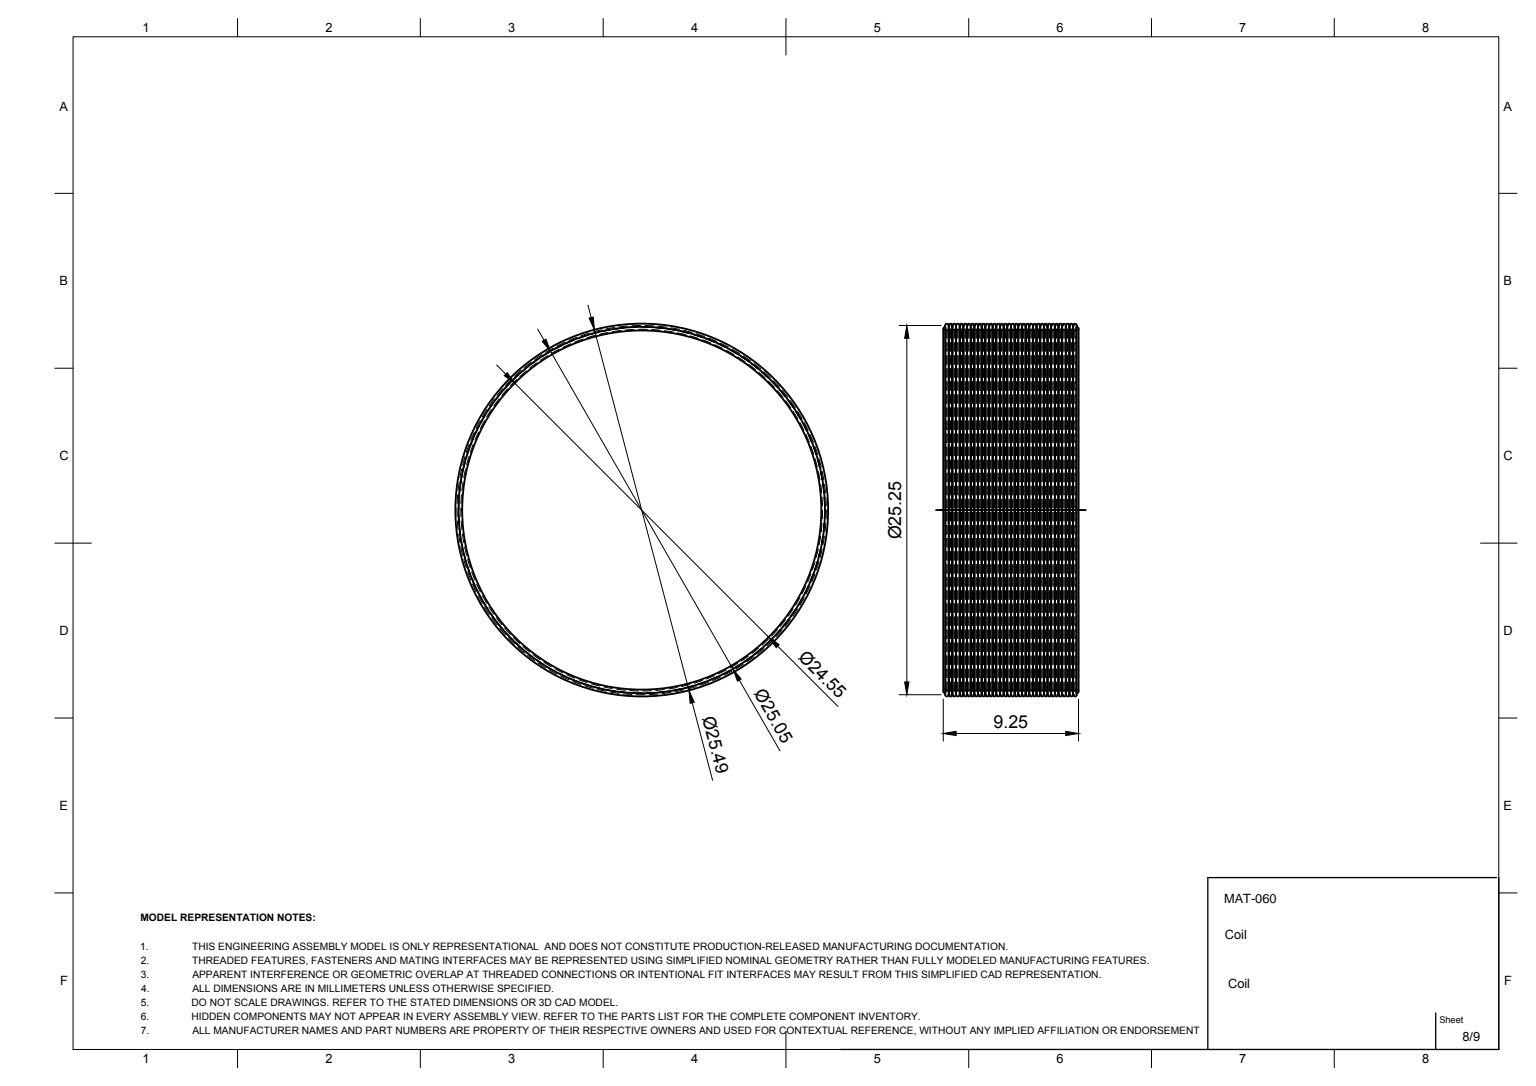
ISO-10303-21;
HEADER;
FILE_DESCRIPTION (('STEP AP214'),
    '1' );
FILE_NAME ('Coil.step',
    '2026-10-29T23:46:56',
    ( '' ),
    ( '' ),
    'SwSTEP 2.0',
    'SolidWorks 2020',
    '' );
FILE_SCHEMA (( 'AUTOMOTIVE_DESIGN' ));
ENDSEC;

DATA;
#4=CIRCLE ( 'NONE', #18333, 0.1250000000000001110 ) ;
#5=EDGE_CURVE ( 'NONE', #10473, #12904, #9508, .T. ) ;
#6=ADVANCED_FACE ( 'NONE', ( #18472 ), #27339, .T. ) ;
#8=ORIENTED_EDGE ( 'NONE', *, *, #21426, .T. ) ;
#12=DIRECTION ( 'NONE',  ( -1.000000000000000000, 0.000000000000000000, 0.000000000000000000 ) ) ;
#21=ORIENTED_EDGE ( 'NONE', *, *, #19854, .F. ) ;
#30=EDGE_CURVE ( 'NONE', #9758, #27591, #28910, .T. ) ;
#31=DIRECTION ( 'NONE',  ( -1.101824276508909887E-16, 1.000000000000000000, -0.000000000000000000 ) ) ;
#32=AXIS2_PLACEMENT_3D ( 'NONE', #27691, #3055, #609 ) ;
#39=VECTOR ( 'NONE', #4275, 1000.000000000000000 ) ;
#43=ORIENTED_EDGE ( 'NONE', *, *, #17117, .T. ) ;
#44=ORIENTED_EDGE ( 'NONE', *, *, #10247, .F. ) ;
#46=DIRECTION ( 'NONE',  ( -1.000000000000000000, 0.000000000000000000, 0.000000000000000000 ) ) ;
#49=EDGE_CURVE ( 'NONE', #29330, #16793, #26511, .T. ) ;
#50=DIRECTION ( 'NONE',  ( -1.000000000000000000, 0.000000000000000000, 0.000000000000000000 ) ) ;
#51=ADVANCED_FACE ( 'NONE', ( #19270 ), #7428, .T. ) ;
#53=DIRECTION ( 'NONE',  ( -1.000000000000000000, 0.000000000000000000, 0.000000000000000000 ) ) ;
#59=AXIS2_PLACEMENT_3D ( 'NONE', #2818, #5773, #10865 ) ;
#63=VERTEX_POINT ( 'NONE', #26669 ) ;
#64=DIRECTION ( 'NONE',  ( -1.101824276508909887E-16, 1.000000000000000000, -0.000000000000000000 ) ) ;
#73=EDGE_LOOP ( 'NONE', ( #31161, #6796, #19023, #7064 ) ) ;
#74=CARTESIAN_POINT ( 'NONE',  ( 21.09992658989238734, 38.56284415653841791, 47.04930799450051637 ) ) ;
#79=DIRECTION ( 'NONE',  ( -1.000000000000000000, 0.000000000000000000, 0.000000000000000000 ) ) ;
#80=DIRECTION ( 'NONE',  ( -1.000000000000000000, -1.101824276508909887E-16, 0.000000000000000000 ) ) ;
#81=EDGE_CURVE ( 'NONE', #21567, #17692, #8244, .T. ) ;
#84=ADVANCED_FACE ( 'NONE', ( #31282 ), #25012, .T. ) ;
#86=ORIENTED_EDGE ( 'NONE', *, *, #14796, .T. ) ;
#89=DIRECTION ( 'NONE',  ( -1.000000000000000000, 0.000000000000000000, 0.000000000000000000 ) ) ;
#92=CARTESIAN_POINT ( 'NONE',  ( 21.09992658989239089, 30.34164230456639544, 47.04930799450051637 ) ) ;
#95=ORIENTED_EDGE ( 'NONE', *, *, #26981, .T. ) ;
#97=ORIENTED_EDGE ( 'NONE', *, *, #2403, .T. ) ;
#102=DIRECTION ( 'NONE',  ( 1.000000000000000000, 0.000000000000000000, 0.000000000000000000 ) ) ;
#104=VERTEX_POINT ( 'NONE', #1886 ) ;
#107=DIRECTION ( 'NONE',  ( 1.000000000000000000, 0.000000000000000000, 0.000000000000000000 ) ) ;
#112=VERTEX_POINT ( 'NONE', #21899 ) ;
#113=CARTESIAN_POINT ( 'NONE',  ( 8.732853799281732776, 24.72145308207319303, 47.04930799450051637 ) ) ;
#116=VERTEX_POINT ( 'NONE', #3866 ) ;
#117=CARTESIAN_POINT ( 'NONE',  ( 8.732853799281729223, 24.47145308207319303, 47.04930799450051637 ) ) ;
#119=DIRECTION ( 'NONE',  ( -1.101824276508909887E-16, 1.000000000000000000, -0.000000000000000000 ) ) ;
#120=CYLINDRICAL_SURFACE ( 'NONE', #5324, 12.36707279061065101 ) ;
#121=FACE_OUTER_BOUND ( 'NONE', #7290, .T. ) ;
#124=TOROIDAL_SURFACE ( 'NONE', #25795, 12.40141737965280555, 0.1250000000000006939 ) ;
#129=ADVANCED_FACE ( 'NONE', ( #26182 ), #24211, .T. ) ;
#130=ADVANCED_FACE ( 'NONE', ( #9112 ), #21404, .F. ) ;
#131=EDGE_LOOP ( 'NONE', ( #2067, #16349, #32197, #29803 ) ) ;
#133=CARTESIAN_POINT ( 'NONE',  ( 33.72499318558949710, 28.84143805560861296, 47.04930799450051637 ) ) ;
#134=ORIENTED_EDGE ( 'NONE', *, *, #4627, .F. ) ;
#135=AXIS2_PLACEMENT_3D ( 'NONE', #30752, #22633, #17877 ) ;
#139=EDGE_LOOP ( 'NONE', ( #10436, #9194, #21125, #26055 ) ) ;
#140=CARTESIAN_POINT ( 'NONE',  ( 21.09992658989239089, 27.84164230456639544, 47.04930799450051637 ) ) ;
#141=ORIENTED_EDGE ( 'NONE', *, *, #21145, .F. ) ;
#142=CIRCLE ( 'NONE', #13264, 12.36707279061065101 ) ;
#146=EDGE_CURVE ( 'NONE', #7136, #25895, #22084, .T. ) ;
#150=FACE_OUTER_BOUND ( 'NONE', #25843, .T. ) ;
#154=VERTEX_POINT ( 'NONE', #31766 ) ;
#157=DIRECTION ( 'NONE',  ( -1.000000000000000000, 0.000000000000000000, 0.000000000000000000 ) ) ;
#172=EDGE_LOOP ( 'NONE', ( #1126, #13141, #16684, #10184 ) ) ;
#173=CARTESIAN_POINT ( 'NONE',  ( 21.09992658989239089, 24.71664230456639899, 47.04930799450051637 ) ) ;
#174=DIRECTION ( 'NONE',  ( -1.101824276508909887E-16, 1.000000000000000000, -0.000000000000000000 ) ) ;
#178=EDGE_CURVE ( 'NONE', #17205, #26283, #21557, .T. ) ;
#181=ORIENTED_EDGE ( 'NONE', *, *, #20445, .T. ) ;
#182=DIRECTION ( 'NONE',  ( -1.000000000000000000, 0.000000000000000000, 0.000000000000000000 ) ) ;
#183=ADVANCED_FACE ( 'NONE', ( #22228 ), #31147, .T. ) ;
#190=CARTESIAN_POINT ( 'NONE',  ( 21.09992658989238734, 38.56284415653841791, 47.04930799450051637 ) ) ;
#191=CARTESIAN_POINT ( 'NONE',  ( 8.698509210239514289, 24.84164230456639544, 47.04930799450051637 ) ) ;
#193=DIRECTION ( 'NONE',  ( -1.000000000000000000, 0.000000000000000000, 0.000000000000000000 ) ) ;
#200=DIRECTION ( 'NONE',  ( -1.000000000000000000, 0.000000000000000000, 0.000000000000000000 ) ) ;
#204=CARTESIAN_POINT ( 'NONE',  ( 33.46699938050303302, 38.56284415653841791, 47.04930799450051637 ) ) ;
#213=ORIENTED_EDGE ( 'NONE', *, *, #21228, .T. ) ;
#215=CARTESIAN_POINT ( 'NONE',  ( 8.732853799281732776, 31.97145308207317171, 47.04930799450051637 ) ) ;
#217=DIRECTION ( 'NONE',  ( -1.000000000000000000, 0.000000000000000000, 0.000000000000000000 ) ) ;
#219=CARTESIAN_POINT ( 'NONE',  ( 8.823509210239564027, 29.84164230456639899, 47.04930799450051637 ) ) ;
#220=ADVANCED_FACE ( 'NONE', ( #24531 ), #2050, .F. ) ;
#221=EDGE_CURVE ( 'NONE', #14341, #26283, #20036, .T. ) ;
#222=EDGE_LOOP ( 'NONE', ( #26928, #11446, #19601, #18830 ) ) ;
#223=DIRECTION ( 'NONE',  ( -1.000000000000000000, 0.000000000000000000, 0.000000000000000000 ) ) ;
#228=DIRECTION ( 'NONE',  ( -1.101824276508909887E-16, 1.000000000000000000, -0.000000000000000000 ) ) ;
#230=CARTESIAN_POINT ( 'NONE',  ( 21.09992658989238734, 31.96183152705962272, 47.04930799450051637 ) ) ;
#231=VERTEX_POINT ( 'NONE', #9774 ) ;
#236=AXIS2_PLACEMENT_3D ( 'NONE', #25222, #28009, #15050 ) ;
#237=DIRECTION ( 'NONE',  ( -1.101824276508909887E-16, 1.000000000000000000, -0.000000000000000000 ) ) ;
#246=ORIENTED_EDGE ( 'NONE', *, *, #15564, .T. ) ;
#248=DIRECTION ( 'NONE',  ( 0.000000000000000000, -0.000000000000000000, -1.000000000000000000 ) ) ;
#254=DIRECTION ( 'NONE',  ( -1.101824276508909887E-16, 1.000000000000000000, -0.000000000000000000 ) ) ;
#256=EDGE_CURVE ( 'NONE', #10661, #20619, #16974, .T. ) ;
#262=EDGE_CURVE ( 'NONE', #32275, #3483, #1780, .T. ) ;
#264=CARTESIAN_POINT ( 'NONE',  ( 8.732853799281732776, 30.71183152705961916, 47.04930799450051637 ) ) ;
#266=ORIENTED_EDGE ( 'NONE', *, *, #15415, .T. ) ;
#267=ORIENTED_EDGE ( 'NONE', *, *, #8560, .T. ) ;
#270=LINE ( 'NONE', #3046, #13238 ) ;
#272=VERTEX_POINT ( 'NONE', #8893 ) ;
#281=DIRECTION ( 'NONE',  ( -1.101824276508909887E-16, 1.000000000000000000, -0.000000000000000000 ) ) ;
#287=CARTESIAN_POINT ( 'NONE',  ( 21.09992658989239089, 24.84164230456639544, 47.04930799450051637 ) ) ;
#291=AXIS2_PLACEMENT_3D ( 'NONE', #31241, #28293, #23031 ) ;
#293=ORIENTED_EDGE ( 'NONE', *, *, #30810, .T. ) ;
#295=DIRECTION ( 'NONE',  ( -1.101824276508909887E-16, 1.000000000000000000, -0.000000000000000000 ) ) ;
#299=ADVANCED_FACE ( 'NONE', ( #6919 ), #23984, .F. ) ;
#303=EDGE_CURVE ( 'NONE', #15685, #10922, #5506, .T. ) ;
#305=CIRCLE ( 'NONE', #9213, 12.27641737965284996 ) ;
#312=CARTESIAN_POINT ( 'NONE',  ( 21.09992658989239089, 28.46183152705961206, 47.04930799450051637 ) ) ;
#314=TOROIDAL_SURFACE ( 'NONE', #1339, 12.61792373059896377, 0.1249999999999977518 ) ;
#321=VERTEX_POINT ( 'NONE', #31552 ) ;
#326=ORIENTED_EDGE ( 'NONE', *, *, #9341, .F. ) ;
#327=CARTESIAN_POINT ( 'NONE',  ( 33.72499318558949710, 27.84184655352419568, 47.04930799450051637 ) ) ;
#330=CIRCLE ( 'NONE', #8187, 12.27641737965285529 ) ;
#331=( GEOMETRIC_REPRESENTATION_CONTEXT ( 3 ) GLOBAL_UNCERTAINTY_ASSIGNED_CONTEXT ( ( #30822 ) ) GLOBAL_UNIT_ASSIGNED_CONTEXT ( ( #10061, #30087, #12694 ) ) REPRESENTATION_CONTEXT ( 'NONE', 'WORKASPACE' ) );
#333=ORIENTED_EDGE ( 'NONE', *, *, #7951, .F. ) ;
#334=ADVANCED_FACE ( 'NONE', ( #16752 ), #23450, .T. ) ;
#335=EDGE_CURVE ( 'NONE', #25296, #11753, #1955, .T. ) ;
#338=DIRECTION ( 'NONE',  ( -1.101824276508909887E-16, 1.000000000000000000, -0.000000000000000000 ) ) ;
#340=DIRECTION ( 'NONE',  ( -1.101824276508909887E-16, 1.000000000000000000, -0.000000000000000000 ) ) ;
#341=ORIENTED_EDGE ( 'NONE', *, *, #19982, .F. ) ;
#346=CARTESIAN_POINT ( 'NONE',  ( 8.698509210239533829, 26.84164230456639899, 47.04930799450051637 ) ) ;
#349=CARTESIAN_POINT ( 'NONE',  ( 21.09992658989239089, 28.46183152705961206, 47.04930799450051637 ) ) ;
#351=DIRECTION ( 'NONE',  ( 1.000000000000000000, 0.000000000000000000, 0.000000000000000000 ) ) ;
#352=DIRECTION ( 'NONE',  ( -1.000000000000000000, 0.000000000000000000, 0.000000000000000000 ) ) ;
#358=DIRECTION ( 'NONE',  ( -1.101824276508909887E-16, 1.000000000000000000, -0.000000000000000000 ) ) ;
#360=AXIS2_PLACEMENT_3D ( 'NONE', #25134, #12675, #32035 ) ;
#362=ORIENTED_EDGE ( 'NONE', *, *, #4106, .T. ) ;
#363=CARTESIAN_POINT ( 'NONE',  ( 8.732853799281732776, 31.21183152705961206, 47.04930799450051637 ) ) ;
#368=DIRECTION ( 'NONE',  ( -1.101824276508909887E-16, 1.000000000000000000, -0.000000000000000000 ) ) ;
#371=EDGE_CURVE ( 'NONE', #32203, #7136, #10883, .T. ) ;
#373=DIRECTION ( 'NONE',  ( -1.101824276508909887E-16, 1.000000000000000000, -0.000000000000000000 ) ) ;
#375=AXIS2_PLACEMENT_3D ( 'NONE', #26320, #1199, #3831 ) ;
#377=ADVANCED_FACE ( 'NONE', ( #14478 ), #21344, .F. ) ;
#381=LINE ( 'NONE', #32408, #22412 ) ;
#387=EDGE_CURVE ( 'NONE', #272, #6908, #900, .T. ) ;
#392=AXIS2_PLACEMENT_3D ( 'NONE', #10385, #24997, #12533 ) ;
#397=DIRECTION ( 'NONE',  ( -0.5849755626391566210, -0.8110509177080080789, 7.163884503654653530E-17 ) ) ;
#401=DIRECTION ( 'NONE',  ( -1.000000000000000000, -1.101824276508909764E-16, 0.000000000000000000 ) ) ;
#403=ORIENTED_EDGE ( 'NONE', *, *, #28119, .T. ) ;
#404=DIRECTION ( 'NONE',  ( -1.101824276508909887E-16, 1.000000000000000000, -0.000000000000000000 ) ) ;
#405=DIRECTION ( 'NONE',  ( -1.000000000000000000, 0.000000000000000000, 0.000000000000000000 ) ) ;
#406=ADVANCED_FACE ( 'NONE', ( #1831 ), #16107, .T. ) ;
#409=AXIS2_PLACEMENT_3D ( 'NONE', #26501, #24355, #11732 ) ;
#410=DIRECTION ( 'NONE',  ( -1.000000000000000000, 0.000000000000000000, 0.000000000000000000 ) ) ;
#412=ORIENTED_EDGE ( 'NONE', *, *, #4110, .T. ) ;
#414=VERTEX_POINT ( 'NONE', #16673 ) ;
#420=TOROIDAL_SURFACE ( 'NONE', #8282, 12.61792373059898154, 0.1249999999999967248 ) ;
#429=EDGE_CURVE ( 'NONE', #5692, #16617, #5104, .T. ) ;
#430=CARTESIAN_POINT ( 'NONE',  ( 33.50134396954523197, 28.09164230456639544, 47.04930799450051637 ) ) ;
#434=DIRECTION ( 'NONE',  ( -1.101824276508909887E-16, 1.000000000000000000, -0.000000000000000000 ) ) ;
#435=EDGE_LOOP ( 'NONE', ( #10154, #19210, #8973, #1783 ) ) ;
#442=DIRECTION ( 'NONE',  ( -1.101824276508909887E-16, 1.000000000000000000, -0.000000000000000000 ) ) ;
#443=DIRECTION ( 'NONE',  ( -1.000000000000000000, 0.000000000000000000, 0.000000000000000000 ) ) ;
#444=ORIENTED_EDGE ( 'NONE', *, *, #23203, .F. ) ;
#445=CARTESIAN_POINT ( 'NONE',  ( 21.09992658989239089, 28.09164230456639544, 47.04930799450051637 ) ) ;
#449=ADVANCED_FACE ( 'NONE', ( #28848 ), #6361, .F. ) ;
#450=AXIS2_PLACEMENT_3D ( 'NONE', #12001, #14627, #24141 ) ;
#457=DIRECTION ( 'NONE',  ( -1.101824276508909887E-16, 1.000000000000000000, -0.000000000000000000 ) ) ;
#460=VERTEX_POINT ( 'NONE', #16358 ) ;
#464=EDGE_LOOP ( 'NONE', ( #6672, #7321, #19519, #30159 ) ) ;
#465=AXIS2_PLACEMENT_3D ( 'NONE', #20669, #30697, #8207 ) ;
#473=EDGE_LOOP ( 'NONE', ( #24500, #19436, #2603, #32349 ) ) ;
#474=AXIS2_PLACEMENT_3D ( 'NONE', #27244, #4772, #14789 ) ;
#477=CARTESIAN_POINT ( 'NONE',  ( 21.09992658989239089, 25.72145308207319303, 47.04930799450051637 ) ) ;
#478=LINE ( 'NONE', #7396, #21500 ) ;
#481=DIRECTION ( 'NONE',  ( -1.101824276508909887E-16, 1.000000000000000000, -0.000000000000000000 ) ) ;
#488=AXIS2_PLACEMENT_3D ( 'NONE', #13721, #10934, #17987 ) ;
#498=CARTESIAN_POINT ( 'NONE',  ( 33.46699938050303302, 38.56284415653841791, 47.04930799450051637 ) ) ;
#505=AXIS2_PLACEMENT_3D ( 'NONE', #21570, #21893, #31922 ) ;
#511=DIRECTION ( 'NONE',  ( -1.101824276508909887E-16, 1.000000000000000000, -0.000000000000000000 ) ) ;
#515=DIRECTION ( 'NONE',  ( -1.224646799147353207E-16, -1.349345573449484691E-32, 1.000000000000000000 ) ) ;
#517=CIRCLE ( 'NONE', #11031, 0.1249999999999966416 ) ;
#518=CIRCLE ( 'NONE', #27799, 12.62506659569710266 ) ;
#519=EDGE_CURVE ( 'NONE', #12816, #17665, #21603, .T. ) ;
#520=DIRECTION ( 'NONE',  ( -1.101824276508909887E-16, 1.000000000000000000, -0.000000000000000000 ) ) ;
#521=EDGE_CURVE ( 'NONE', #13589, #18578, #21569, .T. ) ;
#523=ORIENTED_EDGE ( 'NONE', *, *, #9183, .T. ) ;
#528=ORIENTED_EDGE ( 'NONE', *, *, #976, .F. ) ;
#531=EDGE_CURVE ( 'NONE', #4270, #19118, #14239, .T. ) ;
#537=VECTOR ( 'NONE', #21856, 1000.000000000000000 ) ;
#540=CARTESIAN_POINT ( 'NONE',  ( 33.46699938050303302, 30.47145308207317882, 47.04930799450050927 ) ) ;
#542=CIRCLE ( 'NONE', #23088, 12.27641737965281266 ) ;
#543=ORIENTED_EDGE ( 'NONE', *, *, #8534, .F. ) ;
#544=CIRCLE ( 'NONE', #9998, 12.36707279061065101 ) ;
#552=ORIENTED_EDGE ( 'NONE', *, *, #8175, .T. ) ;
#554=FACE_OUTER_BOUND ( 'NONE', #4438, .T. ) ;
#555=DIRECTION ( 'NONE',  ( -1.101824276508909887E-16, 1.000000000000000000, -0.000000000000000000 ) ) ;
#556=DIRECTION ( 'NONE',  ( -1.101824276508909887E-16, 1.000000000000000000, -0.000000000000000000 ) ) ;
#562=CARTESIAN_POINT ( 'NONE',  ( 21.09992658989239089, 25.09143805560860940, 47.04930799450051637 ) ) ;
#568=EDGE_LOOP ( 'NONE', ( #14512, #13383, #25114, #14670 ) ) ;
#570=ADVANCED_FACE ( 'NONE', ( #26865 ), #5884, .T. ) ;
#573=CIRCLE ( 'NONE', #3187, 12.36707279061065101 ) ;
#574=CARTESIAN_POINT ( 'NONE',  ( 21.09992658989238734, 32.59164230456639899, 47.04930799450051637 ) ) ;
#575=ORIENTED_EDGE ( 'NONE', *, *, #29988, .T. ) ;
#576=CARTESIAN_POINT ( 'NONE',  ( 8.823509210239508960, 24.34164230456639544, 47.04930799450051637 ) ) ;
#578=CIRCLE ( 'NONE', #23109, 12.62506659569710266 ) ;
#579=EDGE_LOOP ( 'NONE', ( #28790, #1429, #13483, #28688 ) ) ;
#580=CIRCLE ( 'NONE', #21523, 12.27641737965287660 ) ;
#582=ORIENTED_EDGE ( 'NONE', *, *, #11719, .F. ) ;
#583=EDGE_CURVE ( 'NONE', #20144, #2267, #11926, .T. ) ;
#590=EDGE_CURVE ( 'NONE', #21064, #20430, #26831, .T. ) ;
#593=VERTEX_POINT ( 'NONE', #10739 ) ;
#597=FACE_OUTER_BOUND ( 'NONE', #26506, .T. ) ;
#599=DIRECTION ( 'NONE',  ( -1.101824276508909887E-16, 1.000000000000000000, -0.000000000000000000 ) ) ;
#602=CARTESIAN_POINT ( 'NONE',  ( 21.09992658989238734, 32.34143805560860585, 47.04930799450051637 ) ) ;
#609=DIRECTION ( 'NONE',  ( -1.000000000000000000, 0.000000000000000000, 0.000000000000000000 ) ) ;
#611=CARTESIAN_POINT ( 'NONE',  ( 21.09992658989238734, 31.34164230456639544, 47.04930799450051637 ) ) ;
#618=DIRECTION ( 'NONE',  ( 0.000000000000000000, -0.000000000000000000, -1.000000000000000000 ) ) ;
#623=ORIENTED_EDGE ( 'NONE', *, *, #14827, .F. ) ;
#625=ADVANCED_FACE ( 'NONE', ( #9634 ), #30756, .F. ) ;
#628=DIRECTION ( 'NONE',  ( -1.101824276508909887E-16, 1.000000000000000000, -0.000000000000000000 ) ) ;
#630=ADVANCED_FACE ( 'NONE', ( #2411 ), #30939, .T. ) ;
#633=AXIS2_PLACEMENT_3D ( 'NONE', #24321, #29422, #19555 ) ;
#635=CARTESIAN_POINT ( 'NONE',  ( 33.50134396954526750, 24.84164230456639544, 47.04930799450051637 ) ) ;
#641=ORIENTED_EDGE ( 'NONE', *, *, #13247, .T. ) ;
#642=CIRCLE ( 'NONE', #30013, 12.36707279061065101 ) ;
#643=DIRECTION ( 'NONE',  ( 1.000000000000000000, 0.000000000000000000, 0.000000000000000000 ) ) ;
#645=DIRECTION ( 'NONE',  ( -1.000000000000000000, -1.101824276508910010E-16, 0.000000000000000000 ) ) ;
#648=DIRECTION ( 'NONE',  ( 1.101824276508909887E-16, -1.000000000000000000, 0.000000000000000000 ) ) ;
#650=DIRECTION ( 'NONE',  ( 1.000000000000000000, 0.000000000000000000, 0.000000000000000000 ) ) ;
#657=CARTESIAN_POINT ( 'NONE',  ( 21.09992658989238734, 38.56284415653841791, 47.04930799450051637 ) ) ;
#658=DIRECTION ( 'NONE',  ( 0.000000000000000000, -0.000000000000000000, -1.000000000000000000 ) ) ;
#661=AXIS2_PLACEMENT_3D ( 'NONE', #13637, #15449, #25779 ) ;
#662=AXIS2_PLACEMENT_3D ( 'NONE', #7675, #4884, #7833 ) ;
#667=DIRECTION ( 'NONE',  ( -1.101824276508909887E-16, 1.000000000000000000, -0.000000000000000000 ) ) ;
#671=EDGE_CURVE ( 'NONE', #28587, #29229, #2630, .T. ) ;
#672=ADVANCED_FACE ( 'NONE', ( #28602 ), #22535, .T. ) ;
#679=DIRECTION ( 'NONE',  ( -1.101824276508909887E-16, 1.000000000000000000, -0.000000000000000000 ) ) ;
#680=CARTESIAN_POINT ( 'NONE',  ( 33.62634396954528171, 23.59164230456639544, 47.04930799450050927 ) ) ;
#682=CIRCLE ( 'NONE', #19008, 12.62506659569710266 ) ;
#687=ORIENTED_EDGE ( 'NONE', *, *, #2527, .F. ) ;
#689=FACE_OUTER_BOUND ( 'NONE', #3946, .T. ) ;
#693=DIRECTION ( 'NONE',  ( -1.224646799147353207E-16, -1.349345573449484691E-32, 1.000000000000000000 ) ) ;
#694=CARTESIAN_POINT ( 'NONE',  ( 8.823509210239512512, 24.59164230456639544, 47.04930799450051637 ) ) ;
#695=EDGE_LOOP ( 'NONE', ( #23280, #30142, #10297, #134 ) ) ;
#696=EDGE_LOOP ( 'NONE', ( #17955, #23554, #928, #3207 ) ) ;
#702=TOROIDAL_SURFACE ( 'NONE', #15402, 12.40141737965284108, 0.1249999999999997918 ) ;
#703=VECTOR ( 'NONE', #2894, 1000.000000000000000 ) ;
#704=DIRECTION ( 'NONE',  ( -1.000000000000000000, 0.000000000000000000, 0.000000000000000000 ) ) ;
#705=APPLICATION_CONTEXT ( 'automotive_design' ) ;
#708=ORIENTED_EDGE ( 'NONE', *, *, #2194, .T. ) ;
#711=EDGE_CURVE ( 'NONE', #20645, #17250, #26734, .T. ) ;
#713=AXIS2_PLACEMENT_3D ( 'NONE', #13100, #30498, #10310 ) ;
#714=EDGE_CURVE ( 'NONE', #24189, #27727, #5769, .T. ) ;
#717=ADVANCED_FACE ( 'NONE', ( #868 ), #14154, .T. ) ;
#729=DIRECTION ( 'NONE',  ( -1.000000000000000000, 0.000000000000000000, 0.000000000000000000 ) ) ;
#735=ORIENTED_EDGE ( 'NONE', *, *, #14856, .T. ) ;
#736=CARTESIAN_POINT ( 'NONE',  ( 21.09992658989239089, 26.59184655352419568, 47.04930799450051637 ) ) ;
#740=VECTOR ( 'NONE', #4684, 1000.000000000000000 ) ;
#741=ORIENTED_EDGE ( 'NONE', *, *, #31620, .T. ) ;
#744=EDGE_CURVE ( 'NONE', #30931, #20832, #4, .T. ) ;
#748=DIRECTION ( 'NONE',  ( -1.101824276508909887E-16, 1.000000000000000000, -0.000000000000000000 ) ) ;
#749=CARTESIAN_POINT ( 'NONE',  ( 33.46699938050304013, 25.21183152705960140, 47.04930799450051637 ) ) ;
#750=CIRCLE ( 'NONE', #26968, 0.1250000000000001110 ) ;
#757=CIRCLE ( 'NONE', #4954, 0.1250000000000001110 ) ;
#763=DIRECTION ( 'NONE',  ( -1.101824276508909887E-16, 1.000000000000000000, -0.000000000000000000 ) ) ;
#766=CARTESIAN_POINT ( 'NONE',  ( 21.09992658989238734, 38.56284415653841791, 47.04930799450051637 ) ) ;
#767=ORIENTED_EDGE ( 'NONE', *, *, #12081, .F. ) ;
#770=DIRECTION ( 'NONE',  ( -1.000000000000000000, -1.101824276508909887E-16, 0.000000000000000000 ) ) ;
#778=AXIS2_PLACEMENT_3D ( 'NONE', #28726, #16083, #11486 ) ;
#781=AXIS2_PLACEMENT_3D ( 'NONE', #5119, #12351, #22344 ) ;
#785=CIRCLE ( 'NONE', #19101, 12.62506659569710266 ) ;
#788=CARTESIAN_POINT ( 'NONE',  ( 8.732853799281738105, 29.21183152705961206, 47.04930799450051637 ) ) ;
#790=EDGE_LOOP ( 'NONE', ( #28035, #4033, #21933, #28843 ) ) ;
#792=CARTESIAN_POINT ( 'NONE',  ( 21.09992658989238734, 30.96183152705961206, 47.04930799450051637 ) ) ;
#797=ORIENTED_EDGE ( 'NONE', *, *, #29579, .T. ) ;
#798=ORIENTED_EDGE ( 'NONE', *, *, #992, .F. ) ;
#800=CARTESIAN_POINT ( 'NONE',  ( 21.09992658989239089, 28.34164230456639544, 47.04930799450051637 ) ) ;
#807=CARTESIAN_POINT ( 'NONE',  ( 33.46699938050304013, 27.47145308207318593, 47.04930799450050927 ) ) ;
#810=ORIENTED_EDGE ( 'NONE', *, *, #8618, .F. ) ;
#812=CARTESIAN_POINT ( 'NONE',  ( 21.09992658989238734, 31.09164230456639544, 47.04930799450051637 ) ) ;
#835=ORIENTED_EDGE ( 'NONE', *, *, #12736, .T. ) ;
#844=ORIENTED_EDGE ( 'NONE', *, *, #2452, .T. ) ;
#850=ORIENTED_EDGE ( 'NONE', *, *, #29495, .F. ) ;
#853=ORIENTED_EDGE ( 'NONE', *, *, #19976, .F. ) ;
#858=CIRCLE ( 'NONE', #22872, 12.62506659569710266 ) ;
#860=EDGE_CURVE ( 'NONE', #13790, #27623, #578, .T. ) ;
#863=CIRCLE ( 'NONE', #13468, 0.1250000000000001110 ) ;
#865=ORIENTED_EDGE ( 'NONE', *, *, #20443, .F. ) ;
#867=FACE_OUTER_BOUND ( 'NONE', #19263, .T. ) ;
#868=FACE_OUTER_BOUND ( 'NONE', #17054, .T. ) ;
#869=AXIS2_PLACEMENT_3D ( 'NONE', #29737, #14966, #29905 ) ;
#881=ORIENTED_EDGE ( 'NONE', *, *, #31352, .F. ) ;
#888=CIRCLE ( 'NONE', #30776, 12.27641737965288726 ) ;
#889=DIRECTION ( 'NONE',  ( -1.000000000000000000, 0.000000000000000000, 0.000000000000000000 ) ) ;
#893=VERTEX_POINT ( 'NONE', #12685 ) ;
#894=EDGE_CURVE ( 'NONE', #7034, #9970, #12106, .T. ) ;
#900=CIRCLE ( 'NONE', #31833, 12.62506659569710266 ) ;
#903=CARTESIAN_POINT ( 'NONE',  ( 8.573509210239501854, 23.59164230456639544, 47.04930799450051637 ) ) ;
#905=ORIENTED_EDGE ( 'NONE', *, *, #16478, .F. ) ;
#906=LINE ( 'NONE', #10621, #25046 ) ;
#910=DIRECTION ( 'NONE',  ( -1.000000000000000000, -1.101824276508909764E-16, 0.000000000000000000 ) ) ;
#913=EDGE_CURVE ( 'NONE', #25724, #15900, #27600, .T. ) ;
#914=ORIENTED_EDGE ( 'NONE', *, *, #23784, .T. ) ;
#917=CARTESIAN_POINT ( 'NONE',  ( 33.50134396954528171, 23.84164230456639544, 47.04930799450051637 ) ) ;
#918=DIRECTION ( 'NONE',  ( -1.000000000000000000, 0.000000000000000000, 0.000000000000000000 ) ) ;
#922=CARTESIAN_POINT ( 'NONE',  ( 21.09992658989239089, 28.46664230456639899, 47.04930799450051637 ) ) ;
#924=CARTESIAN_POINT ( 'NONE',  ( 33.37634396954526750, 25.09164230456639899, 47.04930799450051637 ) ) ;
#926=DIRECTION ( 'NONE',  ( -1.101824276508909887E-16, 1.000000000000000000, -0.000000000000000000 ) ) ;
#928=ORIENTED_EDGE ( 'NONE', *, *, #23814, .T. ) ;
#929=CARTESIAN_POINT ( 'NONE',  ( 33.46699938050304013, 28.72145308207318237, 47.04930799450050927 ) ) ;
#934=ORIENTED_EDGE ( 'NONE', *, *, #16622, .F. ) ;
#940=ORIENTED_EDGE ( 'NONE', *, *, #29043, .F. ) ;
#941=CIRCLE ( 'NONE', #31356, 12.62506659569710266 ) ;
#942=AXIS2_PLACEMENT_3D ( 'NONE', #17620, #12882, #24854 ) ;
#947=DIRECTION ( 'NONE',  ( -1.101824276508909887E-16, 1.000000000000000000, -0.000000000000000000 ) ) ;
#950=ADVANCED_FACE ( 'NONE', ( #2490 ), #25622, .F. ) ;
#951=ORIENTED_EDGE ( 'NONE', *, *, #18687, .F. ) ;
#955=EDGE_CURVE ( 'NONE', #13402, #21770, #9293, .T. ) ;
#963=AXIS2_PLACEMENT_3D ( 'NONE', #7486, #14707, #4524 ) ;
#965=CARTESIAN_POINT ( 'NONE',  ( 33.50134396954524618, 26.59164230456639899, 47.04930799450051637 ) ) ;
#968=CARTESIAN_POINT ( 'NONE',  ( 21.09992658989239089, 26.59164230456639899, 47.04930799450051637 ) ) ;
#976=EDGE_CURVE ( 'NONE', #27344, #24538, #26061, .T. ) ;
#979=VECTOR ( 'NONE', #254, 1000.000000000000000 ) ;
#984=CARTESIAN_POINT ( 'NONE',  ( 21.09992658989239089, 25.34184655352419213, 47.04930799450051637 ) ) ;
#987=AXIS2_PLACEMENT_3D ( 'NONE', #4935, #14949, #9537 ) ;
#992=EDGE_CURVE ( 'NONE', #10697, #9081, #30273, .T. ) ;
#995=ADVANCED_FACE ( 'NONE', ( #18386 ), #31829, .T. ) ;
#997=DIRECTION ( 'NONE',  ( -1.101824276508909887E-16, 1.000000000000000000, -0.000000000000000000 ) ) ;
#1000=DIRECTION ( 'NONE',  ( -1.101824276508909887E-16, 1.000000000000000000, -0.000000000000000000 ) ) ;
#1001=CARTESIAN_POINT ( 'NONE',  ( 8.732853799281734553, 38.56284415653841791, 47.04930799450051637 ) ) ;
#1002=FACE_OUTER_BOUND ( 'NONE', #23225, .T. ) ;
#1003=ORIENTED_EDGE ( 'NONE', *, *, #7201, .T. ) ;
#1004=ORIENTED_EDGE ( 'NONE', *, *, #5227, .F. ) ;
#1006=TOROIDAL_SURFACE ( 'NONE', #23517, 12.40141737965281088, 0.1249999999999987788 ) ;
#1019=AXIS2_PLACEMENT_3D ( 'NONE', #16547, #14431, #19660 ) ;
#1020=ORIENTED_EDGE ( 'NONE', *, *, #10985, .T. ) ;
#1024=TOROIDAL_SURFACE ( 'NONE', #17777, 12.61792373059896732, 0.1249999999999974604 ) ;
#1027=VERTEX_POINT ( 'NONE', #26268 ) ;
#1030=DIRECTION ( 'NONE',  ( -1.000000000000000000, 0.000000000000000000, 0.000000000000000000 ) ) ;
#1031=EDGE_CURVE ( 'NONE', #23957, #25242, #18699, .T. ) ;
#1032=AXIS2_PLACEMENT_3D ( 'NONE', #27247, #9702, #19534 ) ;
#1033=ORIENTED_EDGE ( 'NONE', *, *, #20379, .T. ) ;
#1034=VECTOR ( 'NONE', #9749, 1000.000000000000000 ) ;
#1035=DIRECTION ( 'NONE',  ( -1.101824276508909887E-16, 1.000000000000000000, -0.000000000000000000 ) ) ;
#1037=DIRECTION ( 'NONE',  ( -1.101824276508909887E-16, 1.000000000000000000, -0.000000000000000000 ) ) ;
#1039=AXIS2_PLACEMENT_3D ( 'NONE', #6070, #23305, #5912 ) ;
#1044=DIRECTION ( 'NONE',  ( 1.000000000000000000, 0.000000000000000000, 0.000000000000000000 ) ) ;
#1054=DIRECTION ( 'NONE',  ( -1.101824276508909887E-16, 1.000000000000000000, -0.000000000000000000 ) ) ;
#1055=TOROIDAL_SURFACE ( 'NONE', #17283, 12.40141737965287838, 0.1249999999999998335 ) ;
#1058=ORIENTED_EDGE ( 'NONE', *, *, #4110, .F. ) ;
#1061=CIRCLE ( 'NONE', #21472, 0.1250000000000001110 ) ;
#1062=ORIENTED_EDGE ( 'NONE', *, *, #8099, .F. ) ;
#1064=VECTOR ( 'NONE', #6334, 1000.000000000000000 ) ;
#1068=DIRECTION ( 'NONE',  ( -1.000000000000000000, 0.000000000000000000, 0.000000000000000000 ) ) ;
#1073=VERTEX_POINT ( 'NONE', #6245 ) ;
#1075=FACE_OUTER_BOUND ( 'NONE', #20162, .T. ) ;
#1076=DIRECTION ( 'NONE',  ( -1.101824276508909887E-16, 1.000000000000000000, -0.000000000000000000 ) ) ;
#1084=DIRECTION ( 'NONE',  ( -1.224646799147353207E-16, -1.349345573449484691E-32, 1.000000000000000000 ) ) ;
#1100=ORIENTED_EDGE ( 'NONE', *, *, #7352, .F. ) ;
#1107=ADVANCED_FACE ( 'NONE', ( #13328 ), #31202, .T. ) ;
#1108=EDGE_CURVE ( 'NONE', #22169, #9593, #15435, .T. ) ;
#1112=CARTESIAN_POINT ( 'NONE',  ( 21.09992658989239089, 25.84164230456639899, 47.04930799450051637 ) ) ;
#1114=EDGE_CURVE ( 'NONE', #116, #23509, #31166, .T. ) ;
#1121=VERTEX_POINT ( 'NONE', #10860 ) ;
#1126=ORIENTED_EDGE ( 'NONE', *, *, #29812, .T. ) ;
#1127=DIRECTION ( 'NONE',  ( -1.101824276508909887E-16, 1.000000000000000000, -0.000000000000000000 ) ) ;
#1128=AXIS2_PLACEMENT_3D ( 'NONE', #27328, #4847, #17796 ) ;
#1129=FACE_OUTER_BOUND ( 'NONE', #695, .T. ) ;
#1133=ORIENTED_EDGE ( 'NONE', *, *, #146, .T. ) ;
#1134=DIRECTION ( 'NONE',  ( -1.101824276508909887E-16, 1.000000000000000000, -0.000000000000000000 ) ) ;
#1136=CARTESIAN_POINT ( 'NONE',  ( 33.46699938050303302, 38.56284415653841791, 47.04930799450051637 ) ) ;
#1140=VERTEX_POINT ( 'NONE', #29378 ) ;
#1143=CARTESIAN_POINT ( 'NONE',  ( 33.50134396954523908, 27.09164230456639899, 47.04930799450051637 ) ) ;
#1144=ORIENTED_EDGE ( 'NONE', *, *, #5166, .F. ) ;
#1148=CARTESIAN_POINT ( 'NONE',  ( 21.09992658989239089, 26.59143805560860940, 47.04930799450051637 ) ) ;
#1153=DIRECTION ( 'NONE',  ( -1.101824276508909887E-16, 1.000000000000000000, -0.000000000000000000 ) ) ;
#1154=DIRECTION ( 'NONE',  ( -1.000000000000000000, 0.000000000000000000, 0.000000000000000000 ) ) ;
#1161=FACE_OUTER_BOUND ( 'NONE', #5845, .T. ) ;
#1162=TOROIDAL_SURFACE ( 'NONE', #11675, 12.40141737965283042, 0.1249999999999995420 ) ;
#1164=LINE ( 'NONE', #18085, #25026 ) ;
#1171=ADVANCED_FACE ( 'NONE', ( #12149 ), #27233, .F. ) ;
#1177=DIRECTION ( 'NONE',  ( -1.101824276508909887E-16, 1.000000000000000000, -0.000000000000000000 ) ) ;
#1183=AXIS2_PLACEMENT_3D ( 'NONE', #22137, #14606, #32166 ) ;
#1186=DIRECTION ( 'NONE',  ( -1.000000000000000000, 0.000000000000000000, 0.000000000000000000 ) ) ;
#1190=CARTESIAN_POINT ( 'NONE',  ( 21.09992658989238734, 31.34184655352422766, 47.04930799450051637 ) ) ;
#1199=DIRECTION ( 'NONE',  ( 0.000000000000000000, -0.000000000000000000, -1.000000000000000000 ) ) ;
#1205=DIRECTION ( 'NONE',  ( 1.000000000000000000, 0.000000000000000000, 0.000000000000000000 ) ) ;
#1207=EDGE_CURVE ( 'NONE', #14676, #24757, #29053, .T. ) ;
#1209=TOROIDAL_SURFACE ( 'NONE', #13804, 12.61792373059897621, 0.1249999999999970163 ) ;
#1214=EDGE_CURVE ( 'NONE', #30342, #31925, #15331, .T. ) ;
#1221=DIRECTION ( 'NONE',  ( -1.101824276508909887E-16, 1.000000000000000000, -0.000000000000000000 ) ) ;
#1228=DIRECTION ( 'NONE',  ( -1.000000000000000000, 0.000000000000000000, 0.000000000000000000 ) ) ;
#1229=VERTEX_POINT ( 'NONE', #17703 ) ;
#1232=DIRECTION ( 'NONE',  ( 1.000000000000000000, 0.000000000000000000, 0.000000000000000000 ) ) ;
#1233=DIRECTION ( 'NONE',  ( -1.000000000000000000, 0.000000000000000000, 0.000000000000000000 ) ) ;
#1241=AXIS2_PLACEMENT_3D ( 'NONE', #4451, #6592, #13985 ) ;
#1247=DIRECTION ( 'NONE',  ( -1.101824276508909887E-16, 1.000000000000000000, -0.000000000000000000 ) ) ;
#1249=ORIENTED_EDGE ( 'NONE', *, *, #26072, .T. ) ;
#1250=ORIENTED_EDGE ( 'NONE', *, *, #9597, .F. ) ;
#1253=ADVANCED_FACE ( 'NONE', ( #12805 ), #10093, .T. ) ;
#1254=ORIENTED_EDGE ( 'NONE', *, *, #21788, .F. ) ;
#1258=ORIENTED_EDGE ( 'NONE', *, *, #11197, .F. ) ;
#1264=EDGE_LOOP ( 'NONE', ( #23405, #5716, #4879, #844 ) ) ;
#1266=DIRECTION ( 'NONE',  ( -1.224646799147353207E-16, -1.349345573449484691E-32, 1.000000000000000000 ) ) ;
#1267=ORIENTED_EDGE ( 'NONE', *, *, #2115, .T. ) ;
#1269=CARTESIAN_POINT ( 'NONE',  ( 21.09992658989239089, 24.96183152705960140, 47.04930799450051637 ) ) ;
#1272=AXIS2_PLACEMENT_3D ( 'NONE', #3616, #28729, #21163 ) ;
#1274=DIRECTION ( 'NONE',  ( -1.000000000000000000, 0.000000000000000000, 0.000000000000000000 ) ) ;
#1277=ORIENTED_EDGE ( 'NONE', *, *, #711, .T. ) ;
#1280=CIRCLE ( 'NONE', #5493, 0.1250000000000001110 ) ;
#1282=AXIS2_PLACEMENT_3D ( 'NONE', #25712, #30968, #2899 ) ;
#1284=DIRECTION ( 'NONE',  ( -1.101824276508909887E-16, 1.000000000000000000, -0.000000000000000000 ) ) ;
#1287=DIRECTION ( 'NONE',  ( -1.000000000000000000, 0.000000000000000000, 0.000000000000000000 ) ) ;
#1294=EDGE_CURVE ( 'NONE', #19345, #18749, #642, .T. ) ;
#1297=TOROIDAL_SURFACE ( 'NONE', #778, 12.40141737965288904, 0.1249999999999998612 ) ;
#1304=DIRECTION ( 'NONE',  ( -1.224646799147353207E-16, -1.349345573449484691E-32, 1.000000000000000000 ) ) ;
#1306=VECTOR ( 'NONE', #4417, 1000.000000000000000 ) ;
#1307=ORIENTED_EDGE ( 'NONE', *, *, #13757, .F. ) ;
#1311=VERTEX_POINT ( 'NONE', #2458 ) ;
#1314=CYLINDRICAL_SURFACE ( 'NONE', #9732, 12.36707279061065279 ) ;
#1319=VERTEX_POINT ( 'NONE', #12964 ) ;
#1320=EDGE_CURVE ( 'NONE', #31644, #4648, #25806, .T. ) ;
#1323=FACE_OUTER_BOUND ( 'NONE', #17617, .T. ) ;
#1324=AXIS2_PLACEMENT_3D ( 'NONE', #22136, #32165, #7208 ) ;
#1325=ORIENTED_EDGE ( 'NONE', *, *, #1420, .F. ) ;
#1330=TOROIDAL_SURFACE ( 'NONE', #4473, 12.40141737965281621, 0.1250000000000009159 ) ;
#1334=FACE_OUTER_BOUND ( 'NONE', #579, .T. ) ;
#1335=AXIS2_PLACEMENT_3D ( 'NONE', #21891, #19595, #19435 ) ;
#1337=ADVANCED_FACE ( 'NONE', ( #7876 ), #23185, .T. ) ;
#1338=EDGE_CURVE ( 'NONE', #15696, #1073, #15847, .T. ) ;
#1339=AXIS2_PLACEMENT_3D ( 'NONE', #28718, #16558, #6237 ) ;
#1343=DIRECTION ( 'NONE',  ( 1.000000000000000000, 0.000000000000000000, 0.000000000000000000 ) ) ;
#1347=DIRECTION ( 'NONE',  ( -1.000000000000000000, -1.101824276508910010E-16, 0.000000000000000000 ) ) ;
#1348=CIRCLE ( 'NONE', #5561, 12.36707279061065101 ) ;
#1354=DIRECTION ( 'NONE',  ( 0.000000000000000000, 0.000000000000000000, 1.000000000000000000 ) ) ;
#1355=ORIENTED_EDGE ( 'NONE', *, *, #7152, .T. ) ;
#1360=DIRECTION ( 'NONE',  ( -1.000000000000000000, -1.101824276508909887E-16, 0.000000000000000000 ) ) ;
#1361=DIRECTION ( 'NONE',  ( -1.000000000000000000, 0.000000000000000000, 0.000000000000000000 ) ) ;
#1364=ORIENTED_EDGE ( 'NONE', *, *, #21443, .T. ) ;
#1369=CARTESIAN_POINT ( 'NONE',  ( 8.474859994195282908, 38.56284415653841791, 47.04930799450051637 ) ) ;
#1375=VERTEX_POINT ( 'NONE', #25582 ) ;
#1378=ORIENTED_EDGE ( 'NONE', *, *, #31391, .F. ) ;
#1381=ADVANCED_FACE ( 'NONE', ( #30196 ), #7984, .T. ) ;
#1383=DIRECTION ( 'NONE',  ( -1.101824276508909887E-16, 1.000000000000000000, -0.000000000000000000 ) ) ;
#1384=DIRECTION ( 'NONE',  ( -1.000000000000000000, 0.000000000000000000, 0.000000000000000000 ) ) ;
#1385=EDGE_CURVE ( 'NONE', #10661, #15368, #9022, .T. ) ;
#1391=LINE ( 'NONE', #21247, #8965 ) ;
#1392=VERTEX_POINT ( 'NONE', #20817 ) ;
#1395=DIRECTION ( 'NONE',  ( -1.101824276508909887E-16, 1.000000000000000000, -0.000000000000000000 ) ) ;
#1397=AXIS2_PLACEMENT_3D ( 'NONE', #3502, #11227, #21372 ) ;
#1400=VERTEX_POINT ( 'NONE', #11298 ) ;
#1405=EDGE_CURVE ( 'NONE', #14676, #10661, #3261, .T. ) ;
#1406=DIRECTION ( 'NONE',  ( 0.000000000000000000, -0.000000000000000000, -1.000000000000000000 ) ) ;
#1407=ORIENTED_EDGE ( 'NONE', *, *, #7950, .F. ) ;
#1410=ORIENTED_EDGE ( 'NONE', *, *, #5755, .F. ) ;
#1412=AXIS2_PLACEMENT_3D ( 'NONE', #13319, #28407, #7736 ) ;
#1413=FACE_OUTER_BOUND ( 'NONE', #29852, .T. ) ;
#1414=ORIENTED_EDGE ( 'NONE', *, *, #955, .T. ) ;
#1418=AXIS2_PLACEMENT_3D ( 'NONE', #22607, #24582, #5059 ) ;
#1420=EDGE_CURVE ( 'NONE', #20658, #19118, #20031, .T. ) ;
#1421=DIRECTION ( 'NONE',  ( -1.000000000000000000, 0.000000000000000000, 0.000000000000000000 ) ) ;
#1423=ORIENTED_EDGE ( 'NONE', *, *, #26261, .F. ) ;
#1429=ORIENTED_EDGE ( 'NONE', *, *, #23635, .F. ) ;
#1438=ADVANCED_FACE ( 'NONE', ( #28215 ), #22118, .T. ) ;
#1448=DIRECTION ( 'NONE',  ( -1.101824276508909887E-16, 1.000000000000000000, -0.000000000000000000 ) ) ;
#1451=TOROIDAL_SURFACE ( 'NONE', #31866, 12.40141737965288904, 0.1249999999999998612 ) ;
#1459=CARTESIAN_POINT ( 'NONE',  ( 33.72499318558949710, 31.59184655352418503, 47.04930799450051637 ) ) ;
#1463=EDGE_LOOP ( 'NONE', ( #32458, #3921, #4900, #4428 ) ) ;
#1465=TOROIDAL_SURFACE ( 'NONE', #8296, 12.61792373059898331, 0.1249999999999965583 ) ;
#1471=CARTESIAN_POINT ( 'NONE',  ( 21.09992658989239089, 29.47145308207317882, 47.04930799450051637 ) ) ;
#1474=AXIS2_PLACEMENT_3D ( 'NONE', #17583, #30074, #30231 ) ;
#1477=CARTESIAN_POINT ( 'NONE',  ( 8.474859994195286461, 28.84184655352418858, 47.04930799450051637 ) ) ;
#1479=ORIENTED_EDGE ( 'NONE', *, *, #19983, .T. ) ;
#1485=DIRECTION ( 'NONE',  ( -1.101824276508909887E-16, 1.000000000000000000, -0.000000000000000000 ) ) ;
#1487=ORIENTED_EDGE ( 'NONE', *, *, #15824, .F. ) ;
#1490=CIRCLE ( 'NONE', #7811, 12.36707279061065101 ) ;
#1492=CARTESIAN_POINT ( 'NONE',  ( 33.72499318558949710, 29.34184655352418858, 47.04930799450051637 ) ) ;
#1497=ORIENTED_EDGE ( 'NONE', *, *, #22865, .F. ) ;
#1499=CARTESIAN_POINT ( 'NONE',  ( 8.474859994195286461, 30.09143805560860585, 47.04930799450051637 ) ) ;
#1502=ORIENTED_EDGE ( 'NONE', *, *, #7949, .T. ) ;
#1503=FACE_OUTER_BOUND ( 'NONE', #29236, .T. ) ;
#1507=CIRCLE ( 'NONE', #12003, 12.27641737965281266 ) ;
#1510=DIRECTION ( 'NONE',  ( -1.000000000000000000, -1.101824276508909887E-16, 0.000000000000000000 ) ) ;
#1517=EDGE_LOOP ( 'NONE', ( #29288, #17413, #14062, #5917 ) ) ;
#1518=DIRECTION ( 'NONE',  ( -1.101824276508909887E-16, 1.000000000000000000, -0.000000000000000000 ) ) ;
#1523=ORIENTED_EDGE ( 'NONE', *, *, #1031, .F. ) ;
#1525=AXIS2_PLACEMENT_3D ( 'NONE', #173, #7567, #2636 ) ;
#1530=CARTESIAN_POINT ( 'NONE',  ( 33.71785032049138664, 23.96664230456639899, 47.04930799450051637 ) ) ;
#1536=AXIS2_PLACEMENT_3D ( 'NONE', #16619, #1054, #21066 ) ;
#1538=EDGE_CURVE ( 'NONE', #16672, #11669, #29014, .T. ) ;
#1539=ADVANCED_FACE ( 'NONE', ( #21613 ), #14826, .T. ) ;
#1541=CIRCLE ( 'NONE', #1019, 12.62506659569710266 ) ;
#1545=AXIS2_PLACEMENT_3D ( 'NONE', #3835, #18755, #3997 ) ;
#1548=ORIENTED_EDGE ( 'NONE', *, *, #14796, .F. ) ;
#1553=DIRECTION ( 'NONE',  ( 0.000000000000000000, -0.000000000000000000, -1.000000000000000000 ) ) ;
#1556=AXIS2_PLACEMENT_3D ( 'NONE', #19758, #17627, #12558 ) ;
#1561=CARTESIAN_POINT ( 'NONE',  ( 33.46699938050303302, 38.56284415653841791, 47.04930799450051637 ) ) ;
#1568=FACE_OUTER_BOUND ( 'NONE', #14914, .T. ) ;
#1570=AXIS2_PLACEMENT_3D ( 'NONE', #7904, #5439, #15768 ) ;
#1571=LINE ( 'NONE', #16660, #17978 ) ;
#1579=ORIENTED_EDGE ( 'NONE', *, *, #29541, .F. ) ;
#1580=EDGE_CURVE ( 'NONE', #2178, #10687, #25386, .T. ) ;
#1583=LINE ( 'NONE', #26862, #8802 ) ;
#1594=CIRCLE ( 'NONE', #5809, 12.36707279061065101 ) ;
#1596=CARTESIAN_POINT ( 'NONE',  ( 21.09992658989239089, 24.97145308207319303, 47.04930799450051637 ) ) ;
#1597=ORIENTED_EDGE ( 'NONE', *, *, #31123, .F. ) ;
#1604=CARTESIAN_POINT ( 'NONE',  ( 33.72499318558949710, 26.09143805560860940, 47.04930799450051637 ) ) ;
#1608=ORIENTED_EDGE ( 'NONE', *, *, #11781, .T. ) ;
#1612=DIRECTION ( 'NONE',  ( -1.101824276508909887E-16, 1.000000000000000000, -0.000000000000000000 ) ) ;
#1619=FACE_OUTER_BOUND ( 'NONE', #12270, .T. ) ;
#1621=EDGE_CURVE ( 'NONE', #27550, #112, #2254, .T. ) ;
#1627=ADVANCED_FACE ( 'NONE', ( #7342 ), #12200, .T. ) ;
#1628=ORIENTED_EDGE ( 'NONE', *, *, #5035, .F. ) ;
#1637=ORIENTED_EDGE ( 'NONE', *, *, #10423, .T. ) ;
#1642=DIRECTION ( 'NONE',  ( -1.101824276508909887E-16, 1.000000000000000000, -0.000000000000000000 ) ) ;
#1647=ORIENTED_EDGE ( 'NONE', *, *, #18364, .T. ) ;
#1649=AXIS2_PLACEMENT_3D ( 'NONE', #31446, #1395, #8950 ) ;
#1657=ORIENTED_EDGE ( 'NONE', *, *, #29871, .F. ) ;
#1660=CIRCLE ( 'NONE', #29454, 0.1249999999999983763 ) ;
#1665=VECTOR ( 'NONE', #9472, 1000.000000000000000 ) ;
#1671=ORIENTED_EDGE ( 'NONE', *, *, #9993, .F. ) ;
#1679=DIRECTION ( 'NONE',  ( 0.000000000000000000, -0.000000000000000000, -1.000000000000000000 ) ) ;
#1680=VECTOR ( 'NONE', #31721, 1000.000000000000000 ) ;
#1681=DIRECTION ( 'NONE',  ( -1.000000000000000000, -1.101824276508910010E-16, 0.000000000000000000 ) ) ;
#1687=CARTESIAN_POINT ( 'NONE',  ( 21.09992658989238734, 31.59143805560860585, 47.04930799450051637 ) ) ;
#1690=CIRCLE ( 'NONE', #18969, 0.1250000000000001110 ) ;
#1694=DIRECTION ( 'NONE',  ( -1.101824276508909887E-16, 1.000000000000000000, -0.000000000000000000 ) ) ;
#1695=EDGE_LOOP ( 'NONE', ( #32328, #18815, #6147, #19536 ) ) ;
#1696=DIRECTION ( 'NONE',  ( -1.101824276508909887E-16, 1.000000000000000000, -0.000000000000000000 ) ) ;
#1700=ORIENTED_EDGE ( 'NONE', *, *, #27158, .F. ) ;
#1702=EDGE_LOOP ( 'NONE', ( #19188, #4075, #21485, #17491 ) ) ;
#1704=ORIENTED_EDGE ( 'NONE', *, *, #19291, .T. ) ;
#1706=EDGE_CURVE ( 'NONE', #17323, #12553, #24768, .T. ) ;
#1714=AXIS2_PLACEMENT_3D ( 'NONE', #23583, #11123, #10807 ) ;
#1725=CARTESIAN_POINT ( 'NONE',  ( 21.09992658989238734, 38.56284415653841791, 47.04930799450051637 ) ) ;
#1729=FACE_OUTER_BOUND ( 'NONE', #28058, .T. ) ;
#1731=CARTESIAN_POINT ( 'NONE',  ( 8.732853799281738105, 30.46183152705961561, 47.04930799450051637 ) ) ;
#1732=ORIENTED_EDGE ( 'NONE', *, *, #16074, .T. ) ;
#1733=CARTESIAN_POINT ( 'NONE',  ( 21.09992658989239089, 28.09164230456639544, 47.04930799450051637 ) ) ;
#1734=CYLINDRICAL_SURFACE ( 'NONE', #11748, 12.36707279061065279 ) ;
#1738=ADVANCED_FACE ( 'NONE', ( #11110 ), #26184, .F. ) ;
#1739=DIRECTION ( 'NONE',  ( -1.101824276508909887E-16, 1.000000000000000000, -0.000000000000000000 ) ) ;
#1740=ORIENTED_EDGE ( 'NONE', *, *, #6664, .F. ) ;
#1741=CIRCLE ( 'NONE', #24274, 12.36707279061065101 ) ;
#1746=EDGE_CURVE ( 'NONE', #17665, #27575, #6430, .T. ) ;
#1748=AXIS2_PLACEMENT_3D ( 'NONE', #5290, #25308, #30395 ) ;
#1751=ORIENTED_EDGE ( 'NONE', *, *, #19877, .F. ) ;
#1752=CARTESIAN_POINT ( 'NONE',  ( 21.09992658989239089, 25.46183152705960140, 47.04930799450051637 ) ) ;
#1753=AXIS2_PLACEMENT_3D ( 'NONE', #7802, #25993, #23048 ) ;
#1754=DIRECTION ( 'NONE',  ( -1.101824276508909887E-16, 1.000000000000000000, -0.000000000000000000 ) ) ;
#1756=CIRCLE ( 'NONE', #28514, 0.1250000000000001110 ) ;
#1758=DIRECTION ( 'NONE',  ( -1.101824276508909887E-16, 1.000000000000000000, -0.000000000000000000 ) ) ;
#1766=EDGE_CURVE ( 'NONE', #12417, #27575, #16173, .T. ) ;
#1769=CARTESIAN_POINT ( 'NONE',  ( 8.732853799281734553, 38.56284415653841791, 47.04930799450051637 ) ) ;
#1770=DIRECTION ( 'NONE',  ( -1.000000000000000000, 0.000000000000000000, 0.000000000000000000 ) ) ;
#1775=CARTESIAN_POINT ( 'NONE',  ( 33.71785032049135111, 27.46664230456639899, 47.04930799450051637 ) ) ;
#1780=CIRCLE ( 'NONE', #13322, 12.27641737965283042 ) ;
#1781=DIRECTION ( 'NONE',  ( -1.000000000000000000, 0.000000000000000000, 0.000000000000000000 ) ) ;
#1783=ORIENTED_EDGE ( 'NONE', *, *, #8175, .F. ) ;
#1784=CARTESIAN_POINT ( 'NONE',  ( 33.72499318558949710, 30.59184655352422411, 47.04930799450051637 ) ) ;
#1785=ORIENTED_EDGE ( 'NONE', *, *, #13241, .T. ) ;
#1786=CARTESIAN_POINT ( 'NONE',  ( 21.09992658989238734, 38.56284415653841791, 47.04930799450051637 ) ) ;
#1793=CARTESIAN_POINT ( 'NONE',  ( 8.823509210239526723, 26.09164230456639899, 47.04930799450051637 ) ) ;
#1795=CARTESIAN_POINT ( 'NONE',  ( 33.50134396954518223, 32.59164230456639899, 47.04930799450051637 ) ) ;
#1811=ORIENTED_EDGE ( 'NONE', *, *, #16257, .F. ) ;
#1813=CARTESIAN_POINT ( 'NONE',  ( 21.09992658989239089, 27.59164230456639544, 47.04930799450051637 ) ) ;
#1821=EDGE_LOOP ( 'NONE', ( #10516, #4936, #4488, #13134 ) ) ;
#1825=VECTOR ( 'NONE', #8073, 1000.000000000000000 ) ;
#1831=FACE_OUTER_BOUND ( 'NONE', #26578, .T. ) ;
#1836=CARTESIAN_POINT ( 'NONE',  ( 21.09992658989239089, 29.84164230456639899, 47.04930799450051637 ) ) ;
#1837=EDGE_CURVE ( 'NONE', #5204, #8602, #26814, .T. ) ;
#1840=CARTESIAN_POINT ( 'NONE',  ( 21.09992658989239089, 28.96664230456639899, 47.04930799450051637 ) ) ;
#1844=CIRCLE ( 'NONE', #18607, 0.1250000000000001110 ) ;
#1848=VECTOR ( 'NONE', #1885, 1000.000000000000000 ) ;
#1849=CIRCLE ( 'NONE', #5001, 0.1250000000000001110 ) ;
#1851=EDGE_CURVE ( 'NONE', #25423, #22382, #26024, .T. ) ;
#1861=EDGE_LOOP ( 'NONE', ( #29758, #1487, #31150, #31943 ) ) ;
#1870=DIRECTION ( 'NONE',  ( -1.101824276508909887E-16, 1.000000000000000000, -0.000000000000000000 ) ) ;
#1874=CARTESIAN_POINT ( 'NONE',  ( 21.09992658989239089, 24.71183152705960140, 47.04930799450051637 ) ) ;
#1881=CARTESIAN_POINT ( 'NONE',  ( 21.09992658989239089, 26.71664230456639899, 47.04930799450051637 ) ) ;
#1885=DIRECTION ( 'NONE',  ( -1.101824276508909887E-16, 1.000000000000000000, -0.000000000000000000 ) ) ;
#1886=CARTESIAN_POINT ( 'NONE',  ( 8.732853799281732776, 27.47145308207318237, 47.04930799450051637 ) ) ;
#1892=FACE_OUTER_BOUND ( 'NONE', #30186, .T. ) ;
#1896=DIRECTION ( 'NONE',  ( -1.101824276508909887E-16, 1.000000000000000000, -0.000000000000000000 ) ) ;
#1900=MECHANICAL_DESIGN_GEOMETRIC_PRESENTATION_REPRESENTATION('',(#11858),#30216);
#1901=DIRECTION ( 'NONE',  ( -1.101824276508909887E-16, 1.000000000000000000, -0.000000000000000000 ) ) ;
#1910=DIRECTION ( 'NONE',  ( -1.000000000000000000, 0.000000000000000000, 0.000000000000000000 ) ) ;
#1917=ORIENTED_EDGE ( 'NONE', *, *, #28279, .F. ) ;
#1921=DIRECTION ( 'NONE',  ( -1.101824276508909887E-16, 1.000000000000000000, -0.000000000000000000 ) ) ;
#1923=DIRECTION ( 'NONE',  ( -1.000000000000000000, 0.000000000000000000, 0.000000000000000000 ) ) ;
#1940=VERTEX_POINT ( 'NONE', #6494 ) ;
#1941=DIRECTION ( 'NONE',  ( -1.000000000000000000, 0.000000000000000000, 0.000000000000000000 ) ) ;
#1947=CARTESIAN_POINT ( 'NONE',  ( 33.72499318558949710, 30.84184655352422411, 47.04930799450051637 ) ) ;
#1948=ADVANCED_FACE ( 'NONE', ( #24212 ), #8785, .T. ) ;
#1949=CARTESIAN_POINT ( 'NONE',  ( 21.09992658989239089, 27.72145308207318237, 47.04930799450051637 ) ) ;
#1952=ORIENTED_EDGE ( 'NONE', *, *, #11352, .T. ) ;
#1954=CARTESIAN_POINT ( 'NONE',  ( 8.474859994195282908, 38.56284415653841791, 47.04930799450051637 ) ) ;
#1955=CIRCLE ( 'NONE', #21866, 12.36707279061065101 ) ;
#1956=DIRECTION ( 'NONE',  ( 0.000000000000000000, -0.000000000000000000, -1.000000000000000000 ) ) ;
#1962=ORIENTED_EDGE ( 'NONE', *, *, #4009, .T. ) ;
#1963=DIRECTION ( 'NONE',  ( 1.000000000000000000, 0.000000000000000000, 0.000000000000000000 ) ) ;
#1964=DIRECTION ( 'NONE',  ( -1.101824276508909887E-16, 1.000000000000000000, -0.000000000000000000 ) ) ;
#1966=TOROIDAL_SURFACE ( 'NONE', #22937, 12.61792373059890693, 0.1250000000000019429 ) ;
#1967=DIRECTION ( 'NONE',  ( -1.101824276508909887E-16, 1.000000000000000000, -0.000000000000000000 ) ) ;
#1972=DIRECTION ( 'NONE',  ( -1.000000000000000000, 0.000000000000000000, 0.000000000000000000 ) ) ;
#1979=DIRECTION ( 'NONE',  ( -1.101824276508909887E-16, 1.000000000000000000, -0.000000000000000000 ) ) ;
#1980=DIRECTION ( 'NONE',  ( -1.101824276508909887E-16, 1.000000000000000000, -0.000000000000000000 ) ) ;
#1981=DIRECTION ( 'NONE',  ( -1.101824276508909887E-16, 1.000000000000000000, -0.000000000000000000 ) ) ;
#1984=CIRCLE ( 'NONE', #9326, 12.36707279061065279 ) ;
#1989=DIRECTION ( 'NONE',  ( -1.000000000000000000, 0.000000000000000000, 0.000000000000000000 ) ) ;
#1995=ORIENTED_EDGE ( 'NONE', *, *, #15821, .T. ) ;
#1996=ADVANCED_FACE ( 'NONE', ( #2860 ), #9931, .T. ) ;
#1997=CARTESIAN_POINT ( 'NONE',  ( 33.71785032049099584, 30.96664230456641675, 47.04930799450051637 ) ) ;
#2000=CARTESIAN_POINT ( 'NONE',  ( 21.09992658989238734, 32.59164230456639899, 47.04930799450051637 ) ) ;
#2001=CARTESIAN_POINT ( 'NONE',  ( 8.698509210239571132, 30.34164230456639544, 47.04930799450051637 ) ) ;
#2004=FACE_OUTER_BOUND ( 'NONE', #10096, .T. ) ;
#2006=EDGE_CURVE ( 'NONE', #16515, #15368, #32070, .T. ) ;
#2007=VERTEX_POINT ( 'NONE', #27650 ) ;
#2018=FACE_OUTER_BOUND ( 'NONE', #29941, .T. ) ;
#2019=AXIS2_PLACEMENT_3D ( 'NONE', #9128, #1247, #29308 ) ;
#2020=ORIENTED_EDGE ( 'NONE', *, *, #7856, .F. ) ;
#2021=VERTEX_POINT ( 'NONE', #24868 ) ;
#2025=AXIS2_PLACEMENT_3D ( 'NONE', #31213, #23969, #11345 ) ;
#2026=DIRECTION ( 'NONE',  ( -1.000000000000000000, -1.101824276508909887E-16, 0.000000000000000000 ) ) ;
#2027=VERTEX_POINT ( 'NONE', #9607 ) ;
#2029=ORIENTED_EDGE ( 'NONE', *, *, #14198, .F. ) ;
#2031=EDGE_CURVE ( 'NONE', #28434, #15217, #25759, .T. ) ;
#2032=ORIENTED_EDGE ( 'NONE', *, *, #25394, .F. ) ;
#2041=VERTEX_POINT ( 'NONE', #17475 ) ;
#2042=CIRCLE ( 'NONE', #6239, 0.1250000000000001110 ) ;
#2044=ORIENTED_EDGE ( 'NONE', *, *, #26227, .F. ) ;
#2048=ORIENTED_EDGE ( 'NONE', *, *, #29916, .F. ) ;
#2049=CARTESIAN_POINT ( 'NONE',  ( 21.09992658989239089, 25.09164230456639899, 47.04930799450051637 ) ) ;
#2050=CYLINDRICAL_SURFACE ( 'NONE', #4327, 12.36707279061065101 ) ;
#2058=DIRECTION ( 'NONE',  ( -1.000000000000000000, 0.000000000000000000, 0.000000000000000000 ) ) ;
#2062=CIRCLE ( 'NONE', #31939, 12.62506659569710266 ) ;
#2064=VERTEX_POINT ( 'NONE', #12404 ) ;
#2066=AXIS2_PLACEMENT_3D ( 'NONE', #1530, #9418, #26972 ) ;
#2067=ORIENTED_EDGE ( 'NONE', *, *, #49, .F. ) ;
#2070=ADVANCED_FACE ( 'NONE', ( #27494 ), #29966, .T. ) ;
#2072=EDGE_CURVE ( 'NONE', #12553, #7860, #31016, .T. ) ;
#2075=ORIENTED_EDGE ( 'NONE', *, *, #32083, .T. ) ;
#2076=EDGE_LOOP ( 'NONE', ( #17495, #22198, #1962, #16896 ) ) ;
#2078=DIRECTION ( 'NONE',  ( -1.000000000000000000, 0.000000000000000000, 0.000000000000000000 ) ) ;
#2080=CARTESIAN_POINT ( 'NONE',  ( 21.09992658989239089, 23.71183152705959429, 47.04930799450051637 ) ) ;
#2082=EDGE_LOOP ( 'NONE', ( #15005, #21265, #17984, #14405 ) ) ;
#2089=TOROIDAL_SURFACE ( 'NONE', #19894, 12.40141737965280022, 0.1249999999999992228 ) ;
#2090=TOROIDAL_SURFACE ( 'NONE', #31989, 12.61792373059896200, 0.1249999999999979183 ) ;
#2093=CARTESIAN_POINT ( 'NONE',  ( 33.46699938050304013, 25.22145308207319303, 47.04930799450050927 ) ) ;
#2096=DIRECTION ( 'NONE',  ( -1.000000000000000000, 0.000000000000000000, 0.000000000000000000 ) ) ;
#2097=ORIENTED_EDGE ( 'NONE', *, *, #6002, .F. ) ;
#2100=AXIS2_PLACEMENT_3D ( 'NONE', #6138, #1696, #11716 ) ;
#2101=DIRECTION ( 'NONE',  ( -1.101824276508909887E-16, 1.000000000000000000, -0.000000000000000000 ) ) ;
#2107=CARTESIAN_POINT ( 'NONE',  ( 21.09992658989238734, 31.09164230456639544, 47.04930799450051637 ) ) ;
#2108=CIRCLE ( 'NONE', #27820, 12.52641737965288904 ) ;
#2110=EDGE_CURVE ( 'NONE', #3554, #1319, #4271, .T. ) ;
#2115=EDGE_CURVE ( 'NONE', #25631, #5457, #8469, .T. ) ;
#2117=ORIENTED_EDGE ( 'NONE', *, *, #14572, .T. ) ;
#2118=EDGE_CURVE ( 'NONE', #31159, #14982, #10591, .T. ) ;
#2119=EDGE_CURVE ( 'NONE', #14676, #16515, #11127, .T. ) ;
#2122=TOROIDAL_SURFACE ( 'NONE', #18854, 12.40141737965281621, 0.1250000000000009159 ) ;
#2124=VERTEX_POINT ( 'NONE', #18588 ) ;
#2141=ORIENTED_EDGE ( 'NONE', *, *, #29004, .F. ) ;
#2145=CARTESIAN_POINT ( 'NONE',  ( 8.474859994195282908, 38.56284415653841791, 47.04930799450051637 ) ) ;
#2149=CARTESIAN_POINT ( 'NONE',  ( 8.732853799281738105, 25.71183152705960140, 47.04930799450051637 ) ) ;
#2150=AXIS2_PLACEMENT_3D ( 'NONE', #346, #4958, #2966 ) ;
#2155=EDGE_CURVE ( 'NONE', #30753, #31841, #26830, .T. ) ;
#2156=AXIS2_PLACEMENT_3D ( 'NONE', #13055, #17960, #18436 ) ;
#2157=DIRECTION ( 'NONE',  ( 0.000000000000000000, -0.000000000000000000, -1.000000000000000000 ) ) ;
#2163=CARTESIAN_POINT ( 'NONE',  ( 8.474859994195282908, 38.56284415653841791, 47.04930799450051637 ) ) ;
#2168=TOROIDAL_SURFACE ( 'NONE', #3729, 12.40141737965280555, 0.1250000000000006939 ) ;
#2174=CARTESIAN_POINT ( 'NONE',  ( 21.09992658989238734, 38.56284415653841791, 47.04930799450051637 ) ) ;
#2175=CARTESIAN_POINT ( 'NONE',  ( 8.698509210239507183, 24.09164230456639544, 47.04930799450051637 ) ) ;
#2178=VERTEX_POINT ( 'NONE', #26147 ) ;
#2184=FACE_OUTER_BOUND ( 'NONE', #24835, .T. ) ;
#2188=CARTESIAN_POINT ( 'NONE',  ( 21.09992658989239089, 24.84164230456639544, 47.04930799450051637 ) ) ;
#2189=ORIENTED_EDGE ( 'NONE', *, *, #15032, .T. ) ;
#2194=EDGE_CURVE ( 'NONE', #13126, #21006, #21056, .T. ) ;
#2205=ORIENTED_EDGE ( 'NONE', *, *, #12784, .F. ) ;
#2211=ORIENTED_EDGE ( 'NONE', *, *, #23688, .T. ) ;
#2218=LINE ( 'NONE', #6977, #1848 ) ;
#2224=EDGE_LOOP ( 'NONE', ( #3469, #18305, #23139, #26666 ) ) ;
#2225=CARTESIAN_POINT ( 'NONE',  ( 21.09992658989238734, 31.34184655352422766, 47.04930799450051637 ) ) ;
#2229=DIRECTION ( 'NONE',  ( -1.000000000000000000, 0.000000000000000000, 0.000000000000000000 ) ) ;
#2239=CARTESIAN_POINT ( 'NONE',  ( 33.71785032049134401, 28.21664230456639899, 47.04930799450051637 ) ) ;
#2244=CARTESIAN_POINT ( 'NONE',  ( 21.09992658989238734, 38.56284415653841791, 47.04930799450051637 ) ) ;
#2249=DIRECTION ( 'NONE',  ( -1.000000000000000000, 0.000000000000000000, 0.000000000000000000 ) ) ;
#2250=VERTEX_POINT ( 'NONE', #25434 ) ;
#2252=ORIENTED_EDGE ( 'NONE', *, *, #26261, .T. ) ;
#2254=LINE ( 'NONE', #4716, #27916 ) ;
#2258=ADVANCED_FACE ( 'NONE', ( #20179 ), #3094, .F. ) ;
#2261=LINE ( 'NONE', #29841, #23746 ) ;
#2264=AXIS2_PLACEMENT_3D ( 'NONE', #20141, #15067, #20297 ) ;
#2266=CARTESIAN_POINT ( 'NONE',  ( 21.09992658989239089, 28.09143805560861296, 47.04930799450051637 ) ) ;
#2267=VERTEX_POINT ( 'NONE', #13133 ) ;
#2270=ORIENTED_EDGE ( 'NONE', *, *, #18446, .F. ) ;
#2275=ORIENTED_EDGE ( 'NONE', *, *, #262, .T. ) ;
#2276=DIRECTION ( 'NONE',  ( -1.101824276508909887E-16, 1.000000000000000000, -0.000000000000000000 ) ) ;
#2277=ORIENTED_EDGE ( 'NONE', *, *, #32113, .T. ) ;
#2287=CARTESIAN_POINT ( 'NONE',  ( 21.09992658989239089, 23.84184655352419213, 47.04930799450051637 ) ) ;
#2298=CIRCLE ( 'NONE', #6486, 0.1250000000000001110 ) ;
#2303=ORIENTED_EDGE ( 'NONE', *, *, #4028, .F. ) ;
#2308=ADVANCED_FACE ( 'NONE', ( #22469 ), #25270, .T. ) ;
#2322=AXIS2_PLACEMENT_3D ( 'NONE', #5370, #12921, #15687 ) ;
#2329=DIRECTION ( 'NONE',  ( -1.000000000000000000, 0.000000000000000000, 0.000000000000000000 ) ) ;
#2338=DIRECTION ( 'NONE',  ( -1.000000000000000000, 0.000000000000000000, 0.000000000000000000 ) ) ;
#2340=ORIENTED_EDGE ( 'NONE', *, *, #16245, .T. ) ;
#2342=CARTESIAN_POINT ( 'NONE',  ( 33.72499318558949000, 38.56284415653841791, 47.04930799450051637 ) ) ;
#2346=DIRECTION ( 'NONE',  ( -1.000000000000000000, 0.000000000000000000, 0.000000000000000000 ) ) ;
#2349=EDGE_CURVE ( 'NONE', #63, #14845, #17884, .T. ) ;
#2351=DIRECTION ( 'NONE',  ( -1.101824276508909887E-16, 1.000000000000000000, -0.000000000000000000 ) ) ;
#2362=LINE ( 'NONE', #7286, #1034 ) ;
#2363=DIRECTION ( 'NONE',  ( -1.101824276508909887E-16, 1.000000000000000000, -0.000000000000000000 ) ) ;
#2366=ORIENTED_EDGE ( 'NONE', *, *, #387, .F. ) ;
#2367=ORIENTED_EDGE ( 'NONE', *, *, #7537, .F. ) ;
#2372=CARTESIAN_POINT ( 'NONE',  ( 21.09992658989239089, 29.71183152705961561, 47.04930799450051637 ) ) ;
#2377=ADVANCED_FACE ( 'NONE', ( #28694 ), #25755, .F. ) ;
#2382=DIRECTION ( 'NONE',  ( -1.000000000000000000, -1.101824276508910010E-16, 0.000000000000000000 ) ) ;
#2383=DIRECTION ( 'NONE',  ( -1.101824276508909887E-16, 1.000000000000000000, -0.000000000000000000 ) ) ;
#2384=VERTEX_POINT ( 'NONE', #6061 ) ;
#2386=CARTESIAN_POINT ( 'NONE',  ( 21.09992658989238734, 38.56284415653841791, 47.04930799450051637 ) ) ;
#2392=DIRECTION ( 'NONE',  ( -1.000000000000000000, 0.000000000000000000, 0.000000000000000000 ) ) ;
#2395=EDGE_CURVE ( 'NONE', #16985, #13978, #11459, .T. ) ;
#2396=CARTESIAN_POINT ( 'NONE',  ( 21.09992658989238734, 38.56284415653841791, 47.04930799450051637 ) ) ;
#2397=CYLINDRICAL_SURFACE ( 'NONE', #18502, 12.36707279061065101 ) ;
#2401=AXIS2_PLACEMENT_3D ( 'NONE', #18268, #13216, #8748 ) ;
#2402=ORIENTED_EDGE ( 'NONE', *, *, #17078, .T. ) ;
#2403=EDGE_CURVE ( 'NONE', #27591, #9758, #4892, .T. ) ;
#2411=FACE_OUTER_BOUND ( 'NONE', #20446, .T. ) ;
#2416=ORIENTED_EDGE ( 'NONE', *, *, #23784, .F. ) ;
#2418=EDGE_LOOP ( 'NONE', ( #26739, #13481, #9987, #17226 ) ) ;
#2419=CARTESIAN_POINT ( 'NONE',  ( 21.09992658989239089, 25.09184655352419213, 47.04930799450051637 ) ) ;
#2424=DIRECTION ( 'NONE',  ( -1.000000000000000000, 0.000000000000000000, 0.000000000000000000 ) ) ;
#2427=FACE_OUTER_BOUND ( 'NONE', #23670, .T. ) ;
#2430=CARTESIAN_POINT ( 'NONE',  ( 21.09992658989238734, 31.59184655352418503, 47.04930799450051637 ) ) ;
#2433=FACE_OUTER_BOUND ( 'NONE', #2418, .T. ) ;
#2436=CIRCLE ( 'NONE', #25489, 12.62506659569710266 ) ;
#2437=CARTESIAN_POINT ( 'NONE',  ( 8.698509210239548040, 28.09164230456639544, 47.04930799450051637 ) ) ;
#2440=CARTESIAN_POINT ( 'NONE',  ( 21.09992658989239089, 29.09164230456639899, 47.04930799450051637 ) ) ;
#2444=ORIENTED_EDGE ( 'NONE', *, *, #12081, .T. ) ;
#2446=ORIENTED_EDGE ( 'NONE', *, *, #12465, .T. ) ;
#2452=EDGE_CURVE ( 'NONE', #15022, #19678, #30061, .T. ) ;
#2458=CARTESIAN_POINT ( 'NONE',  ( 8.474859994195286461, 24.84143805560860940, 47.04930799450051637 ) ) ;
#2459=ORIENTED_EDGE ( 'NONE', *, *, #29086, .F. ) ;
#2461=DIRECTION ( 'NONE',  ( -1.101824276508909887E-16, 1.000000000000000000, -0.000000000000000000 ) ) ;
#2462=DIRECTION ( 'NONE',  ( -1.101824276508909887E-16, 1.000000000000000000, -0.000000000000000000 ) ) ;
#2469=AXIS2_PLACEMENT_3D ( 'NONE', #9577, #14503, #4644 ) ;
#2470=CARTESIAN_POINT ( 'NONE',  ( 21.09992658989238734, 38.56284415653841791, 47.04930799450051637 ) ) ;
#2475=FACE_OUTER_BOUND ( 'NONE', #10012, .T. ) ;
#2481=AXIS2_PLACEMENT_3D ( 'NONE', #20226, #2351, #30251 ) ;
#2486=EDGE_CURVE ( 'NONE', #7948, #25895, #16934, .T. ) ;
#2490=FACE_OUTER_BOUND ( 'NONE', #13565, .T. ) ;
#2495=DIRECTION ( 'NONE',  ( -1.000000000000000000, 0.000000000000000000, 0.000000000000000000 ) ) ;
#2506=LINE ( 'NONE', #12858, #30280 ) ;
#2510=ORIENTED_EDGE ( 'NONE', *, *, #19097, .T. ) ;
#2513=AXIS2_PLACEMENT_3D ( 'NONE', #3595, #31183, #18047 ) ;
#2518=CIRCLE ( 'NONE', #5149, 12.36707279061065279 ) ;
#2520=FACE_OUTER_BOUND ( 'NONE', #1517, .T. ) ;
#2521=ORIENTED_EDGE ( 'NONE', *, *, #29812, .F. ) ;
#2524=EDGE_CURVE ( 'NONE', #27647, #17361, #29345, .T. ) ;
#2525=DIRECTION ( 'NONE',  ( -1.101824276508909887E-16, 1.000000000000000000, -0.000000000000000000 ) ) ;
#2527=EDGE_CURVE ( 'NONE', #9420, #29931, #8567, .T. ) ;
#2528=AXIS2_PLACEMENT_3D ( 'NONE', #22537, #27632, #25010 ) ;
#2533=AXIS2_PLACEMENT_3D ( 'NONE', #30091, #358, #7598 ) ;
#2534=DIRECTION ( 'NONE',  ( -1.101824276508909887E-16, 1.000000000000000000, -0.000000000000000000 ) ) ;
#2536=( NAMED_UNIT ( * ) SI_UNIT ( $, .STERADIAN. ) SOLID_ANGLE_UNIT ( ) );
#2537=VERTEX_POINT ( 'NONE', #18995 ) ;
#2540=CARTESIAN_POINT ( 'NONE',  ( 8.698509210239517842, 25.34164230456639899, 47.04930799450051637 ) ) ;
#2549=DIRECTION ( 'NONE',  ( -1.000000000000000000, 0.000000000000000000, 0.000000000000000000 ) ) ;
#2551=DIRECTION ( 'NONE',  ( 0.000000000000000000, -0.000000000000000000, -1.000000000000000000 ) ) ;
#2559=CIRCLE ( 'NONE', #21396, 12.27641737965283397 ) ;
#2570=VERTEX_POINT ( 'NONE', #26557 ) ;
#2573=DIRECTION ( 'NONE',  ( -1.000000000000000000, 0.000000000000000000, 0.000000000000000000 ) ) ;
#2578=DIRECTION ( 'NONE',  ( -1.000000000000000000, -1.101824276508909887E-16, 0.000000000000000000 ) ) ;
#2589=CARTESIAN_POINT ( 'NONE',  ( 8.732853799281734553, 38.56284415653841791, 47.04930799450051637 ) ) ;
#2592=AXIS2_PLACEMENT_3D ( 'NONE', #13616, #19001, #31663 ) ;
#2600=ORIENTED_EDGE ( 'NONE', *, *, #17148, .F. ) ;
#2603=ORIENTED_EDGE ( 'NONE', *, *, #17117, .F. ) ;
#2609=AXIS2_PLACEMENT_3D ( 'NONE', #9333, #24100, #29358 ) ;
#2615=ORIENTED_EDGE ( 'NONE', *, *, #2737, .F. ) ;
#2616=DIRECTION ( 'NONE',  ( -1.000000000000000000, 0.000000000000000000, 0.000000000000000000 ) ) ;
#2623=EDGE_CURVE ( 'NONE', #16795, #10074, #24416, .T. ) ;
#2630=CIRCLE ( 'NONE', #11519, 0.1250000000000001110 ) ;
#2632=FACE_OUTER_BOUND ( 'NONE', #29935, .T. ) ;
#2633=ORIENTED_EDGE ( 'NONE', *, *, #5229, .F. ) ;
#2636=DIRECTION ( 'NONE',  ( -1.000000000000000000, -1.101824276508909887E-16, 0.000000000000000000 ) ) ;
#2639=CIRCLE ( 'NONE', #24632, 12.36707279061065101 ) ;
#2647=DIRECTION ( 'NONE',  ( -1.101824276508909887E-16, 1.000000000000000000, -0.000000000000000000 ) ) ;
#2656=CYLINDRICAL_SURFACE ( 'NONE', #5032, 12.62506659569710266 ) ;
#2665=AXIS2_PLACEMENT_3D ( 'NONE', #20127, #7170, #17167 ) ;
#2666=ORIENTED_EDGE ( 'NONE', *, *, #22445, .F. ) ;
#2670=CARTESIAN_POINT ( 'NONE',  ( 21.09992658989239089, 24.09164230456639544, 47.04930799450051637 ) ) ;
#2688=AXIS2_PLACEMENT_3D ( 'NONE', #14002, #16605, #1681 ) ;
#2698=DIRECTION ( 'NONE',  ( -1.101824276508909887E-16, 1.000000000000000000, -0.000000000000000000 ) ) ;
#2705=DIRECTION ( 'NONE',  ( -1.000000000000000000, 0.000000000000000000, 0.000000000000000000 ) ) ;
#2706=LINE ( 'NONE', #10754, #31338 ) ;
#2707=VECTOR ( 'NONE', #8596, 1000.000000000000000 ) ;
#2710=VECTOR ( 'NONE', #28353, 1000.000000000000000 ) ;
#2711=CARTESIAN_POINT ( 'NONE',  ( 21.09992658989238734, 32.09164230456639899, 47.04930799450051637 ) ) ;
#2714=DIRECTION ( 'NONE',  ( -1.101824276508909887E-16, 1.000000000000000000, -0.000000000000000000 ) ) ;
#2716=EDGE_CURVE ( 'NONE', #32455, #14337, #8035, .T. ) ;
#2717=CARTESIAN_POINT ( 'NONE',  ( 8.482002859293443109, 28.46664230456639899, 47.04930799450051637 ) ) ;
#2718=EDGE_CURVE ( 'NONE', #14523, #2027, #20604, .T. ) ;
#2721=EDGE_CURVE ( 'NONE', #12417, #12904, #1756, .T. ) ;
#2728=AXIS2_PLACEMENT_3D ( 'NONE', #2225, #14868, #27825 ) ;
#2736=DIRECTION ( 'NONE',  ( 0.000000000000000000, -0.000000000000000000, -1.000000000000000000 ) ) ;
#2737=EDGE_CURVE ( 'NONE', #5504, #27500, #14879, .T. ) ;
#2738=EDGE_LOOP ( 'NONE', ( #24640, #20713, #687, #12474 ) ) ;
#2743=AXIS2_PLACEMENT_3D ( 'NONE', #26516, #21579, #8482 ) ;
#2750=AXIS2_PLACEMENT_3D ( 'NONE', #4589, #14614, #21976 ) ;
#2757=AXIS2_PLACEMENT_3D ( 'NONE', #29874, #7390, #17384 ) ;
#2760=ADVANCED_FACE ( 'NONE', ( #30173 ), #14907, .F. ) ;
#2761=AXIS2_PLACEMENT_3D ( 'NONE', #6066, #31179, #31334 ) ;
#2763=EDGE_CURVE ( 'NONE', #2915, #32455, #17494, .T. ) ;
#2764=ORIENTED_EDGE ( 'NONE', *, *, #2763, .T. ) ;
#2767=EDGE_LOOP ( 'NONE', ( #14506, #267, #22597, #1671 ) ) ;
#2773=CIRCLE ( 'NONE', #30032, 12.36707279061065101 ) ;
#2778=ORIENTED_EDGE ( 'NONE', *, *, #15032, .F. ) ;
#2779=ORIENTED_EDGE ( 'NONE', *, *, #14759, .F. ) ;
#2785=LINE ( 'NONE', #15421, #22569 ) ;
#2786=DIRECTION ( 'NONE',  ( -1.000000000000000000, 0.000000000000000000, 0.000000000000000000 ) ) ;
#2792=TOROIDAL_SURFACE ( 'NONE', #20079, 12.40141737965285529, 0.1250000000000000555 ) ;
#2797=EDGE_CURVE ( 'NONE', #21972, #16102, #21675, .T. ) ;
#2799=AXIS2_PLACEMENT_3D ( 'NONE', #31420, #14187, #2026 ) ;
#2801=ORIENTED_EDGE ( 'NONE', *, *, #13825, .F. ) ;
#2802=ORIENTED_EDGE ( 'NONE', *, *, #4971, .T. ) ;
#2803=EDGE_CURVE ( 'NONE', #20430, #16795, #25880, .T. ) ;
#2811=EDGE_CURVE ( 'NONE', #2027, #26330, #3850, .T. ) ;
#2813=EDGE_CURVE ( 'NONE', #26531, #27840, #30084, .T. ) ;
#2818=CARTESIAN_POINT ( 'NONE',  ( 21.09992658989239089, 29.09164230456639899, 47.04930799450051637 ) ) ;
#2829=CARTESIAN_POINT ( 'NONE',  ( 33.72499318558949000, 38.56284415653841791, 47.04930799450051637 ) ) ;
#2836=CARTESIAN_POINT ( 'NONE',  ( 21.09992658989239089, 26.84143805560860940, 47.04930799450051637 ) ) ;
#2838=DIRECTION ( 'NONE',  ( -1.101824276508909887E-16, 1.000000000000000000, -0.000000000000000000 ) ) ;
#2843=ORIENTED_EDGE ( 'NONE', *, *, #18427, .F. ) ;
#2859=DIRECTION ( 'NONE',  ( -1.101824276508909887E-16, 1.000000000000000000, -0.000000000000000000 ) ) ;
#2860=FACE_OUTER_BOUND ( 'NONE', #25007, .T. ) ;
#2874=DIRECTION ( 'NONE',  ( -1.224646799147353207E-16, -1.349345573449484691E-32, 1.000000000000000000 ) ) ;
#2875=ORIENTED_EDGE ( 'NONE', *, *, #7120, .T. ) ;
#2883=AXIS2_PLACEMENT_3D ( 'NONE', #16494, #14042, #31765 ) ;
#2888=ADVANCED_FACE ( 'NONE', ( #15704 ), #27450, .T. ) ;
#2894=DIRECTION ( 'NONE',  ( -1.101824276508909887E-16, 1.000000000000000000, -0.000000000000000000 ) ) ;
#2895=CARTESIAN_POINT ( 'NONE',  ( 8.482002859293450214, 29.21664230456640254, 47.04930799450051637 ) ) ;
#2899=DIRECTION ( 'NONE',  ( 1.000000000000000000, 0.000000000000000000, 0.000000000000000000 ) ) ;
#2908=DIRECTION ( 'NONE',  ( -1.000000000000000000, 0.000000000000000000, 0.000000000000000000 ) ) ;
#2910=ORIENTED_EDGE ( 'NONE', *, *, #17751, .F. ) ;
#2911=CARTESIAN_POINT ( 'NONE',  ( 21.09992658989239089, 26.34143805560860940, 47.04930799450051637 ) ) ;
#2913=AXIS2_PLACEMENT_3D ( 'NONE', #230, #17624, #17784 ) ;
#2915=VERTEX_POINT ( 'NONE', #18638 ) ;
#2917=CARTESIAN_POINT ( 'NONE',  ( 21.09992658989238734, 38.56284415653841791, 47.04930799450051637 ) ) ;
#2919=ORIENTED_EDGE ( 'NONE', *, *, #12849, .T. ) ;
#2920=EDGE_LOOP ( 'NONE', ( #13323, #6461, #20434, #8177 ) ) ;
#2923=ORIENTED_EDGE ( 'NONE', *, *, #25215, .T. ) ;
#2925=ADVANCED_FACE ( 'NONE', ( #3388 ), #6177, .F. ) ;
#2927=CARTESIAN_POINT ( 'NONE',  ( 21.09992658989238734, 38.56284415653841791, 47.04930799450051637 ) ) ;
#2928=LINE ( 'NONE', #12960, #17990 ) ;
#2931=ORIENTED_EDGE ( 'NONE', *, *, #32403, .T. ) ;
#2933=DIRECTION ( 'NONE',  ( -1.101824276508909887E-16, 1.000000000000000000, -0.000000000000000000 ) ) ;
#2943=DIRECTION ( 'NONE',  ( -1.224646799147353207E-16, -1.349345573449484691E-32, 1.000000000000000000 ) ) ;
#2946=DIRECTION ( 'NONE',  ( 0.000000000000000000, -0.000000000000000000, -1.000000000000000000 ) ) ;
#2950=DIRECTION ( 'NONE',  ( -1.000000000000000000, 0.000000000000000000, 0.000000000000000000 ) ) ;
#2956=ORIENTED_EDGE ( 'NONE', *, *, #19881, .F. ) ;
#2958=DIRECTION ( 'NONE',  ( -1.000000000000000000, 0.000000000000000000, 0.000000000000000000 ) ) ;
#2959=CARTESIAN_POINT ( 'NONE',  ( 21.09992658989239089, 25.09184655352419213, 47.04930799450051637 ) ) ;
#2964=ADVANCED_FACE ( 'NONE', ( #21908 ), #1734, .F. ) ;
#2966=DIRECTION ( 'NONE',  ( -1.000000000000000000, 0.000000000000000000, 0.000000000000000000 ) ) ;
#2977=CARTESIAN_POINT ( 'NONE',  ( 21.09992658989239089, 26.09164230456639899, 47.04930799450051637 ) ) ;
#2978=TOROIDAL_SURFACE ( 'NONE', #1412, 12.61792373059897798, 0.1249999999999968636 ) ;
#2980=EDGE_LOOP ( 'NONE', ( #25527, #19797, #14227, #2141 ) ) ;
#2982=LINE ( 'NONE', #27947, #3798 ) ;
#2984=EDGE_CURVE ( 'NONE', #22139, #31904, #10708, .T. ) ;
#2987=DIRECTION ( 'NONE',  ( -1.101824276508909887E-16, 1.000000000000000000, -0.000000000000000000 ) ) ;
#2994=EDGE_CURVE ( 'NONE', #10069, #32344, #11592, .T. ) ;
#2995=EDGE_LOOP ( 'NONE', ( #31600, #19757, #7686, #16895 ) ) ;
#2996=ADVANCED_FACE ( 'NONE', ( #4522 ), #19055, .T. ) ;
#2998=DIRECTION ( 'NONE',  ( 0.000000000000000000, -0.000000000000000000, -1.000000000000000000 ) ) ;
#3001=CARTESIAN_POINT ( 'NONE',  ( 21.09992658989239089, 25.09164230456639899, 47.04930799450051637 ) ) ;
#3005=DIRECTION ( 'NONE',  ( -1.000000000000000000, 0.000000000000000000, 0.000000000000000000 ) ) ;
#3011=TOROIDAL_SURFACE ( 'NONE', #26582, 12.61792373059891226, 0.1250000000000024980 ) ;
#3012=DIRECTION ( 'NONE',  ( 0.000000000000000000, -0.000000000000000000, -1.000000000000000000 ) ) ;
#3014=CARTESIAN_POINT ( 'NONE',  ( 33.72499318558949710, 28.09184655352419213, 47.04930799450051637 ) ) ;
#3015=DIRECTION ( 'NONE',  ( -1.000000000000000000, -1.101824276508909887E-16, 0.000000000000000000 ) ) ;
#3017=ORIENTED_EDGE ( 'NONE', *, *, #1837, .F. ) ;
#3019=CARTESIAN_POINT ( 'NONE',  ( 21.09992658989239089, 25.84164230456639899, 47.04930799450051637 ) ) ;
#3020=CIRCLE ( 'NONE', #27138, 12.36707279061065101 ) ;
#3021=EDGE_CURVE ( 'NONE', #15217, #27344, #29039, .T. ) ;
#3024=DIRECTION ( 'NONE',  ( -1.101824276508909887E-16, 1.000000000000000000, -0.000000000000000000 ) ) ;
#3036=CIRCLE ( 'NONE', #25588, 0.1250000000000001110 ) ;
#3037=TOROIDAL_SURFACE ( 'NONE', #20331, 12.61792373059890693, 0.1250000000000019429 ) ;
#3046=CARTESIAN_POINT ( 'NONE',  ( 33.46699938050303302, 38.56284415653841791, 47.04930799450051637 ) ) ;
#3049=CARTESIAN_POINT ( 'NONE',  ( 21.09992658989239089, 26.84184655352419568, 47.04930799450051637 ) ) ;
#3053=ORIENTED_EDGE ( 'NONE', *, *, #5071, .T. ) ;
#3055=DIRECTION ( 'NONE',  ( -1.101824276508909887E-16, 1.000000000000000000, -0.000000000000000000 ) ) ;
#3059=DIRECTION ( 'NONE',  ( -1.000000000000000000, 0.000000000000000000, 0.000000000000000000 ) ) ;
#3061=ORIENTED_EDGE ( 'NONE', *, *, #10945, .T. ) ;
#3066=VERTEX_POINT ( 'NONE', #18955 ) ;
#3068=ORIENTED_EDGE ( 'NONE', *, *, #25059, .F. ) ;
#3069=DIRECTION ( 'NONE',  ( -1.000000000000000000, -1.101824276508910010E-16, 0.000000000000000000 ) ) ;
#3070=EDGE_CURVE ( 'NONE', #9009, #25296, #26523, .T. ) ;
#3088=ORIENTED_EDGE ( 'NONE', *, *, #28269, .T. ) ;
#3089=DIRECTION ( 'NONE',  ( -1.000000000000000000, 0.000000000000000000, 0.000000000000000000 ) ) ;
#3090=CARTESIAN_POINT ( 'NONE',  ( 21.09992658989238734, 32.34184655352418503, 47.04930799450051637 ) ) ;
#3091=CARTESIAN_POINT ( 'NONE',  ( 21.09992658989239089, 28.59164230456639544, 47.04930799450051637 ) ) ;
#3094=CYLINDRICAL_SURFACE ( 'NONE', #25774, 12.36707279061065101 ) ;
#3096=DIRECTION ( 'NONE',  ( -1.101824276508909887E-16, 1.000000000000000000, -0.000000000000000000 ) ) ;
#3097=DIRECTION ( 'NONE',  ( -1.101824276508909887E-16, 1.000000000000000000, -0.000000000000000000 ) ) ;
#3102=CYLINDRICAL_SURFACE ( 'NONE', #22976, 12.62506659569710266 ) ;
#3111=TOROIDAL_SURFACE ( 'NONE', #15197, 12.40141737965285706, 0.1250000000000007494 ) ;
#3113=VERTEX_POINT ( 'NONE', #19939 ) ;
#3117=DIRECTION ( 'NONE',  ( -1.101824276508909887E-16, 1.000000000000000000, -0.000000000000000000 ) ) ;
#3119=VERTEX_POINT ( 'NONE', #12410 ) ;
#3122=DIRECTION ( 'NONE',  ( -1.101824276508909887E-16, 1.000000000000000000, -0.000000000000000000 ) ) ;
#3123=DIRECTION ( 'NONE',  ( -1.101824276508909887E-16, 1.000000000000000000, -0.000000000000000000 ) ) ;
#3125=AXIS2_PLACEMENT_3D ( 'NONE', #29089, #6607, #16286 ) ;
#3128=CARTESIAN_POINT ( 'NONE',  ( 21.09992658989239089, 28.34164230456639544, 47.04930799450051637 ) ) ;
#3134=EDGE_CURVE ( 'NONE', #27738, #29931, #10692, .T. ) ;
#3135=DIRECTION ( 'NONE',  ( 1.000000000000000000, 0.000000000000000000, 0.000000000000000000 ) ) ;
#3138=VERTEX_POINT ( 'NONE', #12570 ) ;
#3139=DIRECTION ( 'NONE',  ( -1.000000000000000000, 0.000000000000000000, 0.000000000000000000 ) ) ;
#3140=AXIS2_PLACEMENT_3D ( 'NONE', #11063, #16290, #28937 ) ;
#3143=EDGE_LOOP ( 'NONE', ( #3357, #5469, #5179, #30796 ) ) ;
#3144=DIRECTION ( 'NONE',  ( -1.000000000000000000, 0.000000000000000000, 0.000000000000000000 ) ) ;
#3150=ADVANCED_FACE ( 'NONE', ( #17312 ), #16955, .T. ) ;
#3155=DIRECTION ( 'NONE',  ( -1.000000000000000000, 0.000000000000000000, 0.000000000000000000 ) ) ;
#3158=ORIENTED_EDGE ( 'NONE', *, *, #6146, .T. ) ;
#3160=CYLINDRICAL_SURFACE ( 'NONE', #25404, 12.62506659569710266 ) ;
#3166=EDGE_LOOP ( 'NONE', ( #30523, #4042, #31346, #7444 ) ) ;
#3167=CARTESIAN_POINT ( 'NONE',  ( 33.72499318558949710, 28.34143805560861296, 47.04930799450051637 ) ) ;
#3169=CARTESIAN_POINT ( 'NONE',  ( 33.72499318558949000, 38.56284415653841791, 47.04930799450051637 ) ) ;
#3170=LINE ( 'NONE', #17472, #23870 ) ;
#3172=EDGE_CURVE ( 'NONE', #25895, #7948, #8581, .T. ) ;
#3176=DIRECTION ( 'NONE',  ( -1.101824276508909887E-16, 1.000000000000000000, -0.000000000000000000 ) ) ;
#3184=DIRECTION ( 'NONE',  ( 0.000000000000000000, -0.000000000000000000, -1.000000000000000000 ) ) ;
#3186=DIRECTION ( 'NONE',  ( -1.000000000000000000, 0.000000000000000000, 0.000000000000000000 ) ) ;
#3187=AXIS2_PLACEMENT_3D ( 'NONE', #7480, #27159, #27498 ) ;
#3189=ORIENTED_EDGE ( 'NONE', *, *, #6713, .T. ) ;
#3194=AXIS2_PLACEMENT_3D ( 'NONE', #430, #10455, #23246 ) ;
#3201=CARTESIAN_POINT ( 'NONE',  ( 21.09992658989238734, 30.97145308207317171, 47.04930799450051637 ) ) ;
#3202=DIRECTION ( 'NONE',  ( -1.101824276508909887E-16, 1.000000000000000000, -0.000000000000000000 ) ) ;
#3203=CARTESIAN_POINT ( 'NONE',  ( 33.72499318558949000, 38.56284415653841791, 47.04930799450051637 ) ) ;
#3207=ORIENTED_EDGE ( 'NONE', *, *, #14170, .F. ) ;
#3213=DIRECTION ( 'NONE',  ( -1.000000000000000000, 0.000000000000000000, 0.000000000000000000 ) ) ;
#3214=CIRCLE ( 'NONE', #21551, 12.36707279061065279 ) ;
#3216=CLOSED_SHELL ( 'NONE', ( #5387, #22410, #23745, #26164, #7189, #23787, #4533, #20018, #1337, #8499, #20156, #26105, #21236, #5713, #23815, #26573, #30862, #630, #28094, #5545, #1438, #16925, #570, #12981, #24711, #23934, #7824, #30266, #7954, #10399, #9761, #28096, #17342, #31268, #16050, #29813, #3516, #18163, #31132, #22673, #7229, #14594, #29121, #11054, #19746, #20644, #3561, #24605, #3770, #13586, #6080, #6, #23904, #26608, #24436, #22049, #30282, #25126, #27081, #717, #20797, #16148, #6605, #11346, #3717, #10379, #11848, #9338, #13427, #7862, #27433, #3650, #21326, #9363, #26160, #672, #8933, #29983, #4866, #3479, #13432, #8625, #15674, #2925, #13083, #4943, #29953, #10649, #183, #29894, #14873, #28056, #28251, #32214, #26121, #10592, #28452, #28755, #26790, #26753, #6345, #3405, #21279, #31030, #28872, #299, #406, #25268, #21657, #14677, #9296, #14356, #6073, #9265, #17484, #20882, #12422, #4450, #25708, #28324, #995, #449, #28278, #28274, #16479, #13022, #27532, #26489, #22178, #11923, #28706, #2377, #5715, #12464, #27221, #12173, #1627, #19017, #26605, #23653, #23163, #11520, #24385, #10210, #334, #28485, #19245, #24194, #17333, #2964, #31749, #2308, #4863, #31388, #21272, #12659, #28203, #16586, #12956, #1107, #27713, #9857, #10092, #19614, #28796, #30660, #51, #12353, #3416, #6714, #6841, #19131, #17940, #28612, #13358, #14656, #8634, #31671, #18658, #29496, #9382, #15491, #14091, #6348, #2888, #27204, #24945, #1948, #25838, #129, #6673, #28236, #10084, #9123, #5636, #15705, #7642, #16781, #9016, #22292, #23445, #32401, #8181, #19254, #30307, #5718, #1381, #11349, #7543, #1996, #5276, #26304, #25971, #25500, #27879, #31586, #10004, #28396, #9788, #23678, #26571, #25970, #13138, #1253, #15395, #4825, #23992, #84, #23484, #13063, #14310, #22707, #8089, #7418, #19185, #8052, #6429, #28898, #14760, #17168, #27625, #25608, #8340, #6041, #23390, #14209, #13456, #23708, #23275, #15786, #5012, #14304, #25043, #16741, #9499, #16452, #6395, #28948, #27804, #12986, #29990, #10874, #14573, #19856, #13467, #18164, #24982, #7498, #5627, #10770, #18252, #5191, #8266, #5996, #9911, #9946, #20763, #4370, #12702, #30445, #21288, #6117, #21240, #18922, #21068, #26043, #28481, #1539, #23568, #20707, #4658, #24870, #14990, #5082, #24387, #13356, #1738, #10949, #950, #2996, #19420, #11843, #625, #9598, #28128, #12049, #31437, #25923, #130, #2070, #23002, #20758, #4215, #30670, #3591, #10353, #6572, #15125, #26496, #11974, #2760, #4414, #26080, #18010, #26269, #21386, #31548, #32215, #1171, #31309, #20057, #23058, #15013, #8010, #21430, #14083, #11818, #17449, #12871, #24401, #377, #16836, #13681, #24848, #220, #3150, #24380, #5319, #23571, #3300, #30399, #30831, #5758, #31214, #2258, #12949, #13186, #22562, #26604, #5794, #10352, #26201, #20928, #29721, #8656, #11087, #18025, #24717 ) ) ;
#3217=DIRECTION ( 'NONE',  ( -1.000000000000000000, 0.000000000000000000, 0.000000000000000000 ) ) ;
#3221=EDGE_CURVE ( 'NONE', #15469, #15557, #29007, .T. ) ;
#3226=CARTESIAN_POINT ( 'NONE',  ( 8.732853799281732776, 38.56284415653841791, 47.04930799450051637 ) ) ;
#3227=EDGE_CURVE ( 'NONE', #19822, #2124, #29561, .T. ) ;
#3228=FACE_OUTER_BOUND ( 'NONE', #21323, .T. ) ;
#3229=AXIS2_PLACEMENT_3D ( 'NONE', #23885, #4022, #11742 ) ;
#3231=CARTESIAN_POINT ( 'NONE',  ( 21.09992658989239089, 28.46664230456639899, 47.04930799450051637 ) ) ;
#3235=AXIS2_PLACEMENT_3D ( 'NONE', #20134, #5051, #21935 ) ;
#3243=AXIS2_PLACEMENT_3D ( 'NONE', #9141, #21766, #26376 ) ;
#3249=EDGE_CURVE ( 'NONE', #3066, #22635, #12794, .T. ) ;
#3254=CARTESIAN_POINT ( 'NONE',  ( 21.09992658989239089, 29.84184655352422411, 47.04930799450051637 ) ) ;
#3260=ORIENTED_EDGE ( 'NONE', *, *, #14759, .T. ) ;
#3261=CIRCLE ( 'NONE', #21596, 12.36707279061065279 ) ;
#3266=DIRECTION ( 'NONE',  ( -1.101824276508909887E-16, 1.000000000000000000, -0.000000000000000000 ) ) ;
#3270=DIRECTION ( 'NONE',  ( -1.101824276508909887E-16, 1.000000000000000000, -0.000000000000000000 ) ) ;
#3271=DIRECTION ( 'NONE',  ( -1.101824276508909887E-16, 1.000000000000000000, -0.000000000000000000 ) ) ;
#3274=ORIENTED_EDGE ( 'NONE', *, *, #26901, .T. ) ;
#3276=CARTESIAN_POINT ( 'NONE',  ( 33.72499318558949000, 38.56284415653841791, 47.04930799450051637 ) ) ;
#3277=EDGE_LOOP ( 'NONE', ( #21025, #10246, #22649, #9532 ) ) ;
#3278=CIRCLE ( 'NONE', #20052, 12.62506659569710266 ) ;
#3279=AXIS2_PLACEMENT_3D ( 'NONE', #1148, #31200, #18065 ) ;
#3286=CARTESIAN_POINT ( 'NONE',  ( 33.46699938050304013, 28.71183152705961206, 47.04930799450051637 ) ) ;
#3294=CARTESIAN_POINT ( 'NONE',  ( 21.09992658989239089, 27.46664230456639899, 47.04930799450051637 ) ) ;
#3295=CARTESIAN_POINT ( 'NONE',  ( 21.09992658989239089, 27.71183152705960850, 47.04930799450051637 ) ) ;
#3300=ADVANCED_FACE ( 'NONE', ( #8446 ), #32157, .T. ) ;
#3306=CARTESIAN_POINT ( 'NONE',  ( 8.474859994195286461, 30.09184655352422411, 47.04930799450051637 ) ) ;
#3308=DIRECTION ( 'NONE',  ( -1.101824276508909887E-16, 1.000000000000000000, -0.000000000000000000 ) ) ;
#3312=VECTOR ( 'NONE', #28867, 1000.000000000000000 ) ;
#3313=ORIENTED_EDGE ( 'NONE', *, *, #32207, .T. ) ;
#3320=TOROIDAL_SURFACE ( 'NONE', #31565, 12.40141737965284996, 0.1250000000000002776 ) ;
#3321=DIRECTION ( 'NONE',  ( -1.000000000000000000, 0.000000000000000000, 0.000000000000000000 ) ) ;
#3323=DIRECTION ( 'NONE',  ( -1.000000000000000000, 0.000000000000000000, 0.000000000000000000 ) ) ;
#3341=ORIENTED_EDGE ( 'NONE', *, *, #16604, .T. ) ;
#3343=CARTESIAN_POINT ( 'NONE',  ( 8.698509210239571132, 30.84164230456639544, 47.04930799450051637 ) ) ;
#3350=DIRECTION ( 'NONE',  ( -1.000000000000000000, 0.000000000000000000, 0.000000000000000000 ) ) ;
#3354=DIRECTION ( 'NONE',  ( -1.101824276508909887E-16, 1.000000000000000000, -0.000000000000000000 ) ) ;
#3357=ORIENTED_EDGE ( 'NONE', *, *, #30511, .F. ) ;
#3358=CARTESIAN_POINT ( 'NONE',  ( 8.732853799281734553, 38.56284415653841791, 47.04930799450051637 ) ) ;
#3369=VERTEX_POINT ( 'NONE', #15662 ) ;
#3372=FACE_OUTER_BOUND ( 'NONE', #28614, .T. ) ;
#3376=ORIENTED_EDGE ( 'NONE', *, *, #25213, .T. ) ;
#3380=CARTESIAN_POINT ( 'NONE',  ( 21.09992658989239089, 30.47145308207317882, 47.04930799450051637 ) ) ;
#3388=FACE_OUTER_BOUND ( 'NONE', #23219, .T. ) ;
#3389=VERTEX_POINT ( 'NONE', #30772 ) ;
#3391=FACE_OUTER_BOUND ( 'NONE', #18985, .T. ) ;
#3405=ADVANCED_FACE ( 'NONE', ( #6948 ), #11547, .F. ) ;
#3410=CIRCLE ( 'NONE', #12335, 12.36707279061065101 ) ;
#3416=ADVANCED_FACE ( 'NONE', ( #2018 ), #26377, .T. ) ;
#3427=ORIENTED_EDGE ( 'NONE', *, *, #16067, .F. ) ;
#3428=DIRECTION ( 'NONE',  ( -1.000000000000000000, 0.000000000000000000, 0.000000000000000000 ) ) ;
#3429=FACE_OUTER_BOUND ( 'NONE', #7693, .T. ) ;
#3430=DIRECTION ( 'NONE',  ( 0.000000000000000000, -0.000000000000000000, -1.000000000000000000 ) ) ;
#3433=EDGE_CURVE ( 'NONE', #18578, #20832, #31415, .T. ) ;
#3444=VERTEX_POINT ( 'NONE', #6783 ) ;
#3447=DIRECTION ( 'NONE',  ( -1.101824276508909887E-16, 1.000000000000000000, -0.000000000000000000 ) ) ;
#3460=CARTESIAN_POINT ( 'NONE',  ( 33.50134396954526039, 25.59164230456639899, 47.04930799450051637 ) ) ;
#3467=CYLINDRICAL_SURFACE ( 'NONE', #16188, 12.36707279061065101 ) ;
#3469=ORIENTED_EDGE ( 'NONE', *, *, #6527, .F. ) ;
#3471=FACE_OUTER_BOUND ( 'NONE', #4263, .T. ) ;
#3472=ORIENTED_EDGE ( 'NONE', *, *, #28398, .T. ) ;
#3478=ORIENTED_EDGE ( 'NONE', *, *, #24071, .F. ) ;
#3479=ADVANCED_FACE ( 'NONE', ( #18752 ), #16304, .F. ) ;
#3481=AXIS2_PLACEMENT_3D ( 'NONE', #10835, #30852, #3428 ) ;
#3483=VERTEX_POINT ( 'NONE', #19076 ) ;
#3487=AXIS2_PLACEMENT_3D ( 'NONE', #20010, #12151, #7709 ) ;
#3495=ORIENTED_EDGE ( 'NONE', *, *, #7611, .F. ) ;
#3496=DIRECTION ( 'NONE',  ( -1.101824276508909887E-16, 1.000000000000000000, -0.000000000000000000 ) ) ;
#3502=CARTESIAN_POINT ( 'NONE',  ( 21.09992658989239089, 27.09143805560860940, 47.04930799450051637 ) ) ;
#3503=CARTESIAN_POINT ( 'NONE',  ( 21.09992658989238734, 38.56284415653841791, 47.04930799450051637 ) ) ;
#3504=CARTESIAN_POINT ( 'NONE',  ( 21.09992658989239089, 24.21183152705959785, 47.04930799450051637 ) ) ;
#3508=AXIS2_PLACEMENT_3D ( 'NONE', #7108, #11871, #4484 ) ;
#3513=ORIENTED_EDGE ( 'NONE', *, *, #25758, .T. ) ;
#3516=ADVANCED_FACE ( 'NONE', ( #14340 ), #2089, .T. ) ;
#3523=CARTESIAN_POINT ( 'NONE',  ( 33.46699938050304013, 28.22145308207318237, 47.04930799450050927 ) ) ;
#3524=FACE_OUTER_BOUND ( 'NONE', #14074, .T. ) ;
#3527=ORIENTED_EDGE ( 'NONE', *, *, #27906, .T. ) ;
#3533=CIRCLE ( 'NONE', #26076, 12.62506659569710443 ) ;
#3534=DIRECTION ( 'NONE',  ( -1.101824276508909887E-16, 1.000000000000000000, -0.000000000000000000 ) ) ;
#3535=ORIENTED_EDGE ( 'NONE', *, *, #30269, .F. ) ;
#3537=ORIENTED_EDGE ( 'NONE', *, *, #24064, .F. ) ;
#3543=CIRCLE ( 'NONE', #21348, 0.1250000000000001110 ) ;
#3546=ORIENTED_EDGE ( 'NONE', *, *, #16556, .T. ) ;
#3547=CARTESIAN_POINT ( 'NONE',  ( 21.09992658989238734, 30.71183152705961916, 47.04930799450051637 ) ) ;
#3551=EDGE_CURVE ( 'NONE', #2570, #29229, #21449, .T. ) ;
#3554=VERTEX_POINT ( 'NONE', #19901 ) ;
#3559=VERTEX_POINT ( 'NONE', #10230 ) ;
#3561=ADVANCED_FACE ( 'NONE', ( #9901 ), #14143, .T. ) ;
#3567=CARTESIAN_POINT ( 'NONE',  ( 21.09992658989239089, 27.59164230456639544, 47.04930799450051637 ) ) ;
#3569=EDGE_CURVE ( 'NONE', #29858, #2915, #25326, .T. ) ;
#3572=VECTOR ( 'NONE', #23189, 1000.000000000000000 ) ;
#3580=FACE_OUTER_BOUND ( 'NONE', #11296, .T. ) ;
#3589=EDGE_CURVE ( 'NONE', #4416, #28214, #7280, .T. ) ;
#3591=ADVANCED_FACE ( 'NONE', ( #27785 ), #12707, .F. ) ;
#3592=AXIS2_PLACEMENT_3D ( 'NONE', #8090, #12855, #17925 ) ;
#3594=CYLINDRICAL_SURFACE ( 'NONE', #27750, 12.62506659569710266 ) ;
#3595=CARTESIAN_POINT ( 'NONE',  ( 21.09992658989238734, 38.56284415653841791, 47.04930799450051637 ) ) ;
#3598=DIRECTION ( 'NONE',  ( -1.101824276508909887E-16, 1.000000000000000000, -0.000000000000000000 ) ) ;
#3599=ORIENTED_EDGE ( 'NONE', *, *, #19250, .F. ) ;
#3605=ORIENTED_EDGE ( 'NONE', *, *, #22293, .F. ) ;
#3607=CARTESIAN_POINT ( 'NONE',  ( 21.09992658989239089, 24.34143805560860940, 47.04930799450051637 ) ) ;
#3608=DIRECTION ( 'NONE',  ( -1.000000000000000000, 0.000000000000000000, 0.000000000000000000 ) ) ;
#3612=DIRECTION ( 'NONE',  ( -1.101824276508909887E-16, 1.000000000000000000, -0.000000000000000000 ) ) ;
#3616=CARTESIAN_POINT ( 'NONE',  ( 21.09992658989238734, 38.56284415653841791, 47.04930799450051637 ) ) ;
#3617=ORIENTED_EDGE ( 'NONE', *, *, #4028, .T. ) ;
#3627=AXIS2_PLACEMENT_3D ( 'NONE', #30311, #27846, #22258 ) ;
#3628=DIRECTION ( 'NONE',  ( 0.000000000000000000, -0.000000000000000000, -1.000000000000000000 ) ) ;
#3633=ORIENTED_EDGE ( 'NONE', *, *, #5533, .T. ) ;
#3634=DIRECTION ( 'NONE',  ( -1.000000000000000000, -1.101824276508909887E-16, 0.000000000000000000 ) ) ;
#3639=AXIS2_PLACEMENT_3D ( 'NONE', #11718, #21544, #23859 ) ;
#3643=CYLINDRICAL_SURFACE ( 'NONE', #21914, 12.36707279061065101 ) ;
#3646=AXIS2_PLACEMENT_3D ( 'NONE', #14142, #1980, #27092 ) ;
#3650=ADVANCED_FACE ( 'NONE', ( #30253 ), #6265, .T. ) ;
#3653=ORIENTED_EDGE ( 'NONE', *, *, #429, .T. ) ;
#3655=DIRECTION ( 'NONE',  ( -1.000000000000000000, 0.000000000000000000, 0.000000000000000000 ) ) ;
#3657=CIRCLE ( 'NONE', #19947, 12.36707279061065101 ) ;
#3659=AXIS2_PLACEMENT_3D ( 'NONE', #20627, #13096, #8164 ) ;
#3662=AXIS2_PLACEMENT_3D ( 'NONE', #736, #2714, #20752 ) ;
#3663=CARTESIAN_POINT ( 'NONE',  ( 8.732853799281734553, 38.56284415653841791, 47.04930799450051637 ) ) ;
#3665=DIRECTION ( 'NONE',  ( -1.101824276508909887E-16, 1.000000000000000000, -0.000000000000000000 ) ) ;
#3669=ORIENTED_EDGE ( 'NONE', *, *, #371, .T. ) ;
#3677=DIRECTION ( 'NONE',  ( -1.101824276508909887E-16, 1.000000000000000000, -0.000000000000000000 ) ) ;
#3683=AXIS2_PLACEMENT_3D ( 'NONE', #24617, #21661, #27237 ) ;
#3687=TOROIDAL_SURFACE ( 'NONE', #25729, 12.40141737965283930, 0.1250000000000007216 ) ;
#3694=VERTEX_POINT ( 'NONE', #20712 ) ;
#3695=DIRECTION ( 'NONE',  ( -1.000000000000000000, 0.000000000000000000, 0.000000000000000000 ) ) ;
#3696=DIRECTION ( 'NONE',  ( -1.101824276508909887E-16, 1.000000000000000000, -0.000000000000000000 ) ) ;
#3699=CARTESIAN_POINT ( 'NONE',  ( 8.698509210239565803, 29.84164230456639899, 47.04930799450051637 ) ) ;
#3705=AXIS2_PLACEMENT_3D ( 'NONE', #5534, #5694, #12772 ) ;
#3706=FACE_OUTER_BOUND ( 'NONE', #6938, .T. ) ;
#3707=DIRECTION ( 'NONE',  ( -1.101824276508909887E-16, 1.000000000000000000, -0.000000000000000000 ) ) ;
#3708=DIRECTION ( 'NONE',  ( -1.000000000000000000, -1.101824276508910010E-16, 0.000000000000000000 ) ) ;
#3714=AXIS2_PLACEMENT_3D ( 'NONE', #23451, #28545, #20981 ) ;
#3715=DIRECTION ( 'NONE',  ( -1.000000000000000000, 0.000000000000000000, 0.000000000000000000 ) ) ;
#3717=ADVANCED_FACE ( 'NONE', ( #3471 ), #3111, .T. ) ;
#3718=ORIENTED_EDGE ( 'NONE', *, *, #28578, .T. ) ;
#3723=VERTEX_POINT ( 'NONE', #694 ) ;
#3725=CIRCLE ( 'NONE', #11093, 12.27641737965286239 ) ;
#3729=AXIS2_PLACEMENT_3D ( 'NONE', #12399, #17471, #15020 ) ;
#3733=DIRECTION ( 'NONE',  ( 1.000000000000000000, 0.000000000000000000, 0.000000000000000000 ) ) ;
#3734=DIRECTION ( 'NONE',  ( -1.101824276508909887E-16, 1.000000000000000000, -0.000000000000000000 ) ) ;
#3746=EDGE_CURVE ( 'NONE', #21198, #15433, #6100, .T. ) ;
#3749=DIRECTION ( 'NONE',  ( -1.101824276508909887E-16, 1.000000000000000000, -0.000000000000000000 ) ) ;
#3751=ORIENTED_EDGE ( 'NONE', *, *, #11564, .T. ) ;
#3752=DIRECTION ( 'NONE',  ( -1.101824276508909887E-16, 1.000000000000000000, -0.000000000000000000 ) ) ;
#3757=DIRECTION ( 'NONE',  ( -1.000000000000000000, 0.000000000000000000, 0.000000000000000000 ) ) ;
#3763=DIRECTION ( 'NONE',  ( -1.000000000000000000, 0.000000000000000000, 0.000000000000000000 ) ) ;
#3770=ADVANCED_FACE ( 'NONE', ( #28742 ), #12580, .T. ) ;
#3776=ORIENTED_EDGE ( 'NONE', *, *, #19702, .F. ) ;
#3777=CARTESIAN_POINT ( 'NONE',  ( 33.72499318558949000, 38.56284415653841791, 47.04930799450051637 ) ) ;
#3782=EDGE_CURVE ( 'NONE', #14790, #23072, #11508, .T. ) ;
#3787=DIRECTION ( 'NONE',  ( -1.000000000000000000, -1.101824276508909887E-16, 0.000000000000000000 ) ) ;
#3788=CARTESIAN_POINT ( 'NONE',  ( 21.09992658989239089, 30.21183152705961561, 47.04930799450051637 ) ) ;
#3793=ORIENTED_EDGE ( 'NONE', *, *, #25292, .F. ) ;
#3798=VECTOR ( 'NONE', #11155, 1000.000000000000000 ) ;
#3799=EDGE_CURVE ( 'NONE', #26085, #8602, #29337, .T. ) ;
#3803=CARTESIAN_POINT ( 'NONE',  ( 21.09992658989239089, 30.09143805560860585, 47.04930799450051637 ) ) ;
#3805=DIRECTION ( 'NONE',  ( 1.000000000000000000, 0.000000000000000000, 0.000000000000000000 ) ) ;
#3807=EDGE_CURVE ( 'NONE', #22296, #20658, #11678, .T. ) ;
#3810=AXIS2_PLACEMENT_3D ( 'NONE', #3091, #13131, #645 ) ;
#3827=FACE_OUTER_BOUND ( 'NONE', #4604, .T. ) ;
#3829=DIRECTION ( 'NONE',  ( -1.101824276508909887E-16, 1.000000000000000000, -0.000000000000000000 ) ) ;
#3831=DIRECTION ( 'NONE',  ( -1.000000000000000000, 0.000000000000000000, 0.000000000000000000 ) ) ;
#3835=CARTESIAN_POINT ( 'NONE',  ( 21.09992658989239089, 24.59164230456639544, 47.04930799450051637 ) ) ;
#3836=FACE_OUTER_BOUND ( 'NONE', #5344, .T. ) ;
#3838=DIRECTION ( 'NONE',  ( -1.000000000000000000, 0.000000000000000000, 0.000000000000000000 ) ) ;
#3840=VERTEX_POINT ( 'NONE', #2149 ) ;
#3846=EDGE_CURVE ( 'NONE', #10801, #17800, #22516, .T. ) ;
#3849=TOROIDAL_SURFACE ( 'NONE', #2799, 12.40141737965280733, 0.1250000000000013878 ) ;
#3850=CIRCLE ( 'NONE', #22186, 12.27641737965281621 ) ;
#3851=EDGE_CURVE ( 'NONE', #9420, #893, #4775, .T. ) ;
#3852=EDGE_CURVE ( 'NONE', #7282, #1140, #1061, .T. ) ;
#3855=DIRECTION ( 'NONE',  ( -1.101824276508909887E-16, 1.000000000000000000, -0.000000000000000000 ) ) ;
#3856=AXIS2_PLACEMENT_3D ( 'NONE', #13829, #19048, #21514 ) ;
#3861=DIRECTION ( 'NONE',  ( -1.000000000000000000, 0.000000000000000000, 0.000000000000000000 ) ) ;
#3863=DIRECTION ( 'NONE',  ( -1.101824276508909887E-16, 1.000000000000000000, -0.000000000000000000 ) ) ;
#3865=CARTESIAN_POINT ( 'NONE',  ( 8.732853799281738105, 28.46183152705961206, 47.04930799450051637 ) ) ;
#3866=CARTESIAN_POINT ( 'NONE',  ( 8.732853799281732776, 29.47145308207317527, 47.04930799450051637 ) ) ;
#3867=CARTESIAN_POINT ( 'NONE',  ( 21.09992658989239089, 24.96183152705960140, 47.04930799450051637 ) ) ;
#3875=ORIENTED_EDGE ( 'NONE', *, *, #28499, .T. ) ;
#3879=FACE_OUTER_BOUND ( 'NONE', #2224, .T. ) ;
#3884=ORIENTED_EDGE ( 'NONE', *, *, #24193, .F. ) ;
#3901=ORIENTED_EDGE ( 'NONE', *, *, #30886, .F. ) ;
#3902=DIRECTION ( 'NONE',  ( 1.000000000000000000, 0.000000000000000000, 0.000000000000000000 ) ) ;
#3905=DIRECTION ( 'NONE',  ( 0.000000000000000000, -0.000000000000000000, -1.000000000000000000 ) ) ;
#3912=VERTEX_POINT ( 'NONE', #10981 ) ;
#3921=ORIENTED_EDGE ( 'NONE', *, *, #5538, .T. ) ;
#3925=FACE_OUTER_BOUND ( 'NONE', #31699, .T. ) ;
#3926=ORIENTED_EDGE ( 'NONE', *, *, #17786, .F. ) ;
#3930=AXIS2_PLACEMENT_3D ( 'NONE', #12303, #17542, #27561 ) ;
#3936=DIRECTION ( 'NONE',  ( -1.101824276508909887E-16, 1.000000000000000000, -0.000000000000000000 ) ) ;
#3938=CIRCLE ( 'NONE', #14960, 12.27641737965287305 ) ;
#3939=CYLINDRICAL_SURFACE ( 'NONE', #6830, 12.62506659569710266 ) ;
#3940=CIRCLE ( 'NONE', #16002, 12.36707279061065101 ) ;
#3946=EDGE_LOOP ( 'NONE', ( #32120, #21776, #17000, #11287 ) ) ;
#3947=DIRECTION ( 'NONE',  ( -1.101824276508909887E-16, 1.000000000000000000, -0.000000000000000000 ) ) ;
#3954=DIRECTION ( 'NONE',  ( -1.000000000000000000, 0.000000000000000000, 0.000000000000000000 ) ) ;
#3955=CARTESIAN_POINT ( 'NONE',  ( 21.09992658989239089, 24.34164230456639544, 47.04930799450051637 ) ) ;
#3964=VECTOR ( 'NONE', #7440, 1000.000000000000000 ) ;
#3966=CARTESIAN_POINT ( 'NONE',  ( 21.09992658989238734, 38.56284415653841791, 47.04930799450051637 ) ) ;
#3967=CIRCLE ( 'NONE', #1335, 0.1250000000000001110 ) ;
#3968=VERTEX_POINT ( 'NONE', #8353 ) ;
#3969=CARTESIAN_POINT ( 'NONE',  ( 21.09992658989239089, 24.47145308207319303, 47.04930799450051637 ) ) ;
#3972=DIRECTION ( 'NONE',  ( -1.000000000000000000, 0.000000000000000000, 0.000000000000000000 ) ) ;
#3976=CARTESIAN_POINT ( 'NONE',  ( 33.46699938050304013, 26.71183152705960495, 47.04930799450051637 ) ) ;
#3980=DIRECTION ( 'NONE',  ( -1.101824276508909887E-16, 1.000000000000000000, -0.000000000000000000 ) ) ;
#3981=CARTESIAN_POINT ( 'NONE',  ( 8.732853799281734553, 38.56284415653841791, 47.04930799450051637 ) ) ;
#3995=DIRECTION ( 'NONE',  ( -1.000000000000000000, 0.000000000000000000, 0.000000000000000000 ) ) ;
#3996=EDGE_LOOP ( 'NONE', ( #6785, #27567, #29701, #28632 ) ) ;
#3997=DIRECTION ( 'NONE',  ( -1.000000000000000000, 0.000000000000000000, 0.000000000000000000 ) ) ;
#4003=EDGE_LOOP ( 'NONE', ( #6018, #29108, #2802, #29688 ) ) ;
#4009=EDGE_CURVE ( 'NONE', #11017, #22098, #7346, .T. ) ;
#4012=DIRECTION ( 'NONE',  ( -1.000000000000000000, 0.000000000000000000, 0.000000000000000000 ) ) ;
#4017=FACE_OUTER_BOUND ( 'NONE', #22898, .T. ) ;
#4018=EDGE_CURVE ( 'NONE', #2537, #17110, #20459, .T. ) ;
#4021=DIRECTION ( 'NONE',  ( -1.000000000000000000, 0.000000000000000000, 0.000000000000000000 ) ) ;
#4022=DIRECTION ( 'NONE',  ( -1.101824276508909887E-16, 1.000000000000000000, -0.000000000000000000 ) ) ;
#4023=DIRECTION ( 'NONE',  ( -1.101824276508909887E-16, 1.000000000000000000, -0.000000000000000000 ) ) ;
#4028=EDGE_CURVE ( 'NONE', #9505, #19596, #19390, .T. ) ;
#4031=CARTESIAN_POINT ( 'NONE',  ( 33.50134396954525329, 26.34164230456639899, 47.04930799450051637 ) ) ;
#4033=ORIENTED_EDGE ( 'NONE', *, *, #11886, .T. ) ;
#4034=CARTESIAN_POINT ( 'NONE',  ( 21.09992658989239089, 24.09164230456639544, 47.04930799450051637 ) ) ;
#4042=ORIENTED_EDGE ( 'NONE', *, *, #1385, .F. ) ;
#4044=AXIS2_PLACEMENT_3D ( 'NONE', #26598, #8880, #6741 ) ;
#4049=CARTESIAN_POINT ( 'NONE',  ( 21.09992658989238734, 38.56284415653841791, 47.04930799450051637 ) ) ;
#4056=DIRECTION ( 'NONE',  ( -1.101824276508909887E-16, 1.000000000000000000, -0.000000000000000000 ) ) ;
#4057=ORIENTED_EDGE ( 'NONE', *, *, #16753, .F. ) ;
#4074=DIRECTION ( 'NONE',  ( -1.101824276508909887E-16, 1.000000000000000000, -0.000000000000000000 ) ) ;
#4075=ORIENTED_EDGE ( 'NONE', *, *, #9216, .F. ) ;
#4079=FACE_OUTER_BOUND ( 'NONE', #31918, .T. ) ;
#4082=ORIENTED_EDGE ( 'NONE', *, *, #11049, .F. ) ;
#4085=CIRCLE ( 'NONE', #27700, 12.62506659569710266 ) ;
#4092=CIRCLE ( 'NONE', #13044, 12.36707279061065101 ) ;
#4097=AXIS2_PLACEMENT_3D ( 'NONE', #11526, #21522, #29581 ) ;
#4104=DIRECTION ( 'NONE',  ( -1.101824276508909887E-16, 1.000000000000000000, -0.000000000000000000 ) ) ;
#4106=EDGE_CURVE ( 'NONE', #29845, #14608, #27798, .T. ) ;
#4109=EDGE_CURVE ( 'NONE', #14664, #32344, #24650, .T. ) ;
#4110=EDGE_CURVE ( 'NONE', #10069, #13562, #28321, .T. ) ;
#4118=DIRECTION ( 'NONE',  ( -1.224646799147353207E-16, -1.349345573449484691E-32, 1.000000000000000000 ) ) ;
#4119=AXIS2_PLACEMENT_3D ( 'NONE', #23476, #15771, #21316 ) ;
#4122=AXIS2_PLACEMENT_3D ( 'NONE', #28429, #6255, #3787 ) ;
#4133=EDGE_CURVE ( 'NONE', #5692, #12300, #5781, .T. ) ;
#4136=CIRCLE ( 'NONE', #31269, 12.27641737965282687 ) ;
#4137=DIRECTION ( 'NONE',  ( -1.101824276508909887E-16, 1.000000000000000000, -0.000000000000000000 ) ) ;
#4143=ORIENTED_EDGE ( 'NONE', *, *, #2721, .T. ) ;
#4144=CYLINDRICAL_SURFACE ( 'NONE', #10283, 12.62506659569710266 ) ;
#4147=VECTOR ( 'NONE', #27086, 1000.000000000000000 ) ;
#4148=DIRECTION ( 'NONE',  ( -1.000000000000000000, 0.000000000000000000, 0.000000000000000000 ) ) ;
#4156=DIRECTION ( 'NONE',  ( -1.224646799147353207E-16, -1.349345573449484691E-32, 1.000000000000000000 ) ) ;
#4157=EDGE_CURVE ( 'NONE', #11938, #12012, #2639, .T. ) ;
#4158=CARTESIAN_POINT ( 'NONE',  ( 21.09992658989239089, 27.84164230456639544, 47.04930799450051637 ) ) ;
#4159=DIRECTION ( 'NONE',  ( -1.000000000000000000, 0.000000000000000000, 0.000000000000000000 ) ) ;
#4160=FACE_OUTER_BOUND ( 'NONE', #14723, .T. ) ;
#4169=AXIS2_PLACEMENT_3D ( 'NONE', #24838, #30097, #27128 ) ;
#4171=TOROIDAL_SURFACE ( 'NONE', #15200, 12.40141737965284463, 0.1250000000000005274 ) ;
#4172=FACE_OUTER_BOUND ( 'NONE', #7776, .T. ) ;
#4175=CIRCLE ( 'NONE', #3662, 12.62506659569710266 ) ;
#4187=CARTESIAN_POINT ( 'NONE',  ( 21.09992658989239089, 30.09143805560860585, 47.04930799450051637 ) ) ;
#4191=AXIS2_PLACEMENT_3D ( 'NONE', #17329, #28132, #15813 ) ;
#4197=DIRECTION ( 'NONE',  ( -1.000000000000000000, 0.000000000000000000, 0.000000000000000000 ) ) ;
#4201=ORIENTED_EDGE ( 'NONE', *, *, #20155, .T. ) ;
#4202=EDGE_CURVE ( 'NONE', #16708, #2250, #10489, .T. ) ;
#4210=CIRCLE ( 'NONE', #22542, 0.1249999999999966416 ) ;
#4213=EDGE_CURVE ( 'NONE', #26728, #28996, #20961, .T. ) ;
#4215=ADVANCED_FACE ( 'NONE', ( #12442 ), #6863, .F. ) ;
#4217=EDGE_CURVE ( 'NONE', #1940, #28369, #517, .T. ) ;
#4220=DIRECTION ( 'NONE',  ( -1.101824276508909887E-16, 1.000000000000000000, -0.000000000000000000 ) ) ;
#4228=CIRCLE ( 'NONE', #17243, 0.1250000000000001110 ) ;
#4231=ORIENTED_EDGE ( 'NONE', *, *, #30871, .F. ) ;
#4232=CARTESIAN_POINT ( 'NONE',  ( 21.09992658989238734, 31.71664230456639544, 47.04930799450051637 ) ) ;
#4233=ORIENTED_EDGE ( 'NONE', *, *, #6806, .F. ) ;
#4235=DIRECTION ( 'NONE',  ( -1.000000000000000000, 0.000000000000000000, 0.000000000000000000 ) ) ;
#4242=ORIENTED_EDGE ( 'NONE', *, *, #18829, .F. ) ;
#4243=DIRECTION ( 'NONE',  ( -1.101824276508909887E-16, 1.000000000000000000, -0.000000000000000000 ) ) ;
#4245=CIRCLE ( 'NONE', #25216, 0.1250000000000001110 ) ;
#4248=ORIENTED_EDGE ( 'NONE', *, *, #25645, .F. ) ;
#4263=EDGE_LOOP ( 'NONE', ( #12466, #5613, #11706, #20959 ) ) ;
#4267=DIRECTION ( 'NONE',  ( -1.101824276508909887E-16, 1.000000000000000000, -0.000000000000000000 ) ) ;
#4270=VERTEX_POINT ( 'NONE', #15539 ) ;
#4271=CIRCLE ( 'NONE', #7967, 0.1250000000000018319 ) ;
#4273=DIRECTION ( 'NONE',  ( -1.101824276508909887E-16, 1.000000000000000000, -0.000000000000000000 ) ) ;
#4274=CIRCLE ( 'NONE', #28392, 12.36707279061065279 ) ;
#4275=DIRECTION ( 'NONE',  ( -1.101824276508909887E-16, 1.000000000000000000, -0.000000000000000000 ) ) ;
#4279=ORIENTED_EDGE ( 'NONE', *, *, #583, .T. ) ;
#4286=ORIENTED_EDGE ( 'NONE', *, *, #11091, .F. ) ;
#4288=DIRECTION ( 'NONE',  ( -1.101824276508909887E-16, 1.000000000000000000, -0.000000000000000000 ) ) ;
#4291=EDGE_LOOP ( 'NONE', ( #12065, #32115, #13056, #24213 ) ) ;
#4293=VECTOR ( 'NONE', #23197, 1000.000000000000000 ) ;
#4294=DIRECTION ( 'NONE',  ( -1.000000000000000000, 0.000000000000000000, 0.000000000000000000 ) ) ;
#4301=EDGE_CURVE ( 'NONE', #23854, #28828, #13144, .T. ) ;
#4308=DIRECTION ( 'NONE',  ( -1.101824276508909887E-16, 1.000000000000000000, -0.000000000000000000 ) ) ;
#4313=ORIENTED_EDGE ( 'NONE', *, *, #4109, .T. ) ;
#4314=DIRECTION ( 'NONE',  ( -1.000000000000000000, 0.000000000000000000, 0.000000000000000000 ) ) ;
#4327=AXIS2_PLACEMENT_3D ( 'NONE', #2386, #7142, #7307 ) ;
#4333=ORIENTED_EDGE ( 'NONE', *, *, #3746, .T. ) ;
#4334=EDGE_CURVE ( 'NONE', #29845, #29925, #24684, .T. ) ;
#4337=VECTOR ( 'NONE', #8384, 1000.000000000000000 ) ;
#4342=AXIS2_PLACEMENT_3D ( 'NONE', #9129, #1901, #11912 ) ;
#4344=CYLINDRICAL_SURFACE ( 'NONE', #30292, 12.62506659569710266 ) ;
#4345=DIRECTION ( 'NONE',  ( -1.000000000000000000, -1.101824276508909887E-16, 0.000000000000000000 ) ) ;
#4350=FACE_OUTER_BOUND ( 'NONE', #5588, .T. ) ;
#4353=ORIENTED_EDGE ( 'NONE', *, *, #18364, .F. ) ;
#4357=CARTESIAN_POINT ( 'NONE',  ( 33.50134396954520355, 30.84164230456639544, 47.04930799450051637 ) ) ;
#4358=DIRECTION ( 'NONE',  ( -1.000000000000000000, -1.101824276508909887E-16, 0.000000000000000000 ) ) ;
#4361=ORIENTED_EDGE ( 'NONE', *, *, #23247, .T. ) ;
#4362=DIRECTION ( 'NONE',  ( -1.101824276508909887E-16, 1.000000000000000000, -0.000000000000000000 ) ) ;
#4366=DIRECTION ( 'NONE',  ( -1.224646799147353207E-16, -1.349345573449484691E-32, 1.000000000000000000 ) ) ;
#4367=ORIENTED_EDGE ( 'NONE', *, *, #8099, .T. ) ;
#4368=AXIS2_PLACEMENT_3D ( 'NONE', #12576, #3677, #8135 ) ;
#4369=ORIENTED_EDGE ( 'NONE', *, *, #11634, .F. ) ;
#4370=ADVANCED_FACE ( 'NONE', ( #7681 ), #23627, .T. ) ;
#4371=EDGE_CURVE ( 'NONE', #154, #7848, #7372, .T. ) ;
#4373=TOROIDAL_SURFACE ( 'NONE', #13306, 12.40141737965284996, 0.1250000000000002776 ) ;
#4381=CARTESIAN_POINT ( 'NONE',  ( 33.37634396954523908, 27.84164230456639544, 47.04930799450051637 ) ) ;
#4384=EDGE_LOOP ( 'NONE', ( #865, #24429, #25277, #4233 ) ) ;
#4391=DIRECTION ( 'NONE',  ( -1.000000000000000000, 0.000000000000000000, 0.000000000000000000 ) ) ;
#4392=CARTESIAN_POINT ( 'NONE',  ( 33.46699938050304013, 30.96183152705961206, 47.04930799450051637 ) ) ;
#4395=AXIS2_PLACEMENT_3D ( 'NONE', #14861, #24867, #9606 ) ;
#4398=EDGE_CURVE ( 'NONE', #24757, #20619, #10538, .T. ) ;
#4400=DIRECTION ( 'NONE',  ( -1.000000000000000000, -1.101824276508909887E-16, 0.000000000000000000 ) ) ;
#4402=DIRECTION ( 'NONE',  ( -1.000000000000000000, -1.101824276508909764E-16, 0.000000000000000000 ) ) ;
#4405=DIRECTION ( 'NONE',  ( -1.000000000000000000, -1.101824276508909887E-16, 0.000000000000000000 ) ) ;
#4411=CARTESIAN_POINT ( 'NONE',  ( 8.698509210239528500, 26.34164230456639899, 47.04930799450051637 ) ) ;
#4414=ADVANCED_FACE ( 'NONE', ( #3706 ), #30971, .T. ) ;
#4416=VERTEX_POINT ( 'NONE', #6170 ) ;
#4417=DIRECTION ( 'NONE',  ( -1.101824276508909887E-16, 1.000000000000000000, -0.000000000000000000 ) ) ;
#4418=EDGE_CURVE ( 'NONE', #27343, #4474, #20481, .T. ) ;
#4419=DIRECTION ( 'NONE',  ( 0.000000000000000000, -0.000000000000000000, -1.000000000000000000 ) ) ;
#4420=DIRECTION ( 'NONE',  ( -1.000000000000000000, 0.000000000000000000, 0.000000000000000000 ) ) ;
#4423=FACE_OUTER_BOUND ( 'NONE', #31942, .T. ) ;
#4425=CARTESIAN_POINT ( 'NONE',  ( 8.698509210239553369, 28.59164230456639544, 47.04930799450051637 ) ) ;
#4427=TOROIDAL_SURFACE ( 'NONE', #236, 12.40141737965280733, 0.1250000000000013878 ) ;
#4428=ORIENTED_EDGE ( 'NONE', *, *, #5169, .F. ) ;
#4432=CIRCLE ( 'NONE', #11798, 12.62506659569710266 ) ;
#4433=EDGE_LOOP ( 'NONE', ( #31520, #28479, #26857, #32336 ) ) ;
#4436=DIRECTION ( 'NONE',  ( -1.000000000000000000, -1.101824276508909887E-16, 0.000000000000000000 ) ) ;
#4438=EDGE_LOOP ( 'NONE', ( #21987, #25905, #2521, #26758 ) ) ;
#4443=FACE_OUTER_BOUND ( 'NONE', #10671, .T. ) ;
#4447=ORIENTED_EDGE ( 'NONE', *, *, #5423, .T. ) ;
#4449=LINE ( 'NONE', #19538, #12050 ) ;
#4450=ADVANCED_FACE ( 'NONE', ( #13891 ), #18787, .F. ) ;
#4451=CARTESIAN_POINT ( 'NONE',  ( 21.09992658989239089, 30.59184655352422411, 47.04930799450051637 ) ) ;
#4457=EDGE_LOOP ( 'NONE', ( #25748, #15735, #1267, #14519 ) ) ;
#4473=AXIS2_PLACEMENT_3D ( 'NONE', #12481, #10018, #27570 ) ;
#4474=VERTEX_POINT ( 'NONE', #26189 ) ;
#4475=DIRECTION ( 'NONE',  ( -1.000000000000000000, 0.000000000000000000, 0.000000000000000000 ) ) ;
#4483=ORIENTED_EDGE ( 'NONE', *, *, #7310, .T. ) ;
#4484=DIRECTION ( 'NONE',  ( -1.000000000000000000, 0.000000000000000000, 0.000000000000000000 ) ) ;
#4488=ORIENTED_EDGE ( 'NONE', *, *, #10587, .T. ) ;
#4489=DIRECTION ( 'NONE',  ( -1.000000000000000000, 0.000000000000000000, 0.000000000000000000 ) ) ;
#4501=ORIENTED_EDGE ( 'NONE', *, *, #15892, .F. ) ;
#4502=CARTESIAN_POINT ( 'NONE',  ( 21.09992658989239089, 29.34184655352418858, 47.04930799450051637 ) ) ;
#4505=TOROIDAL_SURFACE ( 'NONE', #28121, 12.61792373059897088, 0.1249999999999973216 ) ;
#4507=DIRECTION ( 'NONE',  ( -1.000000000000000000, 0.000000000000000000, 0.000000000000000000 ) ) ;
#4517=DIRECTION ( 'NONE',  ( 1.000000000000000000, 0.000000000000000000, 0.000000000000000000 ) ) ;
#4522=FACE_OUTER_BOUND ( 'NONE', #28993, .T. ) ;
#4524=DIRECTION ( 'NONE',  ( -1.000000000000000000, 0.000000000000000000, 0.000000000000000000 ) ) ;
#4525=CIRCLE ( 'NONE', #17090, 12.27641737965284641 ) ;
#4528=EDGE_CURVE ( 'NONE', #22254, #14930, #14721, .T. ) ;
#4531=ORIENTED_EDGE ( 'NONE', *, *, #22002, .T. ) ;
#4533=ADVANCED_FACE ( 'NONE', ( #19447 ), #12629, .T. ) ;
#4538=ORIENTED_EDGE ( 'NONE', *, *, #12418, .F. ) ;
#4539=VERTEX_POINT ( 'NONE', #19273 ) ;
#4544=CARTESIAN_POINT ( 'NONE',  ( 8.482002859293407582, 25.21664230456640254, 47.04930799450051637 ) ) ;
#4552=CIRCLE ( 'NONE', #27093, 12.36707279061065101 ) ;
#4554=FACE_OUTER_BOUND ( 'NONE', #25039, .T. ) ;
#4566=DIRECTION ( 'NONE',  ( -1.000000000000000000, 0.000000000000000000, 0.000000000000000000 ) ) ;
#4573=CARTESIAN_POINT ( 'NONE',  ( 33.71785032049137953, 24.96664230456639899, 47.04930799450051637 ) ) ;
#4576=VERTEX_POINT ( 'NONE', #29636 ) ;
#4577=FACE_OUTER_BOUND ( 'NONE', #22028, .T. ) ;
#4581=AXIS2_PLACEMENT_3D ( 'NONE', #21865, #12032, #16614 ) ;
#4584=EDGE_CURVE ( 'NONE', #14930, #7948, #25203, .T. ) ;
#4585=AXIS2_PLACEMENT_3D ( 'NONE', #26888, #11797, #29524 ) ;
#4588=CARTESIAN_POINT ( 'NONE',  ( 21.09992658989238734, 31.09143805560860585, 47.04930799450051637 ) ) ;
#4589=CARTESIAN_POINT ( 'NONE',  ( 33.50134396954523908, 27.09164230456639899, 47.04930799450051637 ) ) ;
#4592=DIRECTION ( 'NONE',  ( -1.000000000000000000, -1.101824276508909887E-16, 0.000000000000000000 ) ) ;
#4596=ORIENTED_EDGE ( 'NONE', *, *, #19838, .T. ) ;
#4604=EDGE_LOOP ( 'NONE', ( #7449, #30645, #7942, #4501 ) ) ;
#4605=CARTESIAN_POINT ( 'NONE',  ( 33.46699938050304013, 25.71183152705960140, 47.04930799450051637 ) ) ;
#4606=DIRECTION ( 'NONE',  ( 1.000000000000000000, 0.000000000000000000, 0.000000000000000000 ) ) ;
#4611=ORIENTED_EDGE ( 'NONE', *, *, #5533, .F. ) ;
#4612=CIRCLE ( 'NONE', #22954, 12.36707279061065279 ) ;
#4614=EDGE_LOOP ( 'NONE', ( #881, #23097, #19769, #9967 ) ) ;
#4620=AXIS2_PLACEMENT_3D ( 'NONE', #15962, #16120, #11057 ) ;
#4623=CARTESIAN_POINT ( 'NONE',  ( 21.09992658989239089, 23.59164230456639544, 47.04930799450051637 ) ) ;
#4625=EDGE_CURVE ( 'NONE', #15368, #11910, #23106, .T. ) ;
#4627=EDGE_CURVE ( 'NONE', #26804, #8205, #573, .T. ) ;
#4629=CARTESIAN_POINT ( 'NONE',  ( 21.09992658989239089, 29.59143805560861296, 47.04930799450051637 ) ) ;
#4632=FACE_OUTER_BOUND ( 'NONE', #31524, .T. ) ;
#4633=CYLINDRICAL_SURFACE ( 'NONE', #27883, 12.36707279061065279 ) ;
#4639=CARTESIAN_POINT ( 'NONE',  ( 21.09992658989238734, 38.56284415653841791, 47.04930799450051637 ) ) ;
#4641=CIRCLE ( 'NONE', #20893, 12.62506659569710443 ) ;
#4644=DIRECTION ( 'NONE',  ( -1.000000000000000000, 0.000000000000000000, 0.000000000000000000 ) ) ;
#4648=VERTEX_POINT ( 'NONE', #24372 ) ;
#4654=CARTESIAN_POINT ( 'NONE',  ( 33.72499318558949710, 26.59184655352419568, 47.04930799450051637 ) ) ;
#4656=ORIENTED_EDGE ( 'NONE', *, *, #26627, .F. ) ;
#4658=ADVANCED_FACE ( 'NONE', ( #14536 ), #4680, .T. ) ;
#4660=VECTOR ( 'NONE', #4915, 1000.000000000000000 ) ;
#4662=ORIENTED_EDGE ( 'NONE', *, *, #28051, .F. ) ;
#4663=CIRCLE ( 'NONE', #465, 0.1250000000000001110 ) ;
#4665=DIRECTION ( 'NONE',  ( -1.101824276508909887E-16, 1.000000000000000000, -0.000000000000000000 ) ) ;
#4666=FACE_OUTER_BOUND ( 'NONE', #790, .T. ) ;
#4673=CYLINDRICAL_SURFACE ( 'NONE', #16827, 12.36707279061065101 ) ;
#4676=DIRECTION ( 'NONE',  ( -1.101824276508909887E-16, 1.000000000000000000, -0.000000000000000000 ) ) ;
#4678=DIRECTION ( 'NONE',  ( -1.101824276508909887E-16, 1.000000000000000000, -0.000000000000000000 ) ) ;
#4680=CYLINDRICAL_SURFACE ( 'NONE', #21518, 12.62506659569710443 ) ;
#4682=VERTEX_POINT ( 'NONE', #21743 ) ;
#4684=DIRECTION ( 'NONE',  ( -1.101824276508909887E-16, 1.000000000000000000, -0.000000000000000000 ) ) ;
#4689=AXIS2_PLACEMENT_3D ( 'NONE', #29465, #23720, #3861 ) ;
#4691=DIRECTION ( 'NONE',  ( -1.000000000000000000, -1.101824276508909887E-16, 0.000000000000000000 ) ) ;
#4694=AXIS2_PLACEMENT_3D ( 'NONE', #14139, #23974, #23810 ) ;
#4695=CIRCLE ( 'NONE', #3639, 0.1250000000000001110 ) ;
#4696=EDGE_LOOP ( 'NONE', ( #9349, #18022, #11086, #8 ) ) ;
#4699=FACE_OUTER_BOUND ( 'NONE', #20142, .T. ) ;
#4700=AXIS2_PLACEMENT_3D ( 'NONE', #21734, #16812, #14367 ) ;
#4702=ORIENTED_EDGE ( 'NONE', *, *, #17456, .F. ) ;
#4703=ORIENTED_EDGE ( 'NONE', *, *, #31720, .T. ) ;
#4704=DIRECTION ( 'NONE',  ( -1.000000000000000000, -1.101824276508910010E-16, 0.000000000000000000 ) ) ;
#4709=CARTESIAN_POINT ( 'NONE',  ( 21.09992658989239089, 25.34184655352419213, 47.04930799450051637 ) ) ;
#4711=DIRECTION ( 'NONE',  ( -1.000000000000000000, 0.000000000000000000, 0.000000000000000000 ) ) ;
#4714=ORIENTED_EDGE ( 'NONE', *, *, #21959, .T. ) ;
#4716=CARTESIAN_POINT ( 'NONE',  ( 33.72499318558949000, 38.56284415653841791, 47.04930799450051637 ) ) ;
#4720=CIRCLE ( 'NONE', #31460, 0.1250000000000001110 ) ;
#4725=AXIS2_PLACEMENT_3D ( 'NONE', #74, #2698, #12728 ) ;
#4728=ORIENTED_EDGE ( 'NONE', *, *, #26650, .F. ) ;
#4731=LINE ( 'NONE', #12287, #19788 ) ;
#4733=DIRECTION ( 'NONE',  ( -1.000000000000000000, -1.101824276508909887E-16, 0.000000000000000000 ) ) ;
#4737=CARTESIAN_POINT ( 'NONE',  ( 33.46699938050304013, 27.71183152705960850, 47.04930799450051637 ) ) ;
#4739=ORIENTED_EDGE ( 'NONE', *, *, #6896, .F. ) ;
#4750=EDGE_CURVE ( 'NONE', #24189, #5504, #25029, .T. ) ;
#4752=CARTESIAN_POINT ( 'NONE',  ( 33.46699938050304013, 28.21183152705961206, 47.04930799450051637 ) ) ;
#4753=EDGE_CURVE ( 'NONE', #3840, #27647, #3020, .T. ) ;
#4759=ORIENTED_EDGE ( 'NONE', *, *, #16209, .F. ) ;
#4764=DIRECTION ( 'NONE',  ( -1.101824276508909887E-16, 1.000000000000000000, -0.000000000000000000 ) ) ;
#4767=SHAPE_DEFINITION_REPRESENTATION ( #32111, #14743 ) ;
#4772=DIRECTION ( 'NONE',  ( -1.101824276508909887E-16, 1.000000000000000000, -0.000000000000000000 ) ) ;
#4773=ORIENTED_EDGE ( 'NONE', *, *, #8534, .T. ) ;
#4775=LINE ( 'NONE', #14624, #5236 ) ;
#4776=ORIENTED_EDGE ( 'NONE', *, *, #24228, .F. ) ;
#4779=FACE_OUTER_BOUND ( 'NONE', #20181, .T. ) ;
#4783=EDGE_CURVE ( 'NONE', #1392, #31159, #8778, .T. ) ;
#4786=DIRECTION ( 'NONE',  ( -1.101824276508909887E-16, 1.000000000000000000, -0.000000000000000000 ) ) ;
#4790=DIRECTION ( 'NONE',  ( -1.101824276508909887E-16, 1.000000000000000000, -0.000000000000000000 ) ) ;
#4793=EDGE_CURVE ( 'NONE', #22254, #231, #2706, .T. ) ;
#4795=CIRCLE ( 'NONE', #23143, 12.36707279061065101 ) ;
#4800=CARTESIAN_POINT ( 'NONE',  ( 8.732853799281732776, 31.47145308207317171, 47.04930799450051637 ) ) ;
#4802=VERTEX_POINT ( 'NONE', #15026 ) ;
#4804=DIRECTION ( 'NONE',  ( -1.000000000000000000, 0.000000000000000000, 0.000000000000000000 ) ) ;
#4808=CARTESIAN_POINT ( 'NONE',  ( 8.823509210239553369, 28.59164230456639544, 47.04930799450051637 ) ) ;
#4809=ORIENTED_EDGE ( 'NONE', *, *, #19977, .T. ) ;
#4812=DIRECTION ( 'NONE',  ( -1.101824276508909887E-16, 1.000000000000000000, -0.000000000000000000 ) ) ;
#4815=ORIENTED_EDGE ( 'NONE', *, *, #5946, .T. ) ;
#4820=CARTESIAN_POINT ( 'NONE',  ( 33.71785032049129427, 32.21664230456639899, 47.04930799450051637 ) ) ;
#4823=TOROIDAL_SURFACE ( 'NONE', #31551, 12.40141737965288904, 0.1249999999999998612 ) ;
#4825=ADVANCED_FACE ( 'NONE', ( #27652 ), #23960, .T. ) ;
#4827=VERTEX_POINT ( 'NONE', #27822 ) ;
#4828=EDGE_CURVE ( 'NONE', #22606, #27738, #6162, .T. ) ;
#4834=CYLINDRICAL_SURFACE ( 'NONE', #942, 12.62506659569710266 ) ;
#4837=ORIENTED_EDGE ( 'NONE', *, *, #26462, .F. ) ;
#4839=ORIENTED_EDGE ( 'NONE', *, *, #4133, .F. ) ;
#4841=VECTOR ( 'NONE', #17031, 1000.000000000000000 ) ;
#4844=EDGE_LOOP ( 'NONE', ( #1144, #4483, #18182, #31824 ) ) ;
#4845=DIRECTION ( 'NONE',  ( -1.000000000000000000, 0.000000000000000000, 0.000000000000000000 ) ) ;
#4847=DIRECTION ( 'NONE',  ( -1.224646799147353207E-16, -1.349345573449484691E-32, 1.000000000000000000 ) ) ;
#4854=EDGE_CURVE ( 'NONE', #17679, #5749, #7222, .T. ) ;
#4859=AXIS2_PLACEMENT_3D ( 'NONE', #21490, #1642, #11665 ) ;
#4863=ADVANCED_FACE ( 'NONE', ( #15982 ), #1966, .T. ) ;
#4864=AXIS2_PLACEMENT_3D ( 'NONE', #766, #23727, #1233 ) ;
#4866=ADVANCED_FACE ( 'NONE', ( #18912 ), #23462, .T. ) ;
#4867=AXIS2_PLACEMENT_3D ( 'NONE', #16348, #26363, #13428 ) ;
#4869=DIRECTION ( 'NONE',  ( -1.101824276508909887E-16, 1.000000000000000000, -0.000000000000000000 ) ) ;
#4870=ORIENTED_EDGE ( 'NONE', *, *, #531, .T. ) ;
#4878=DIRECTION ( 'NONE',  ( -1.101824276508909887E-16, 1.000000000000000000, -0.000000000000000000 ) ) ;
#4879=ORIENTED_EDGE ( 'NONE', *, *, #27843, .T. ) ;
#4881=ORIENTED_EDGE ( 'NONE', *, *, #10420, .T. ) ;
#4884=DIRECTION ( 'NONE',  ( 0.000000000000000000, -0.000000000000000000, -1.000000000000000000 ) ) ;
#4888=DIRECTION ( 'NONE',  ( -1.000000000000000000, 0.000000000000000000, 0.000000000000000000 ) ) ;
#4889=CARTESIAN_POINT ( 'NONE',  ( 8.474859994195282908, 38.56284415653841791, 47.04930799450051637 ) ) ;
#4891=CIRCLE ( 'NONE', #23231, 0.1250000000000001110 ) ;
#4892=CIRCLE ( 'NONE', #13289, 12.62506659569710266 ) ;
#4897=LINE ( 'NONE', #2589, #26094 ) ;
#4900=ORIENTED_EDGE ( 'NONE', *, *, #11198, .T. ) ;
#4901=VERTEX_POINT ( 'NONE', #11542 ) ;
#4903=EDGE_CURVE ( 'NONE', #31649, #30197, #8599, .T. ) ;
#4904=ORIENTED_EDGE ( 'NONE', *, *, #7124, .T. ) ;
#4915=DIRECTION ( 'NONE',  ( -1.101824276508909887E-16, 1.000000000000000000, -0.000000000000000000 ) ) ;
#4923=DIRECTION ( 'NONE',  ( -1.000000000000000000, -1.101824276508909887E-16, 0.000000000000000000 ) ) ;
#4924=DIRECTION ( 'NONE',  ( -1.101824276508909887E-16, 1.000000000000000000, -0.000000000000000000 ) ) ;
#4933=DIRECTION ( 'NONE',  ( 0.5849755626391567320, -0.8110509177080079679, 0.000000000000000000 ) ) ;
#4935=CARTESIAN_POINT ( 'NONE',  ( 21.09992658989239089, 23.71664230456639899, 47.04930799450051637 ) ) ;
#4936=ORIENTED_EDGE ( 'NONE', *, *, #1108, .F. ) ;
#4941=DIRECTION ( 'NONE',  ( -1.000000000000000000, -1.101824276508909887E-16, 0.000000000000000000 ) ) ;
#4942=EDGE_CURVE ( 'NONE', #5204, #25724, #7200, .T. ) ;
#4943=ADVANCED_FACE ( 'NONE', ( #25831 ), #11377, .F. ) ;
#4954=AXIS2_PLACEMENT_3D ( 'NONE', #23470, #18207, #23315 ) ;
#4958=DIRECTION ( 'NONE',  ( 0.000000000000000000, -0.000000000000000000, -1.000000000000000000 ) ) ;
#4965=CARTESIAN_POINT ( 'NONE',  ( 8.474859994195282908, 38.56284415653841791, 47.04930799450051637 ) ) ;
#4970=FACE_OUTER_BOUND ( 'NONE', #26014, .T. ) ;
#4971=EDGE_CURVE ( 'NONE', #26330, #17665, #8257, .T. ) ;
#4974=CARTESIAN_POINT ( 'NONE',  ( 21.09992658989239089, 28.84143805560861296, 47.04930799450051637 ) ) ;
#4978=CARTESIAN_POINT ( 'NONE',  ( 33.72499318558949710, 27.34184655352419568, 47.04930799450051637 ) ) ;
#4979=DIRECTION ( 'NONE',  ( -1.101824276508909887E-16, 1.000000000000000000, -0.000000000000000000 ) ) ;
#4985=CIRCLE ( 'NONE', #8624, 0.1249999999999966416 ) ;
#4990=ORIENTED_EDGE ( 'NONE', *, *, #9116, .F. ) ;
#4997=CARTESIAN_POINT ( 'NONE',  ( 21.09992658989238734, 38.56284415653841791, 47.04930799450051637 ) ) ;
#5001=AXIS2_PLACEMENT_3D ( 'NONE', #917, #13563, #1232 ) ;
#5012=ADVANCED_FACE ( 'NONE', ( #14335 ), #17267, .T. ) ;
#5017=DIRECTION ( 'NONE',  ( -1.000000000000000000, 0.000000000000000000, 0.000000000000000000 ) ) ;
#5023=CARTESIAN_POINT ( 'NONE',  ( 21.09992658989238734, 38.56284415653841791, 47.04930799450051637 ) ) ;
#5024=DIRECTION ( 'NONE',  ( -1.101824276508909887E-16, 1.000000000000000000, -0.000000000000000000 ) ) ;
#5026=AXIS2_PLACEMENT_3D ( 'NONE', #8509, #13918, #28532 ) ;
#5028=ORIENTED_EDGE ( 'NONE', *, *, #22871, .F. ) ;
#5032=AXIS2_PLACEMENT_3D ( 'NONE', #12350, #24652, #27443 ) ;
#5033=ORIENTED_EDGE ( 'NONE', *, *, #22865, .T. ) ;
#5035=EDGE_CURVE ( 'NONE', #31841, #28626, #3533, .T. ) ;
#5040=CARTESIAN_POINT ( 'NONE',  ( 33.71785032049098163, 30.71664230456641675, 47.04930799450051637 ) ) ;
#5042=CARTESIAN_POINT ( 'NONE',  ( 21.09992658989238734, 32.54735957529758394, 47.04930799450051637 ) ) ;
#5050=ORIENTED_EDGE ( 'NONE', *, *, #22218, .T. ) ;
#5051=DIRECTION ( 'NONE',  ( -1.101824276508909887E-16, 1.000000000000000000, -0.000000000000000000 ) ) ;
#5058=ORIENTED_EDGE ( 'NONE', *, *, #19441, .F. ) ;
#5059=DIRECTION ( 'NONE',  ( -1.000000000000000000, -1.101824276508909764E-16, 0.000000000000000000 ) ) ;
#5065=VERTEX_POINT ( 'NONE', #7442 ) ;
#5071=EDGE_CURVE ( 'NONE', #21917, #22795, #5134, .T. ) ;
#5074=EDGE_LOOP ( 'NONE', ( #5386, #17473, #10996, #26237 ) ) ;
#5075=CARTESIAN_POINT ( 'NONE',  ( 21.09992658989238734, 31.34164230456639544, 47.04930799450051637 ) ) ;
#5076=DIRECTION ( 'NONE',  ( -1.000000000000000000, -1.101824276508909887E-16, 0.000000000000000000 ) ) ;
#5077=DIRECTION ( 'NONE',  ( -1.101824276508909887E-16, 1.000000000000000000, -0.000000000000000000 ) ) ;
#5082=ADVANCED_FACE ( 'NONE', ( #3429 ), #3037, .T. ) ;
#5084=DIRECTION ( 'NONE',  ( -1.000000000000000000, -1.101824276508909887E-16, 0.000000000000000000 ) ) ;
#5091=ORIENTED_EDGE ( 'NONE', *, *, #30269, .T. ) ;
#5092=FACE_OUTER_BOUND ( 'NONE', #9779, .T. ) ;
#5098=ORIENTED_EDGE ( 'NONE', *, *, #9790, .T. ) ;
#5099=DIRECTION ( 'NONE',  ( -1.101824276508909887E-16, 1.000000000000000000, -0.000000000000000000 ) ) ;
#5100=DIRECTION ( 'NONE',  ( -1.000000000000000000, 0.000000000000000000, 0.000000000000000000 ) ) ;
#5104=CIRCLE ( 'NONE', #29210, 12.36707279061065101 ) ;
#5112=AXIS2_PLACEMENT_3D ( 'NONE', #8913, #21055, #6459 ) ;
#5113=DIRECTION ( 'NONE',  ( -1.101824276508909887E-16, 1.000000000000000000, -0.000000000000000000 ) ) ;
#5116=EDGE_CURVE ( 'NONE', #6679, #19678, #6189, .T. ) ;
#5119=CARTESIAN_POINT ( 'NONE',  ( 33.71785032049135111, 27.71664230456639899, 47.04930799450051637 ) ) ;
#5121=EDGE_CURVE ( 'NONE', #2124, #20651, #22515, .T. ) ;
#5127=EDGE_CURVE ( 'NONE', #21917, #2124, #941, .T. ) ;
#5128=CARTESIAN_POINT ( 'NONE',  ( 21.09992658989238734, 32.34184655352418503, 47.04930799450051637 ) ) ;
#5130=EDGE_LOOP ( 'NONE', ( #15036, #27392, #19586, #25265 ) ) ;
#5132=DIRECTION ( 'NONE',  ( -1.000000000000000000, 0.000000000000000000, 0.000000000000000000 ) ) ;
#5133=FACE_OUTER_BOUND ( 'NONE', #1821, .T. ) ;
#5134=LINE ( 'NONE', #5462, #18720 ) ;
#5140=ORIENTED_EDGE ( 'NONE', *, *, #17571, .T. ) ;
#5143=AXIS2_PLACEMENT_3D ( 'NONE', #30789, #8303, #28168 ) ;
#5146=DIRECTION ( 'NONE',  ( -1.000000000000000000, 0.000000000000000000, 0.000000000000000000 ) ) ;
#5148=CIRCLE ( 'NONE', #21375, 0.1250000000000001110 ) ;
#5149=AXIS2_PLACEMENT_3D ( 'NONE', #11396, #1383, #6316 ) ;
#5152=EDGE_CURVE ( 'NONE', #25906, #12709, #19265, .T. ) ;
#5155=CARTESIAN_POINT ( 'NONE',  ( 8.732853799281734553, 38.56284415653841791, 47.04930799450051637 ) ) ;
#5156=AXIS2_PLACEMENT_3D ( 'NONE', #10734, #26130, #3321 ) ;
#5157=AXIS2_PLACEMENT_3D ( 'NONE', #6154, #14363, #24357 ) ;
#5158=VECTOR ( 'NONE', #11161, 1000.000000000000000 ) ;
#5159=ORIENTED_EDGE ( 'NONE', *, *, #28137, .F. ) ;
#5160=DIRECTION ( 'NONE',  ( -1.101824276508909887E-16, 1.000000000000000000, -0.000000000000000000 ) ) ;
#5161=ORIENTED_EDGE ( 'NONE', *, *, #671, .F. ) ;
#5162=AXIS2_PLACEMENT_3D ( 'NONE', #14009, #24004, #13846 ) ;
#5165=CARTESIAN_POINT ( 'NONE',  ( 8.732853799281732776, 25.22145308207319303, 47.04930799450051637 ) ) ;
#5166=EDGE_CURVE ( 'NONE', #3444, #15199, #20847, .T. ) ;
#5167=AXIS2_PLACEMENT_3D ( 'NONE', #22561, #14381, #20107 ) ;
#5169=EDGE_CURVE ( 'NONE', #31904, #9250, #10912, .T. ) ;
#5177=ORIENTED_EDGE ( 'NONE', *, *, #5822, .F. ) ;
#5179=ORIENTED_EDGE ( 'NONE', *, *, #3852, .T. ) ;
#5182=CARTESIAN_POINT ( 'NONE',  ( 33.37634396954518223, 32.59164230456639899, 47.04930799450051637 ) ) ;
#5191=ADVANCED_FACE ( 'NONE', ( #9323 ), #9331, .T. ) ;
#5204=VERTEX_POINT ( 'NONE', #13938 ) ;
#5207=CIRCLE ( 'NONE', #16196, 0.1250000000000001110 ) ;
#5210=FACE_OUTER_BOUND ( 'NONE', #30047, .T. ) ;
#5213=LINE ( 'NONE', #27862, #32044 ) ;
#5217=DIRECTION ( 'NONE',  ( -1.000000000000000000, 0.000000000000000000, 0.000000000000000000 ) ) ;
#5220=ORIENTED_EDGE ( 'NONE', *, *, #18289, .F. ) ;
#5221=AXIS2_PLACEMENT_3D ( 'NONE', #31500, #28702, #9008 ) ;
#5223=VERTEX_POINT ( 'NONE', #8837 ) ;
#5226=ORIENTED_EDGE ( 'NONE', *, *, #21782, .T. ) ;
#5227=EDGE_CURVE ( 'NONE', #2178, #7469, #28725, .T. ) ;
#5229=EDGE_CURVE ( 'NONE', #18133, #31159, #5148, .T. ) ;
#5230=CIRCLE ( 'NONE', #27215, 12.36707279061065101 ) ;
#5236=VECTOR ( 'NONE', #12165, 1000.000000000000000 ) ;
#5237=AXIS2_PLACEMENT_3D ( 'NONE', #6788, #16469, #4159 ) ;
#5238=EDGE_LOOP ( 'NONE', ( #20326, #14785, #17444, #17400 ) ) ;
#5239=DIRECTION ( 'NONE',  ( -1.101824276508909887E-16, 1.000000000000000000, -0.000000000000000000 ) ) ;
#5240=AXIS2_PLACEMENT_3D ( 'NONE', #13042, #2534, #15334 ) ;
#5244=TOROIDAL_SURFACE ( 'NONE', #23588, 12.40141737965284108, 0.1249999999999997918 ) ;
#5245=ORIENTED_EDGE ( 'NONE', *, *, #4398, .T. ) ;
#5250=DIRECTION ( 'NONE',  ( -1.000000000000000000, 0.000000000000000000, 0.000000000000000000 ) ) ;
#5255=EDGE_LOOP ( 'NONE', ( #26407, #23963, #30773, #28159 ) ) ;
#5260=ORIENTED_EDGE ( 'NONE', *, *, #18116, .F. ) ;
#5263=ORIENTED_EDGE ( 'NONE', *, *, #11852, .F. ) ;
#5265=DIRECTION ( 'NONE',  ( -1.000000000000000000, 0.000000000000000000, 0.000000000000000000 ) ) ;
#5270=AXIS2_PLACEMENT_3D ( 'NONE', #25346, #17787, #19925 ) ;
#5271=AXIS2_PLACEMENT_3D ( 'NONE', #24536, #14376, #24373 ) ;
#5276=ADVANCED_FACE ( 'NONE', ( #23932 ), #420, .T. ) ;
#5279=DIRECTION ( 'NONE',  ( -1.101824276508909887E-16, 1.000000000000000000, -0.000000000000000000 ) ) ;
#5282=EDGE_LOOP ( 'NONE', ( #7158, #28115, #17849, #4143 ) ) ;
#5288=DIRECTION ( 'NONE',  ( -1.101824276508909887E-16, 1.000000000000000000, -0.000000000000000000 ) ) ;
#5290=CARTESIAN_POINT ( 'NONE',  ( 21.09992658989239089, 29.09143805560861296, 47.04930799450051637 ) ) ;
#5294=CARTESIAN_POINT ( 'NONE',  ( 33.72499318558949710, 31.59143805560860585, 47.04930799450051637 ) ) ;
#5296=CIRCLE ( 'NONE', #6853, 12.62506659569710266 ) ;
#5301=DIRECTION ( 'NONE',  ( -1.101824276508909887E-16, 1.000000000000000000, -0.000000000000000000 ) ) ;
#5302=DIRECTION ( 'NONE',  ( 1.000000000000000000, 0.000000000000000000, 0.000000000000000000 ) ) ;
#5306=DIRECTION ( 'NONE',  ( -1.224646799147353207E-16, -1.349345573449484691E-32, 1.000000000000000000 ) ) ;
#5308=ORIENTED_EDGE ( 'NONE', *, *, #2524, .T. ) ;
#5309=EDGE_LOOP ( 'NONE', ( #1423, #20680, #29015, #543 ) ) ;
#5310=DIRECTION ( 'NONE',  ( -1.224646799147353207E-16, -1.349345573449484691E-32, 1.000000000000000000 ) ) ;
#5313=AXIS2_PLACEMENT_3D ( 'NONE', #22269, #27531, #2578 ) ;
#5314=DIRECTION ( 'NONE',  ( -1.101824276508909887E-16, 1.000000000000000000, -0.000000000000000000 ) ) ;
#5315=CARTESIAN_POINT ( 'NONE',  ( 21.09992658989238734, 38.56284415653841791, 47.04930799450051637 ) ) ;
#5319=ADVANCED_FACE ( 'NONE', ( #32309 ), #17192, .T. ) ;
#5323=FACE_OUTER_BOUND ( 'NONE', #30250, .T. ) ;
#5324=AXIS2_PLACEMENT_3D ( 'NONE', #16861, #15063, #4888 ) ;
#5328=AXIS2_PLACEMENT_3D ( 'NONE', #14164, #21694, #1510 ) ;
#5329=VERTEX_POINT ( 'NONE', #133 ) ;
#5331=ORIENTED_EDGE ( 'NONE', *, *, #18801, .F. ) ;
#5341=CARTESIAN_POINT ( 'NONE',  ( 21.09992658989239089, 27.84184655352419568, 47.04930799450051637 ) ) ;
#5342=AXIS2_PLACEMENT_3D ( 'NONE', #20623, #25870, #918 ) ;
#5344=EDGE_LOOP ( 'NONE', ( #5711, #22841, #12288, #10331 ) ) ;
#5345=CIRCLE ( 'NONE', #16839, 0.1250000000000001110 ) ;
#5348=ORIENTED_EDGE ( 'NONE', *, *, #2194, .F. ) ;
#5354=ORIENTED_EDGE ( 'NONE', *, *, #14424, .F. ) ;
#5362=EDGE_CURVE ( 'NONE', #19781, #17800, #15598, .T. ) ;
#5363=AXIS2_PLACEMENT_3D ( 'NONE', #7604, #14667, #19900 ) ;
#5369=DIRECTION ( 'NONE',  ( 1.000000000000000000, 0.000000000000000000, 0.000000000000000000 ) ) ;
#5370=CARTESIAN_POINT ( 'NONE',  ( 21.09992658989238734, 31.21183152705961206, 47.04930799450051637 ) ) ;
#5381=DIRECTION ( 'NONE',  ( -1.000000000000000000, 0.000000000000000000, 0.000000000000000000 ) ) ;
#5386=ORIENTED_EDGE ( 'NONE', *, *, #25817, .F. ) ;
#5387=ADVANCED_FACE ( 'NONE', ( #11951 ), #1451, .T. ) ;
#5388=ORIENTED_EDGE ( 'NONE', *, *, #11257, .F. ) ;
#5390=AXIS2_PLACEMENT_3D ( 'NONE', #18817, #25749, #26226 ) ;
#5394=CYLINDRICAL_SURFACE ( 'NONE', #26718, 12.62506659569710266 ) ;
#5403=CIRCLE ( 'NONE', #1714, 12.27641737965283575 ) ;
#5404=CYLINDRICAL_SURFACE ( 'NONE', #22816, 12.36707279061065101 ) ;
#5412=EDGE_CURVE ( 'NONE', #3113, #11837, #4731, .T. ) ;
#5414=DIRECTION ( 'NONE',  ( 0.000000000000000000, -0.000000000000000000, -1.000000000000000000 ) ) ;
#5416=DIRECTION ( 'NONE',  ( -1.101824276508909887E-16, 1.000000000000000000, -0.000000000000000000 ) ) ;
#5423=EDGE_CURVE ( 'NONE', #28525, #2384, #4897, .T. ) ;
#5425=AXIS2_PLACEMENT_3D ( 'NONE', #30653, #15385, #5536 ) ;
#5428=ORIENTED_EDGE ( 'NONE', *, *, #23971, .F. ) ;
#5429=DIRECTION ( 'NONE',  ( -1.101824276508909887E-16, 1.000000000000000000, -0.000000000000000000 ) ) ;
#5434=EDGE_CURVE ( 'NONE', #5749, #31925, #14039, .T. ) ;
#5439=DIRECTION ( 'NONE',  ( -1.101824276508909887E-16, 1.000000000000000000, -0.000000000000000000 ) ) ;
#5441=CIRCLE ( 'NONE', #8071, 0.1249999999999983763 ) ;
#5444=CYLINDRICAL_SURFACE ( 'NONE', #16363, 12.62506659569710266 ) ;
#5457=VERTEX_POINT ( 'NONE', #929 ) ;
#5462=CARTESIAN_POINT ( 'NONE',  ( 33.72499318558949000, 38.56284415653841791, 47.04930799450051637 ) ) ;
#5464=FACE_OUTER_BOUND ( 'NONE', #18096, .T. ) ;
#5465=EDGE_LOOP ( 'NONE', ( #22318, #25044, #2615, #5028 ) ) ;
#5467=CARTESIAN_POINT ( 'NONE',  ( 33.37634396954522487, 29.09164230456639899, 47.04930799450051637 ) ) ;
#5469=ORIENTED_EDGE ( 'NONE', *, *, #16209, .T. ) ;
#5476=CARTESIAN_POINT ( 'NONE',  ( 21.09992658989239089, 26.34164230456639899, 47.04930799450051637 ) ) ;
#5478=FACE_OUTER_BOUND ( 'NONE', #29296, .T. ) ;
#5482=EDGE_LOOP ( 'NONE', ( #21216, #20006, #13745, #6086 ) ) ;
#5488=DIRECTION ( 'NONE',  ( -1.101824276508909887E-16, 1.000000000000000000, -0.000000000000000000 ) ) ;
#5490=DIRECTION ( 'NONE',  ( -1.101824276508909887E-16, 1.000000000000000000, -0.000000000000000000 ) ) ;
#5493=AXIS2_PLACEMENT_3D ( 'NONE', #21090, #21403, #23249 ) ;
#5501=ORIENTED_EDGE ( 'NONE', *, *, #31177, .T. ) ;
#5502=CARTESIAN_POINT ( 'NONE',  ( 21.09992658989239089, 23.59164230456639544, 47.04930799450051637 ) ) ;
#5504=VERTEX_POINT ( 'NONE', #25400 ) ;
#5506=CIRCLE ( 'NONE', #28840, 12.27641737965283930 ) ;
#5518=DIRECTION ( 'NONE',  ( -1.101824276508909887E-16, 1.000000000000000000, -0.000000000000000000 ) ) ;
#5526=DIRECTION ( 'NONE',  ( -1.101824276508909887E-16, 1.000000000000000000, -0.000000000000000000 ) ) ;
#5528=FACE_OUTER_BOUND ( 'NONE', #11715, .T. ) ;
#5533=EDGE_CURVE ( 'NONE', #15187, #28369, #30338, .T. ) ;
#5534=CARTESIAN_POINT ( 'NONE',  ( 21.09992658989239089, 30.46664230456641675, 47.04930799450051637 ) ) ;
#5535=DIRECTION ( 'NONE',  ( -1.000000000000000000, -1.101824276508909887E-16, 0.000000000000000000 ) ) ;
#5536=DIRECTION ( 'NONE',  ( -1.000000000000000000, 0.000000000000000000, 0.000000000000000000 ) ) ;
#5538=EDGE_CURVE ( 'NONE', #22139, #19299, #11457, .T. ) ;
#5540=AXIS2_PLACEMENT_3D ( 'NONE', #10007, #29374, #24939 ) ;
#5543=DIRECTION ( 'NONE',  ( -1.101824276508909887E-16, 1.000000000000000000, -0.000000000000000000 ) ) ;
#5544=DIRECTION ( 'NONE',  ( -1.000000000000000000, 0.000000000000000000, 0.000000000000000000 ) ) ;
#5545=ADVANCED_FACE ( 'NONE', ( #10312 ), #8832, .T. ) ;
#5546=AXIS2_PLACEMENT_3D ( 'NONE', #20501, #5414, #30361 ) ;
#5549=DIRECTION ( 'NONE',  ( -1.101824276508909887E-16, 1.000000000000000000, -0.000000000000000000 ) ) ;
#5553=ORIENTED_EDGE ( 'NONE', *, *, #11012, .T. ) ;
#5555=DIRECTION ( 'NONE',  ( -1.000000000000000000, 0.000000000000000000, 0.000000000000000000 ) ) ;
#5556=CIRCLE ( 'NONE', #13940, 12.36707279061065279 ) ;
#5557=ORIENTED_EDGE ( 'NONE', *, *, #22197, .F. ) ;
#5558=EDGE_LOOP ( 'NONE', ( #31240, #31024, #30960, #3341 ) ) ;
#5559=DIRECTION ( 'NONE',  ( -1.101824276508909887E-16, 1.000000000000000000, -0.000000000000000000 ) ) ;
#5561=AXIS2_PLACEMENT_3D ( 'NONE', #22646, #19690, #25279 ) ;
#5564=CYLINDRICAL_SURFACE ( 'NONE', #12753, 12.62506659569710266 ) ;
#5571=DIRECTION ( 'NONE',  ( 0.000000000000000000, -0.000000000000000000, -1.000000000000000000 ) ) ;
#5574=EDGE_CURVE ( 'NONE', #23509, #116, #4092, .T. ) ;
#5580=FACE_OUTER_BOUND ( 'NONE', #22644, .T. ) ;
#5584=CARTESIAN_POINT ( 'NONE',  ( 21.09992658989239089, 26.71183152705960495, 47.04930799450051637 ) ) ;
#5585=FACE_OUTER_BOUND ( 'NONE', #25051, .T. ) ;
#5586=AXIS2_PLACEMENT_3D ( 'NONE', #24257, #4243, #14260 ) ;
#5587=LINE ( 'NONE', #12982, #14425 ) ;
#5588=EDGE_LOOP ( 'NONE', ( #13571, #3053, #16681, #28901 ) ) ;
#5590=VECTOR ( 'NONE', #7085, 1000.000000000000000 ) ;
#5592=ORIENTED_EDGE ( 'NONE', *, *, #28913, .F. ) ;
#5594=EDGE_CURVE ( 'NONE', #21972, #30111, #6211, .T. ) ;
#5595=CARTESIAN_POINT ( 'NONE',  ( 8.823509210239555145, 28.84164230456639544, 47.04930799450051637 ) ) ;
#5596=DIRECTION ( 'NONE',  ( -1.000000000000000000, 0.000000000000000000, 0.000000000000000000 ) ) ;
#5600=LINE ( 'NONE', #21814, #25417 ) ;
#5601=CARTESIAN_POINT ( 'NONE',  ( 8.474859994195282908, 38.56284415653841791, 47.04930799450051637 ) ) ;
#5608=FACE_OUTER_BOUND ( 'NONE', #24785, .T. ) ;
#5609=CARTESIAN_POINT ( 'NONE',  ( 21.09992658989239089, 30.09164230456639544, 47.04930799450051637 ) ) ;
#5613=ORIENTED_EDGE ( 'NONE', *, *, #5116, .T. ) ;
#5614=CARTESIAN_POINT ( 'NONE',  ( 33.50134396954521776, 29.59164230456639899, 47.04930799450051637 ) ) ;
#5617=ORIENTED_EDGE ( 'NONE', *, *, #23857, .T. ) ;
#5627=ADVANCED_FACE ( 'NONE', ( #3879 ), #26362, .T. ) ;
#5631=AXIS2_PLACEMENT_3D ( 'NONE', #31091, #5823, #28619 ) ;
#5632=CARTESIAN_POINT ( 'NONE',  ( 33.46699938050304013, 27.21183152705960495, 47.04930799450051637 ) ) ;
#5636=ADVANCED_FACE ( 'NONE', ( #19282 ), #12508, .T. ) ;
#5640=ORIENTED_EDGE ( 'NONE', *, *, #1706, .T. ) ;
#5642=DIRECTION ( 'NONE',  ( -1.224646799147353207E-16, -1.349345573449484691E-32, 1.000000000000000000 ) ) ;
#5647=AXIS2_PLACEMENT_3D ( 'NONE', #5785, #23339, #15793 ) ;
#5659=CARTESIAN_POINT ( 'NONE',  ( 21.09992658989239089, 27.84143805560860940, 47.04930799450051637 ) ) ;
#5662=AXIS2_PLACEMENT_3D ( 'NONE', #3001, #29780, #19920 ) ;
#5663=DIRECTION ( 'NONE',  ( -1.101824276508909887E-16, 1.000000000000000000, -0.000000000000000000 ) ) ;
#5666=DIRECTION ( 'NONE',  ( -1.101824276508909887E-16, 1.000000000000000000, -0.000000000000000000 ) ) ;
#5671=AXIS2_PLACEMENT_3D ( 'NONE', #13463, #20830, #5910 ) ;
#5674=AXIS2_PLACEMENT_3D ( 'NONE', #2977, #15615, #22688 ) ;
#5675=AXIS2_PLACEMENT_3D ( 'NONE', #31459, #16183, #11424 ) ;
#5680=AXIS2_PLACEMENT_3D ( 'NONE', #19550, #24157, #27105 ) ;
#5682=ORIENTED_EDGE ( 'NONE', *, *, #18204, .T. ) ;
#5683=DIRECTION ( 'NONE',  ( -1.101824276508909887E-16, 1.000000000000000000, -0.000000000000000000 ) ) ;
#5685=DIRECTION ( 'NONE',  ( -1.000000000000000000, 0.000000000000000000, 0.000000000000000000 ) ) ;
#5686=DIRECTION ( 'NONE',  ( -1.000000000000000000, 0.000000000000000000, 0.000000000000000000 ) ) ;
#5687=VERTEX_POINT ( 'NONE', #8651 ) ;
#5689=ORIENTED_EDGE ( 'NONE', *, *, #22934, .F. ) ;
#5692=VERTEX_POINT ( 'NONE', #11274 ) ;
#5694=DIRECTION ( 'NONE',  ( -1.101824276508909887E-16, 1.000000000000000000, -0.000000000000000000 ) ) ;
#5698=LINE ( 'NONE', #11118, #2710 ) ;
#5700=ORIENTED_EDGE ( 'NONE', *, *, #24671, .F. ) ;
#5702=TOROIDAL_SURFACE ( 'NONE', #9892, 12.61792373059898686, 0.1249999999999964195 ) ;
#5705=AXIS2_PLACEMENT_3D ( 'NONE', #26437, #21495, #29720 ) ;
#5709=DIRECTION ( 'NONE',  ( -1.000000000000000000, 0.000000000000000000, 0.000000000000000000 ) ) ;
#5711=ORIENTED_EDGE ( 'NONE', *, *, #8662, .F. ) ;
#5713=ADVANCED_FACE ( 'NONE', ( #1568 ), #7281, .T. ) ;
#5715=ADVANCED_FACE ( 'NONE', ( #19119 ), #28222, .T. ) ;
#5716=ORIENTED_EDGE ( 'NONE', *, *, #22671, .F. ) ;
#5717=CARTESIAN_POINT ( 'NONE',  ( 8.823509210239507183, 24.09164230456639544, 47.04930799450051637 ) ) ;
#5718=ADVANCED_FACE ( 'NONE', ( #6666 ), #25037, .T. ) ;
#5720=VECTOR ( 'NONE', #9092, 1000.000000000000000 ) ;
#5721=ORIENTED_EDGE ( 'NONE', *, *, #10847, .T. ) ;
#5728=ORIENTED_EDGE ( 'NONE', *, *, #18773, .F. ) ;
#5730=ORIENTED_EDGE ( 'NONE', *, *, #15663, .F. ) ;
#5731=CIRCLE ( 'NONE', #474, 12.36707279061065101 ) ;
#5742=CARTESIAN_POINT ( 'NONE',  ( 21.09992658989238734, 32.59164230456639899, 47.04930799450051637 ) ) ;
#5744=ORIENTED_EDGE ( 'NONE', *, *, #20077, .F. ) ;
#5747=CIRCLE ( 'NONE', #488, 0.1250000000000001110 ) ;
#5749=VERTEX_POINT ( 'NONE', #29642 ) ;
#5755=EDGE_CURVE ( 'NONE', #25242, #27840, #6723, .T. ) ;
#5756=AXIS2_PLACEMENT_3D ( 'NONE', #24590, #2276, #22124 ) ;
#5758=ADVANCED_FACE ( 'NONE', ( #14872 ), #24879, .F. ) ;
#5761=EDGE_CURVE ( 'NONE', #22214, #3389, #31894, .T. ) ;
#5767=CARTESIAN_POINT ( 'NONE',  ( 21.09992658989239089, 28.84164230456639544, 47.04930799450051637 ) ) ;
#5769=CIRCLE ( 'NONE', #9956, 12.51969897791880015 ) ;
#5773=DIRECTION ( 'NONE',  ( -1.101824276508909887E-16, 1.000000000000000000, -0.000000000000000000 ) ) ;
#5781=CIRCLE ( 'NONE', #25691, 0.1250000000000001110 ) ;
#5782=AXIS2_PLACEMENT_3D ( 'NONE', #31194, #13632, #21809 ) ;
#5783=DIRECTION ( 'NONE',  ( -1.000000000000000000, -1.101824276508909887E-16, 0.000000000000000000 ) ) ;
#5784=ORIENTED_EDGE ( 'NONE', *, *, #19854, .T. ) ;
#5785=CARTESIAN_POINT ( 'NONE',  ( 21.09992658989238734, 38.56284415653841791, 47.04930799450051637 ) ) ;
#5793=EDGE_CURVE ( 'NONE', #28202, #6910, #19295, .T. ) ;
#5794=ADVANCED_FACE ( 'NONE', ( #24379 ), #17731, .T. ) ;
#5805=CIRCLE ( 'NONE', #27803, 0.1250000000000001110 ) ;
#5808=TOROIDAL_SURFACE ( 'NONE', #7376, 12.40141737965288726, 0.1250000000000003331 ) ;
#5809=AXIS2_PLACEMENT_3D ( 'NONE', #18526, #1134, #26078 ) ;
#5812=EDGE_LOOP ( 'NONE', ( #26107, #18547, #641, #2117 ) ) ;
#5816=CARTESIAN_POINT ( 'NONE',  ( 8.732853799281738105, 28.96183152705961206, 47.04930799450051637 ) ) ;
#5819=DIRECTION ( 'NONE',  ( -1.224646799147353207E-16, -1.349345573449484691E-32, 1.000000000000000000 ) ) ;
#5822=EDGE_CURVE ( 'NONE', #12300, #2537, #32443, .T. ) ;
#5823=DIRECTION ( 'NONE',  ( -1.101824276508909887E-16, 1.000000000000000000, -0.000000000000000000 ) ) ;
#5825=ORIENTED_EDGE ( 'NONE', *, *, #20564, .F. ) ;
#5830=ORIENTED_EDGE ( 'NONE', *, *, #17573, .T. ) ;
#5837=EDGE_CURVE ( 'NONE', #23957, #16025, #28241, .T. ) ;
#5841=VERTEX_POINT ( 'NONE', #19456 ) ;
#5845=EDGE_LOOP ( 'NONE', ( #18482, #7052, #16904, #12038 ) ) ;
#5871=CARTESIAN_POINT ( 'NONE',  ( 21.09992658989238734, 32.34164230456639899, 47.04930799450051637 ) ) ;
#5876=DIRECTION ( 'NONE',  ( 1.000000000000000000, 0.000000000000000000, 0.000000000000000000 ) ) ;
#5884=TOROIDAL_SURFACE ( 'NONE', #17390, 12.40141737965283397, 0.1249999999999992922 ) ;
#5886=ORIENTED_EDGE ( 'NONE', *, *, #25435, .T. ) ;
#5887=TOROIDAL_SURFACE ( 'NONE', #10086, 12.61792373059897265, 0.1249999999999971551 ) ;
#5891=FACE_OUTER_BOUND ( 'NONE', #10062, .T. ) ;
#5892=DIRECTION ( 'NONE',  ( -1.101824276508909887E-16, 1.000000000000000000, -0.000000000000000000 ) ) ;
#5903=CARTESIAN_POINT ( 'NONE',  ( 8.732853799281732776, 38.56284415653841791, 47.04930799450051637 ) ) ;
#5906=DIRECTION ( 'NONE',  ( -1.000000000000000000, 0.000000000000000000, 0.000000000000000000 ) ) ;
#5909=FACE_OUTER_BOUND ( 'NONE', #8842, .T. ) ;
#5910=DIRECTION ( 'NONE',  ( -1.000000000000000000, 0.000000000000000000, 0.000000000000000000 ) ) ;
#5911=ORIENTED_EDGE ( 'NONE', *, *, #26650, .T. ) ;
#5912=DIRECTION ( 'NONE',  ( -1.000000000000000000, 0.000000000000000000, 0.000000000000000000 ) ) ;
#5915=AXIS2_PLACEMENT_3D ( 'NONE', #16724, #19522, #11988 ) ;
#5916=CIRCLE ( 'NONE', #30546, 0.1250000000000001110 ) ;
#5917=ORIENTED_EDGE ( 'NONE', *, *, #31720, .F. ) ;
#5920=ORIENTED_EDGE ( 'NONE', *, *, #1851, .T. ) ;
#5924=ORIENTED_EDGE ( 'NONE', *, *, #31820, .T. ) ;
#5925=DIRECTION ( 'NONE',  ( 0.000000000000000000, -0.000000000000000000, -1.000000000000000000 ) ) ;
#5928=EDGE_LOOP ( 'NONE', ( #7459, #14271, #25219, #19380 ) ) ;
#5931=DIRECTION ( 'NONE',  ( -1.000000000000000000, 0.000000000000000000, 0.000000000000000000 ) ) ;
#5932=DIRECTION ( 'NONE',  ( -1.000000000000000000, -1.101824276508909887E-16, 0.000000000000000000 ) ) ;
#5933=DIRECTION ( 'NONE',  ( -1.000000000000000000, -1.101824276508910010E-16, 0.000000000000000000 ) ) ;
#5938=SURFACE_STYLE_USAGE ( .BOTH. , #28735 ) ;
#5942=CARTESIAN_POINT ( 'NONE',  ( 8.823509210239521394, 25.84164230456639899, 47.04930799450051637 ) ) ;
#5945=EDGE_CURVE ( 'NONE', #15557, #27550, #23544, .T. ) ;
#5946=EDGE_CURVE ( 'NONE', #321, #12078, #27748, .T. ) ;
#5948=CIRCLE ( 'NONE', #4368, 12.36707279061065101 ) ;
#5949=CARTESIAN_POINT ( 'NONE',  ( 8.474859994195286461, 24.09184655352419213, 47.04930799450051637 ) ) ;
#5951=AXIS2_PLACEMENT_3D ( 'NONE', #965, #10987, #20982 ) ;
#5954=DIRECTION ( 'NONE',  ( -1.101824276508909887E-16, 1.000000000000000000, -0.000000000000000000 ) ) ;
#5959=VECTOR ( 'NONE', #8644, 1000.000000000000000 ) ;
#5963=AXIS2_PLACEMENT_3D ( 'NONE', #3504, #27985, #13698 ) ;
#5964=CIRCLE ( 'NONE', #8582, 0.1250000000000001110 ) ;
#5966=CARTESIAN_POINT ( 'NONE',  ( 33.72499318558949710, 29.09143805560861296, 47.04930799450051637 ) ) ;
#5969=DIRECTION ( 'NONE',  ( -1.000000000000000000, 0.000000000000000000, 0.000000000000000000 ) ) ;
#5972=FACE_OUTER_BOUND ( 'NONE', #21824, .T. ) ;
#5974=DIRECTION ( 'NONE',  ( 1.000000000000000000, 0.000000000000000000, 0.000000000000000000 ) ) ;
#5975=AXIS2_PLACEMENT_3D ( 'NONE', #11580, #21575, #21251 ) ;
#5977=DIRECTION ( 'NONE',  ( 1.000000000000000000, 0.000000000000000000, 0.000000000000000000 ) ) ;
#5984=DIRECTION ( 'NONE',  ( -1.101824276508909887E-16, 1.000000000000000000, -0.000000000000000000 ) ) ;
#5988=EDGE_CURVE ( 'NONE', #20933, #3444, #2062, .T. ) ;
#5992=CARTESIAN_POINT ( 'NONE',  ( 8.732853799281738105, 27.71183152705960850, 47.04930799450051637 ) ) ;
#5994=ORIENTED_EDGE ( 'NONE', *, *, #19785, .F. ) ;
#5996=ADVANCED_FACE ( 'NONE', ( #23221 ), #17778, .T. ) ;
#5999=CYLINDRICAL_SURFACE ( 'NONE', #11416, 12.62506659569710266 ) ;
#6002=EDGE_CURVE ( 'NONE', #9593, #22169, #24594, .T. ) ;
#6003=AXIS2_PLACEMENT_3D ( 'NONE', #1840, #6927, #23834 ) ;
#6006=CARTESIAN_POINT ( 'NONE',  ( 21.09992658989239089, 27.34143805560860940, 47.04930799450051637 ) ) ;
#6011=DIRECTION ( 'NONE',  ( -1.000000000000000000, 0.000000000000000000, 0.000000000000000000 ) ) ;
#6015=CARTESIAN_POINT ( 'NONE',  ( 21.09992658989239089, 29.84164230456639899, 47.04930799450051637 ) ) ;
#6016=DIRECTION ( 'NONE',  ( 1.000000000000000000, 0.000000000000000000, 0.000000000000000000 ) ) ;
#6018=ORIENTED_EDGE ( 'NONE', *, *, #25247, .F. ) ;
#6019=DIRECTION ( 'NONE',  ( 0.000000000000000000, -0.000000000000000000, -1.000000000000000000 ) ) ;
#6021=DIRECTION ( 'NONE',  ( 1.000000000000000000, 0.000000000000000000, 0.000000000000000000 ) ) ;
#6024=ORIENTED_EDGE ( 'NONE', *, *, #2486, .F. ) ;
#6025=FACE_OUTER_BOUND ( 'NONE', #9430, .T. ) ;
#6033=ORIENTED_EDGE ( 'NONE', *, *, #30807, .F. ) ;
#6035=AXIS2_PLACEMENT_3D ( 'NONE', #20212, #27275, #9725 ) ;
#6041=ADVANCED_FACE ( 'NONE', ( #8450 ), #20398, .T. ) ;
#6061=CARTESIAN_POINT ( 'NONE',  ( 8.732853799281731000, 28.22145308207318237, 47.04930799450051637 ) ) ;
#6062=ORIENTED_EDGE ( 'NONE', *, *, #8060, .F. ) ;
#6066=CARTESIAN_POINT ( 'NONE',  ( 21.09992658989239089, 25.96664230456639899, 47.04930799450051637 ) ) ;
#6067=DIRECTION ( 'NONE',  ( -1.000000000000000000, 0.000000000000000000, 0.000000000000000000 ) ) ;
#6070=CARTESIAN_POINT ( 'NONE',  ( 21.09992658989239089, 27.09184655352419568, 47.04930799450051637 ) ) ;
#6072=ORIENTED_EDGE ( 'NONE', *, *, #30135, .T. ) ;
#6073=ADVANCED_FACE ( 'NONE', ( #14018 ), #18808, .T. ) ;
#6080=ADVANCED_FACE ( 'NONE', ( #18920 ), #25654, .T. ) ;
#6081=CIRCLE ( 'NONE', #32282, 12.27641737965286772 ) ;
#6083=CARTESIAN_POINT ( 'NONE',  ( 33.46699938050304013, 25.47145308207319303, 47.04930799450050927 ) ) ;
#6084=FACE_OUTER_BOUND ( 'NONE', #26768, .T. ) ;
#6086=ORIENTED_EDGE ( 'NONE', *, *, #21961, .F. ) ;
#6094=DIRECTION ( 'NONE',  ( 1.000000000000000000, 0.000000000000000000, 0.000000000000000000 ) ) ;
#6098=ORIENTED_EDGE ( 'NONE', *, *, #24228, .T. ) ;
#6099=DIRECTION ( 'NONE',  ( -1.101824276508909887E-16, 1.000000000000000000, -0.000000000000000000 ) ) ;
#6100=LINE ( 'NONE', #13659, #14661 ) ;
#6101=ORIENTED_EDGE ( 'NONE', *, *, #24054, .T. ) ;
#6104=AXIS2_PLACEMENT_3D ( 'NONE', #7624, #4665, #12881 ) ;
#6107=CARTESIAN_POINT ( 'NONE',  ( 21.09992658989238734, 31.47145308207317171, 47.04930799450051637 ) ) ;
#6108=CIRCLE ( 'NONE', #16575, 12.62506659569710266 ) ;
#6110=CARTESIAN_POINT ( 'NONE',  ( 8.474859994195286461, 26.09143805560860940, 47.04930799450051637 ) ) ;
#6117=ADVANCED_FACE ( 'NONE', ( #3836 ), #28284, .T. ) ;
#6120=CARTESIAN_POINT ( 'NONE',  ( 33.50134396954518223, 32.59164230456639899, 47.04930799450051637 ) ) ;
#6129=DIRECTION ( 'NONE',  ( 0.000000000000000000, -0.000000000000000000, -1.000000000000000000 ) ) ;
#6135=CYLINDRICAL_SURFACE ( 'NONE', #15322, 12.36707279061065101 ) ;
#6138=CARTESIAN_POINT ( 'NONE',  ( 21.09992658989238734, 30.71183152705961916, 47.04930799450051637 ) ) ;
#6140=CIRCLE ( 'NONE', #375, 0.1250000000000001110 ) ;
#6146=EDGE_CURVE ( 'NONE', #7677, #29646, #16732, .T. ) ;
#6147=ORIENTED_EDGE ( 'NONE', *, *, #23092, .F. ) ;
#6149=EDGE_CURVE ( 'NONE', #15078, #12341, #7837, .T. ) ;
#6154=CARTESIAN_POINT ( 'NONE',  ( 21.09992658989238734, 32.59164230456639899, 47.04930799450051637 ) ) ;
#6156=TOROIDAL_SURFACE ( 'NONE', #17156, 12.40141737965281088, 0.1249999999999987788 ) ;
#6158=DIRECTION ( 'NONE',  ( -1.000000000000000000, 0.000000000000000000, 0.000000000000000000 ) ) ;
#6162=CIRCLE ( 'NONE', #22396, 12.62506659569710266 ) ;
#6166=DIRECTION ( 'NONE',  ( -1.101824276508909887E-16, 1.000000000000000000, -0.000000000000000000 ) ) ;
#6167=DIRECTION ( 'NONE',  ( -1.101824276508909887E-16, 1.000000000000000000, -0.000000000000000000 ) ) ;
#6170=CARTESIAN_POINT ( 'NONE',  ( 8.474859994195281132, 31.09143805560860585, 47.04930799450051637 ) ) ;
#6174=CARTESIAN_POINT ( 'NONE',  ( 21.09992658989239089, 26.09164230456639899, 47.04930799450051637 ) ) ;
#6177=CYLINDRICAL_SURFACE ( 'NONE', #30623, 12.36707279061065101 ) ;
#6178=ORIENTED_EDGE ( 'NONE', *, *, #13247, .F. ) ;
#6180=CARTESIAN_POINT ( 'NONE',  ( 8.474859994195281132, 31.34184655352422766, 47.04930799450051637 ) ) ;
#6181=ORIENTED_EDGE ( 'NONE', *, *, #14388, .F. ) ;
#6182=EDGE_LOOP ( 'NONE', ( #29548, #31097, #8929, #26099 ) ) ;
#6188=AXIS2_PLACEMENT_3D ( 'NONE', #20417, #3176, #80 ) ;
#6189=CIRCLE ( 'NONE', #11406, 12.27641737965285706 ) ;
#6194=ORIENTED_EDGE ( 'NONE', *, *, #13094, .F. ) ;
#6197=DIRECTION ( 'NONE',  ( -1.000000000000000000, 0.000000000000000000, 0.000000000000000000 ) ) ;
#6200=AXIS2_PLACEMENT_3D ( 'NONE', #15482, #64, #10085 ) ;
#6204=ORIENTED_EDGE ( 'NONE', *, *, #22218, .F. ) ;
#6205=DIRECTION ( 'NONE',  ( 0.000000000000000000, -0.000000000000000000, -1.000000000000000000 ) ) ;
#6206=CIRCLE ( 'NONE', #10410, 12.36707279061065101 ) ;
#6207=DIRECTION ( 'NONE',  ( -1.000000000000000000, 0.000000000000000000, 0.000000000000000000 ) ) ;
#6210=TOROIDAL_SURFACE ( 'NONE', #23521, 12.40141737965288371, 0.1249999999999996253 ) ;
#6211=CIRCLE ( 'NONE', #20876, 0.1250000000000001110 ) ;
#6214=EDGE_CURVE ( 'NONE', #4827, #8205, #8368, .T. ) ;
#6222=CARTESIAN_POINT ( 'NONE',  ( 33.46699938050303302, 38.56284415653841791, 47.04930799450051637 ) ) ;
#6234=ORIENTED_EDGE ( 'NONE', *, *, #31859, .F. ) ;
#6236=EDGE_CURVE ( 'NONE', #16953, #7900, #30391, .T. ) ;
#6237=DIRECTION ( 'NONE',  ( -1.000000000000000000, -1.101824276508909887E-16, 0.000000000000000000 ) ) ;
#6238=DIRECTION ( 'NONE',  ( -1.101824276508909887E-16, 1.000000000000000000, -0.000000000000000000 ) ) ;
#6239=AXIS2_PLACEMENT_3D ( 'NONE', #9501, #24587, #29526 ) ;
#6244=ORIENTED_EDGE ( 'NONE', *, *, #5412, .F. ) ;
#6245=CARTESIAN_POINT ( 'NONE',  ( 8.474859994195281132, 32.09143805560860585, 47.04930799450051637 ) ) ;
#6251=( NAMED_UNIT ( * ) PLANE_ANGLE_UNIT ( ) SI_UNIT ( $, .RADIAN. ) );
#6253=ORIENTED_EDGE ( 'NONE', *, *, #13094, .T. ) ;
#6255=DIRECTION ( 'NONE',  ( -1.101824276508909887E-16, 1.000000000000000000, -0.000000000000000000 ) ) ;
#6260=DIRECTION ( 'NONE',  ( -1.101824276508909887E-16, 1.000000000000000000, -0.000000000000000000 ) ) ;
#6265=TOROIDAL_SURFACE ( 'NONE', #23028, 12.40141737965287660, 0.1250000000000007772 ) ;
#6268=TOROIDAL_SURFACE ( 'NONE', #6800, 12.40141737965283220, 0.1250000000000002498 ) ;
#6269=CIRCLE ( 'NONE', #9953, 0.1250000000000001110 ) ;
#6271=DIRECTION ( 'NONE',  ( -1.000000000000000000, 0.000000000000000000, 0.000000000000000000 ) ) ;
#6280=EDGE_LOOP ( 'NONE', ( #25294, #28340, #32270, #3495 ) ) ;
#6281=AXIS2_PLACEMENT_3D ( 'NONE', #20040, #27756, #9716 ) ;
#6282=CARTESIAN_POINT ( 'NONE',  ( 21.09992658989239089, 28.34143805560861296, 47.04930799450051637 ) ) ;
#6284=LINE ( 'NONE', #3981, #537 ) ;
#6286=CARTESIAN_POINT ( 'NONE',  ( 0.000000000000000000, 0.000000000000000000, 0.000000000000000000 ) ) ;
#6293=CARTESIAN_POINT ( 'NONE',  ( 8.823509210239569356, 30.09164230456639544, 47.04930799450051637 ) ) ;
#6299=ORIENTED_EDGE ( 'NONE', *, *, #29258, .T. ) ;
#6304=EDGE_CURVE ( 'NONE', #19672, #24538, #4449, .T. ) ;
#6308=AXIS2_PLACEMENT_3D ( 'NONE', #28540, #21779, #31162 ) ;
#6312=CIRCLE ( 'NONE', #28854, 12.62506659569710266 ) ;
#6315=DIRECTION ( 'NONE',  ( -1.000000000000000000, -1.101824276508909887E-16, 0.000000000000000000 ) ) ;
#6316=DIRECTION ( 'NONE',  ( -1.000000000000000000, 0.000000000000000000, 0.000000000000000000 ) ) ;
#6318=CIRCLE ( 'NONE', #25735, 0.1250000000000001110 ) ;
#6325=EDGE_LOOP ( 'NONE', ( #23278, #9581, #21890, #31152 ) ) ;
#6327=DIRECTION ( 'NONE',  ( -1.101824276508909887E-16, 1.000000000000000000, -0.000000000000000000 ) ) ;
#6333=DIRECTION ( 'NONE',  ( -1.101824276508909887E-16, 1.000000000000000000, -0.000000000000000000 ) ) ;
#6334=DIRECTION ( 'NONE',  ( -1.101824276508909887E-16, 1.000000000000000000, -0.000000000000000000 ) ) ;
#6335=DIRECTION ( 'NONE',  ( -1.101824276508909887E-16, 1.000000000000000000, -0.000000000000000000 ) ) ;
#6338=DIRECTION ( 'NONE',  ( 1.000000000000000000, 0.000000000000000000, 0.000000000000000000 ) ) ;
#6341=ORIENTED_EDGE ( 'NONE', *, *, #8229, .T. ) ;
#6344=DIRECTION ( 'NONE',  ( -1.000000000000000000, 0.000000000000000000, 0.000000000000000000 ) ) ;
#6345=ADVANCED_FACE ( 'NONE', ( #14471 ), #17807, .T. ) ;
#6346=EDGE_CURVE ( 'NONE', #16617, #2537, #21985, .T. ) ;
#6347=ORIENTED_EDGE ( 'NONE', *, *, #744, .T. ) ;
#6348=ADVANCED_FACE ( 'NONE', ( #4779 ), #24465, .T. ) ;
#6351=EDGE_CURVE ( 'NONE', #22098, #15469, #9212, .T. ) ;
#6357=APPLICATION_CONTEXT ( 'automotive_design' ) ;
#6359=CIRCLE ( 'NONE', #17295, 0.1249999999999983763 ) ;
#6361=CYLINDRICAL_SURFACE ( 'NONE', #20014, 12.36707279061065101 ) ;
#6388=LINE ( 'NONE', #13783, #28855 ) ;
#6389=DIRECTION ( 'NONE',  ( -1.000000000000000000, 0.000000000000000000, 0.000000000000000000 ) ) ;
#6390=EDGE_CURVE ( 'NONE', #11991, #14790, #14087, .T. ) ;
#6392=CIRCLE ( 'NONE', #27365, 12.62506659569710266 ) ;
#6393=CIRCLE ( 'NONE', #24814, 12.27641737965280555 ) ;
#6394=ORIENTED_EDGE ( 'NONE', *, *, #15635, .T. ) ;
#6395=ADVANCED_FACE ( 'NONE', ( #5585 ), #10518, .T. ) ;
#6396=CARTESIAN_POINT ( 'NONE',  ( 21.09992658989238734, 31.84143805560860940, 47.04930799450051637 ) ) ;
#6404=CARTESIAN_POINT ( 'NONE',  ( 21.09992658989239089, 28.72145308207318237, 47.04930799450051637 ) ) ;
#6407=DIRECTION ( 'NONE',  ( -1.101824276508909887E-16, 1.000000000000000000, -0.000000000000000000 ) ) ;
#6415=( NAMED_UNIT ( * ) SI_UNIT ( $, .STERADIAN. ) SOLID_ANGLE_UNIT ( ) );
#6418=DIRECTION ( 'NONE',  ( -1.000000000000000000, 0.000000000000000000, 0.000000000000000000 ) ) ;
#6421=CIRCLE ( 'NONE', #5915, 0.1249999999999983763 ) ;
#6423=CARTESIAN_POINT ( 'NONE',  ( 21.09992658989238734, 31.09184655352422411, 47.04930799450051637 ) ) ;
#6427=CARTESIAN_POINT ( 'NONE',  ( 33.72499318558949000, 38.56284415653841791, 47.04930799450051637 ) ) ;
#6429=ADVANCED_FACE ( 'NONE', ( #17894 ), #3102, .T. ) ;
#6430=CIRCLE ( 'NONE', #10645, 12.36707279061065101 ) ;
#6435=EDGE_CURVE ( 'NONE', #23854, #116, #17724, .T. ) ;
#6439=EDGE_CURVE ( 'NONE', #29925, #32344, #31379, .T. ) ;
#6442=LINE ( 'NONE', #26460, #18035 ) ;
#6444=CARTESIAN_POINT ( 'NONE',  ( 33.72499318558949710, 26.59143805560860940, 47.04930799450051637 ) ) ;
#6452=AXIS2_PLACEMENT_3D ( 'NONE', #9981, #22925, #19981 ) ;
#6455=CARTESIAN_POINT ( 'NONE',  ( 8.698509210239549816, 28.34164230456639544, 47.04930799450051637 ) ) ;
#6459=DIRECTION ( 'NONE',  ( -1.000000000000000000, 0.000000000000000000, 0.000000000000000000 ) ) ;
#6461=ORIENTED_EDGE ( 'NONE', *, *, #221, .F. ) ;
#6464=DIRECTION ( 'NONE',  ( -1.101824276508909887E-16, 1.000000000000000000, -0.000000000000000000 ) ) ;
#6467=CARTESIAN_POINT ( 'NONE',  ( 21.09992658989239089, 26.21664230456639899, 47.04930799450051637 ) ) ;
#6471=ORIENTED_EDGE ( 'NONE', *, *, #14198, .T. ) ;
#6475=EDGE_LOOP ( 'NONE', ( #5388, #11403, #4367, #2211 ) ) ;
#6477=AXIS2_PLACEMENT_3D ( 'NONE', #22767, #7523, #443 ) ;
#6478=DIRECTION ( 'NONE',  ( -1.000000000000000000, 0.000000000000000000, 0.000000000000000000 ) ) ;
#6482=EDGE_LOOP ( 'NONE', ( #11460, #1704, #15754, #19240 ) ) ;
#6486=AXIS2_PLACEMENT_3D ( 'NONE', #23191, #23354, #10735 ) ;
#6487=EDGE_CURVE ( 'NONE', #16617, #5692, #6206, .T. ) ;
#6491=DIRECTION ( 'NONE',  ( -1.101824276508909887E-16, 1.000000000000000000, -0.000000000000000000 ) ) ;
#6494=CARTESIAN_POINT ( 'NONE',  ( 8.474859994195286461, 26.09184655352419213, 47.04930799450051637 ) ) ;
#6495=ORIENTED_EDGE ( 'NONE', *, *, #9867, .T. ) ;
#6498=DIRECTION ( 'NONE',  ( -1.101824276508909887E-16, 1.000000000000000000, -0.000000000000000000 ) ) ;
#6507=DIRECTION ( 'NONE',  ( -1.101824276508909887E-16, 1.000000000000000000, -0.000000000000000000 ) ) ;
#6513=AXIS2_PLACEMENT_3D ( 'NONE', #28646, #3696, #6928 ) ;
#6515=AXIS2_PLACEMENT_3D ( 'NONE', #10041, #20203, #182 ) ;
#6518=ORIENTED_EDGE ( 'NONE', *, *, #16373, .T. ) ;
#6519=DIRECTION ( 'NONE',  ( -1.000000000000000000, 0.000000000000000000, 0.000000000000000000 ) ) ;
#6522=DIRECTION ( 'NONE',  ( -1.101824276508909887E-16, 1.000000000000000000, -0.000000000000000000 ) ) ;
#6526=EDGE_CURVE ( 'NONE', #22606, #9420, #15644, .T. ) ;
#6527=EDGE_CURVE ( 'NONE', #17250, #31644, #20993, .T. ) ;
#6529=ORIENTED_EDGE ( 'NONE', *, *, #18874, .F. ) ;
#6541=AXIS2_PLACEMENT_3D ( 'NONE', #17093, #7588, #27111 ) ;
#6542=ORIENTED_EDGE ( 'NONE', *, *, #303, .F. ) ;
#6548=AXIS2_PLACEMENT_3D ( 'NONE', #30515, #18653, #15891 ) ;
#6551=ORIENTED_EDGE ( 'NONE', *, *, #21432, .T. ) ;
#6554=FACE_OUTER_BOUND ( 'NONE', #5130, .T. ) ;
#6555=CARTESIAN_POINT ( 'NONE',  ( 21.09992658989238734, 38.56284415653841791, 47.04930799450051637 ) ) ;
#6559=ORIENTED_EDGE ( 'NONE', *, *, #5755, .T. ) ;
#6560=AXIS2_PLACEMENT_3D ( 'NONE', #27929, #26102, #31045 ) ;
#6563=AXIS2_PLACEMENT_3D ( 'NONE', #27326, #20096, #4845 ) ;
#6564=DIRECTION ( 'NONE',  ( 1.000000000000000000, 0.000000000000000000, 0.000000000000000000 ) ) ;
#6572=ADVANCED_FACE ( 'NONE', ( #18842 ), #31022, .F. ) ;
#6574=DIRECTION ( 'NONE',  ( -1.101824276508909887E-16, 1.000000000000000000, -0.000000000000000000 ) ) ;
#6581=CARTESIAN_POINT ( 'NONE',  ( 21.09992658989239089, 26.96183152705960495, 47.04930799450051637 ) ) ;
#6583=DIRECTION ( 'NONE',  ( -1.101824276508909887E-16, 1.000000000000000000, -0.000000000000000000 ) ) ;
#6584=AXIS2_PLACEMENT_3D ( 'NONE', #24732, #19473, #17165 ) ;
#6592=DIRECTION ( 'NONE',  ( -1.101824276508909887E-16, 1.000000000000000000, -0.000000000000000000 ) ) ;
#6594=EDGE_CURVE ( 'NONE', #30310, #22128, #27703, .T. ) ;
#6595=EDGE_CURVE ( 'NONE', #31343, #29220, #13620, .T. ) ;
#6598=DIRECTION ( 'NONE',  ( 0.000000000000000000, -0.000000000000000000, -1.000000000000000000 ) ) ;
#6605=ADVANCED_FACE ( 'NONE', ( #3925 ), #13546, .T. ) ;
#6607=DIRECTION ( 'NONE',  ( -1.101824276508909887E-16, 1.000000000000000000, -0.000000000000000000 ) ) ;
#6614=ORIENTED_EDGE ( 'NONE', *, *, #7576, .F. ) ;
#6618=DIRECTION ( 'NONE',  ( 1.000000000000000000, 0.000000000000000000, 0.000000000000000000 ) ) ;
#6624=DIRECTION ( 'NONE',  ( -1.000000000000000000, -1.101824276508909887E-16, 0.000000000000000000 ) ) ;
#6628=CARTESIAN_POINT ( 'NONE',  ( 33.71785032049135111, 27.21664230456639899, 47.04930799450051637 ) ) ;
#6633=CARTESIAN_POINT ( 'NONE',  ( 8.732853799281738105, 26.96183152705960495, 47.04930799450051637 ) ) ;
#6635=AXIS2_PLACEMENT_3D ( 'NONE', #6870, #28870, #13937 ) ;
#6642=CIRCLE ( 'NONE', #869, 12.27641737965282687 ) ;
#6644=DIRECTION ( 'NONE',  ( -1.000000000000000000, 0.000000000000000000, 0.000000000000000000 ) ) ;
#6645=ORIENTED_EDGE ( 'NONE', *, *, #8890, .F. ) ;
#6646=CARTESIAN_POINT ( 'NONE',  ( 33.72499318558949710, 30.09143805560860585, 47.04930799450051637 ) ) ;
#6655=ORIENTED_EDGE ( 'NONE', *, *, #29004, .T. ) ;
#6658=LINE ( 'NONE', #1561, #22079 ) ;
#6659=DIRECTION ( 'NONE',  ( -1.000000000000000000, 0.000000000000000000, 0.000000000000000000 ) ) ;
#6664=EDGE_CURVE ( 'NONE', #15469, #30180, #32437, .T. ) ;
#6666=FACE_OUTER_BOUND ( 'NONE', #1695, .T. ) ;
#6672=ORIENTED_EDGE ( 'NONE', *, *, #23092, .T. ) ;
#6673=ADVANCED_FACE ( 'NONE', ( #15194 ), #31913, .T. ) ;
#6675=AXIS2_PLACEMENT_3D ( 'NONE', #13816, #15618, #18403 ) ;
#6679=VERTEX_POINT ( 'NONE', #10116 ) ;
#6683=CARTESIAN_POINT ( 'NONE',  ( 21.09992658989239089, 30.46183152705961561, 47.04930799450051637 ) ) ;
#6685=EDGE_LOOP ( 'NONE', ( #13660, #11027, #1657, #16407 ) ) ;
#6686=DIRECTION ( 'NONE',  ( -1.101824276508909887E-16, 1.000000000000000000, -0.000000000000000000 ) ) ;
#6691=CARTESIAN_POINT ( 'NONE',  ( 8.698509210239526723, 26.09164230456639899, 47.04930799450051637 ) ) ;
#6697=EDGE_LOOP ( 'NONE', ( #25460, #21704, #6347, #20153 ) ) ;
#6699=DIRECTION ( 'NONE',  ( 0.000000000000000000, -0.000000000000000000, -1.000000000000000000 ) ) ;
#6703=FACE_OUTER_BOUND ( 'NONE', #13449, .T. ) ;
#6707=EDGE_LOOP ( 'NONE', ( #11496, #24901, #19577, #19952 ) ) ;
#6713=EDGE_CURVE ( 'NONE', #27697, #19462, #11475, .T. ) ;
#6714=ADVANCED_FACE ( 'NONE', ( #11645 ), #21638, .T. ) ;
#6720=ORIENTED_EDGE ( 'NONE', *, *, #25059, .T. ) ;
#6723=CIRCLE ( 'NONE', #25083, 0.1250000000000001110 ) ;
#6726=ORIENTED_EDGE ( 'NONE', *, *, #32113, .F. ) ;
#6728=ORIENTED_EDGE ( 'NONE', *, *, #521, .T. ) ;
#6731=CARTESIAN_POINT ( 'NONE',  ( 8.698509210239521394, 25.59164230456639899, 47.04930799450051637 ) ) ;
#6734=ORIENTED_EDGE ( 'NONE', *, *, #8851, .F. ) ;
#6735=ORIENTED_EDGE ( 'NONE', *, *, #5152, .F. ) ;
#6739=CARTESIAN_POINT ( 'NONE',  ( 21.09992658989238734, 38.56284415653841791, 47.04930799450051637 ) ) ;
#6741=DIRECTION ( 'NONE',  ( -1.000000000000000000, -1.101824276508909764E-16, 0.000000000000000000 ) ) ;
#6744=DIRECTION ( 'NONE',  ( -1.000000000000000000, -1.101824276508909887E-16, 0.000000000000000000 ) ) ;
#6746=CIRCLE ( 'NONE', #22452, 0.1250000000000001110 ) ;
#6755=CARTESIAN_POINT ( 'NONE',  ( 21.09992658989238734, 38.56284415653841791, 47.04930799450051637 ) ) ;
#6759=EDGE_LOOP ( 'NONE', ( #623, #22827, #20146, #28642 ) ) ;
#6760=DIRECTION ( 'NONE',  ( -1.000000000000000000, -1.101824276508909887E-16, 0.000000000000000000 ) ) ;
#6770=DIRECTION ( 'NONE',  ( -1.101824276508909887E-16, 1.000000000000000000, -0.000000000000000000 ) ) ;
#6773=FACE_OUTER_BOUND ( 'NONE', #13650, .T. ) ;
#6778=CARTESIAN_POINT ( 'NONE',  ( 33.72499318558949710, 26.84143805560860940, 47.04930799450051637 ) ) ;
#6783=CARTESIAN_POINT ( 'NONE',  ( 33.72499318558949710, 26.34184655352419213, 47.04930799450051637 ) ) ;
#6785=ORIENTED_EDGE ( 'NONE', *, *, #6390, .T. ) ;
#6788=CARTESIAN_POINT ( 'NONE',  ( 8.698509210239574685, 31.09164230456639544, 47.04930799450051637 ) ) ;
#6790=ORIENTED_EDGE ( 'NONE', *, *, #7723, .F. ) ;
#6794=VECTOR ( 'NONE', #22584, 1000.000000000000000 ) ;
#6796=ORIENTED_EDGE ( 'NONE', *, *, #18887, .T. ) ;
#6799=AXIS2_PLACEMENT_3D ( 'NONE', #7115, #17113, #27134 ) ;
#6800=AXIS2_PLACEMENT_3D ( 'NONE', #2440, #25086, #3069 ) ;
#6806=EDGE_CURVE ( 'NONE', #1229, #8522, #15994, .T. ) ;
#6807=VERTEX_POINT ( 'NONE', #576 ) ;
#6810=CARTESIAN_POINT ( 'NONE',  ( 33.50134396954526750, 24.59164230456639544, 47.04930799450051637 ) ) ;
#6816=DIRECTION ( 'NONE',  ( -1.000000000000000000, -1.101824276508909887E-16, 0.000000000000000000 ) ) ;
#6817=CIRCLE ( 'NONE', #29360, 0.1250000000000001110 ) ;
#6824=ORIENTED_EDGE ( 'NONE', *, *, #13469, .F. ) ;
#6826=DIRECTION ( 'NONE',  ( -1.000000000000000000, -1.101824276508909887E-16, 0.000000000000000000 ) ) ;
#6830=AXIS2_PLACEMENT_3D ( 'NONE', #18691, #9186, #16714 ) ;
#6831=CARTESIAN_POINT ( 'NONE',  ( 33.37634396954525329, 26.09164230456639899, 47.04930799450051637 ) ) ;
#6832=ORIENTED_EDGE ( 'NONE', *, *, #29808, .T. ) ;
#6833=AXIS2_PLACEMENT_3D ( 'NONE', #25311, #17917, #352 ) ;
#6834=ORIENTED_EDGE ( 'NONE', *, *, #18561, .T. ) ;
#6841=ADVANCED_FACE ( 'NONE', ( #22899 ), #7292, .T. ) ;
#6845=ORIENTED_EDGE ( 'NONE', *, *, #8974, .T. ) ;
#6851=CARTESIAN_POINT ( 'NONE',  ( 8.474859994195286461, 24.34143805560860940, 47.04930799450051637 ) ) ;
#6853=AXIS2_PLACEMENT_3D ( 'NONE', #17991, #12923, #22912 ) ;
#6854=EDGE_LOOP ( 'NONE', ( #29889, #8246, #1811, #11190 ) ) ;
#6856=EDGE_LOOP ( 'NONE', ( #853, #23700, #1647, #17755 ) ) ;
#6860=ORIENTED_EDGE ( 'NONE', *, *, #10274, .T. ) ;
#6863=CYLINDRICAL_SURFACE ( 'NONE', #14683, 12.36707279061065101 ) ;
#6865=DIRECTION ( 'NONE',  ( -1.224646799147353207E-16, -1.349345573449484691E-32, 1.000000000000000000 ) ) ;
#6870=CARTESIAN_POINT ( 'NONE',  ( 21.09992658989238734, 38.56284415653841791, 47.04930799450051637 ) ) ;
#6871=DIRECTION ( 'NONE',  ( -1.000000000000000000, 0.000000000000000000, 0.000000000000000000 ) ) ;
#6872=CIRCLE ( 'NONE', #28365, 12.62506659569710266 ) ;
#6873=DIRECTION ( 'NONE',  ( -1.000000000000000000, 0.000000000000000000, 0.000000000000000000 ) ) ;
#6879=DIRECTION ( 'NONE',  ( -1.000000000000000000, -1.101824276508909887E-16, 0.000000000000000000 ) ) ;
#6885=ORIENTED_EDGE ( 'NONE', *, *, #31431, .T. ) ;
#6893=LINE ( 'NONE', #16894, #26332 ) ;
#6894=ORIENTED_EDGE ( 'NONE', *, *, #24233, .T. ) ;
#6895=ORIENTED_EDGE ( 'NONE', *, *, #25491, .F. ) ;
#6896=EDGE_CURVE ( 'NONE', #7848, #154, #9377, .T. ) ;
#6897=ORIENTED_EDGE ( 'NONE', *, *, #7458, .T. ) ;
#6900=DIRECTION ( 'NONE',  ( -1.000000000000000000, 0.000000000000000000, 0.000000000000000000 ) ) ;
#6904=ORIENTED_EDGE ( 'NONE', *, *, #18446, .T. ) ;
#6908=VERTEX_POINT ( 'NONE', #18452 ) ;
#6910=VERTEX_POINT ( 'NONE', #5992 ) ;
#6914=CYLINDRICAL_SURFACE ( 'NONE', #15919, 12.36707279061065101 ) ;
#6916=AXIS2_PLACEMENT_3D ( 'NONE', #3343, #30449, #31088 ) ;
#6919=FACE_OUTER_BOUND ( 'NONE', #15988, .T. ) ;
#6921=DIRECTION ( 'NONE',  ( -1.000000000000000000, -1.101824276508909887E-16, 0.000000000000000000 ) ) ;
#6925=CIRCLE ( 'NONE', #25290, 12.62506659569710266 ) ;
#6927=DIRECTION ( 'NONE',  ( -1.101824276508909887E-16, 1.000000000000000000, -0.000000000000000000 ) ) ;
#6928=DIRECTION ( 'NONE',  ( -1.000000000000000000, -1.101824276508909887E-16, 0.000000000000000000 ) ) ;
#6934=CIRCLE ( 'NONE', #25291, 0.1250000000000001110 ) ;
#6938=EDGE_LOOP ( 'NONE', ( #15090, #9621, #31171, #9096 ) ) ;
#6944=ORIENTED_EDGE ( 'NONE', *, *, #28841, .T. ) ;
#6948=FACE_OUTER_BOUND ( 'NONE', #32005, .T. ) ;
#6957=EDGE_LOOP ( 'NONE', ( #27657, #22779, #12673, #6944 ) ) ;
#6958=ORIENTED_EDGE ( 'NONE', *, *, #25491, .T. ) ;
#6959=AXIS2_PLACEMENT_3D ( 'NONE', #29181, #6865, #19155 ) ;
#6966=CARTESIAN_POINT ( 'NONE',  ( 8.474859994195281132, 31.84143805560860940, 47.04930799450051637 ) ) ;
#6967=CARTESIAN_POINT ( 'NONE',  ( 21.09992658989239089, 24.09184655352419213, 47.04930799450051637 ) ) ;
#6977=CARTESIAN_POINT ( 'NONE',  ( 33.72499318558949000, 38.56284415653841791, 47.04930799450051637 ) ) ;
#6982=DIRECTION ( 'NONE',  ( -1.101824276508909887E-16, 1.000000000000000000, -0.000000000000000000 ) ) ;
#6985=ORIENTED_EDGE ( 'NONE', *, *, #19979, .F. ) ;
#6987=CARTESIAN_POINT ( 'NONE',  ( 21.09992658989238734, 38.56284415653841791, 47.04930799450051637 ) ) ;
#6989=DIRECTION ( 'NONE',  ( -1.000000000000000000, -1.101824276508909887E-16, 0.000000000000000000 ) ) ;
#6994=EDGE_CURVE ( 'NONE', #8369, #12497, #24183, .T. ) ;
#7001=FACE_OUTER_BOUND ( 'NONE', #28482, .T. ) ;
#7005=AXIS2_PLACEMENT_3D ( 'NONE', #22559, #248, #89 ) ;
#7009=DIRECTION ( 'NONE',  ( -1.101824276508909887E-16, 1.000000000000000000, -0.000000000000000000 ) ) ;
#7012=EDGE_LOOP ( 'NONE', ( #12862, #9503, #20635, #6985 ) ) ;
#7013=DIRECTION ( 'NONE',  ( -1.000000000000000000, 0.000000000000000000, 0.000000000000000000 ) ) ;
#7021=CARTESIAN_POINT ( 'NONE',  ( 21.09992658989239089, 26.46183152705960140, 47.04930799450051637 ) ) ;
#7028=CARTESIAN_POINT ( 'NONE',  ( 21.09992658989238734, 38.56284415653841791, 47.04930799450051637 ) ) ;
#7029=LINE ( 'NONE', #7193, #4841 ) ;
#7031=EDGE_LOOP ( 'NONE', ( #5354, #7973, #24362, #9616 ) ) ;
#7034=VERTEX_POINT ( 'NONE', #6633 ) ;
#7035=CARTESIAN_POINT ( 'NONE',  ( 21.09992658989239089, 28.34143805560861296, 47.04930799450051637 ) ) ;
#7038=EDGE_CURVE ( 'NONE', #10115, #7900, #1507, .T. ) ;
#7039=EDGE_CURVE ( 'NONE', #20933, #20144, #16186, .T. ) ;
#7040=ORIENTED_EDGE ( 'NONE', *, *, #3021, .F. ) ;
#7041=CARTESIAN_POINT ( 'NONE',  ( 21.09992658989239089, 24.21183152705959785, 47.04930799450051637 ) ) ;
#7042=FACE_OUTER_BOUND ( 'NONE', #10643, .T. ) ;
#7044=ORIENTED_EDGE ( 'NONE', *, *, #19696, .F. ) ;
#7047=AXIS2_PLACEMENT_3D ( 'NONE', #1471, #11489, #30720 ) ;
#7051=EDGE_LOOP ( 'NONE', ( #1579, #28415, #29978, #19054 ) ) ;
#7052=ORIENTED_EDGE ( 'NONE', *, *, #4157, .F. ) ;
#7054=CARTESIAN_POINT ( 'NONE',  ( 33.50134396954522487, 29.09164230456639899, 47.04930799450051637 ) ) ;
#7055=VECTOR ( 'NONE', #30217, 1000.000000000000000 ) ;
#7060=DIRECTION ( 'NONE',  ( -1.000000000000000000, 0.000000000000000000, 0.000000000000000000 ) ) ;
#7063=ORIENTED_EDGE ( 'NONE', *, *, #4627, .T. ) ;
#7064=ORIENTED_EDGE ( 'NONE', *, *, #4371, .F. ) ;
#7065=DIRECTION ( 'NONE',  ( -1.224646799147353207E-16, -1.349345573449484691E-32, 1.000000000000000000 ) ) ;
#7072=ORIENTED_EDGE ( 'NONE', *, *, #5793, .T. ) ;
#7075=DIRECTION ( 'NONE',  ( -1.000000000000000000, 0.000000000000000000, 0.000000000000000000 ) ) ;
#7076=AXIS2_PLACEMENT_3D ( 'NONE', #24647, #22176, #32204 ) ;
#7078=CIRCLE ( 'NONE', #26475, 12.62506659569710266 ) ;
#7085=DIRECTION ( 'NONE',  ( -1.101824276508909887E-16, 1.000000000000000000, -0.000000000000000000 ) ) ;
#7091=DIRECTION ( 'NONE',  ( -1.224646799147353207E-16, -1.349345573449484691E-32, 1.000000000000000000 ) ) ;
#7092=FACE_OUTER_BOUND ( 'NONE', #10589, .T. ) ;
#7102=CIRCLE ( 'NONE', #16527, 12.62506659569710266 ) ;
#7108=CARTESIAN_POINT ( 'NONE',  ( 21.09992658989239089, 28.71183152705961206, 47.04930799450051637 ) ) ;
#7115=CARTESIAN_POINT ( 'NONE',  ( 8.698509210239503631, 23.84164230456639544, 47.04930799450051637 ) ) ;
#7120=EDGE_CURVE ( 'NONE', #10702, #321, #18796, .T. ) ;
#7124=EDGE_CURVE ( 'NONE', #7136, #14930, #4136, .T. ) ;
#7127=EDGE_CURVE ( 'NONE', #16912, #27697, #12419, .T. ) ;
#7128=AXIS2_PLACEMENT_3D ( 'NONE', #6581, #29223, #1972 ) ;
#7130=ORIENTED_EDGE ( 'NONE', *, *, #20443, .T. ) ;
#7136=VERTEX_POINT ( 'NONE', #219 ) ;
#7142=DIRECTION ( 'NONE',  ( -1.101824276508909887E-16, 1.000000000000000000, -0.000000000000000000 ) ) ;
#7150=ORIENTED_EDGE ( 'NONE', *, *, #25244, .T. ) ;
#7152=EDGE_CURVE ( 'NONE', #22214, #21573, #11887, .T. ) ;
#7158=ORIENTED_EDGE ( 'NONE', *, *, #5, .F. ) ;
#7160=EDGE_CURVE ( 'NONE', #20645, #4648, #17613, .T. ) ;
#7161=EDGE_CURVE ( 'NONE', #4474, #27343, #13472, .T. ) ;
#7162=DIRECTION ( 'NONE',  ( -1.000000000000000000, 0.000000000000000000, 0.000000000000000000 ) ) ;
#7167=CARTESIAN_POINT ( 'NONE',  ( 33.72499318558949000, 38.56284415653841791, 47.04930799450051637 ) ) ;
#7170=DIRECTION ( 'NONE',  ( -1.101824276508909887E-16, 1.000000000000000000, -0.000000000000000000 ) ) ;
#7177=DIRECTION ( 'NONE',  ( 0.000000000000000000, -0.000000000000000000, -1.000000000000000000 ) ) ;
#7180=CARTESIAN_POINT ( 'NONE',  ( 21.09992658989239089, 27.96183152705961206, 47.04930799450051637 ) ) ;
#7181=CARTESIAN_POINT ( 'NONE',  ( 8.732853799281734553, 38.56284415653841791, 47.04930799450051637 ) ) ;
#7185=DIRECTION ( 'NONE',  ( -1.101824276508909887E-16, 1.000000000000000000, -0.000000000000000000 ) ) ;
#7188=DIRECTION ( 'NONE',  ( -1.224646799147353207E-16, -1.349345573449484691E-32, 1.000000000000000000 ) ) ;
#7189=ADVANCED_FACE ( 'NONE', ( #25333 ), #24994, .T. ) ;
#7193=CARTESIAN_POINT ( 'NONE',  ( 8.474859994195282908, 38.56284415653841791, 47.04930799450051637 ) ) ;
#7194=CARTESIAN_POINT ( 'NONE',  ( 8.732853799281736329, 25.47145308207319303, 47.04930799450051637 ) ) ;
#7199=ORIENTED_EDGE ( 'NONE', *, *, #15196, .T. ) ;
#7200=CIRCLE ( 'NONE', #25034, 12.36707279061065279 ) ;
#7201=EDGE_CURVE ( 'NONE', #12012, #11938, #4552, .T. ) ;
#7206=ORIENTED_EDGE ( 'NONE', *, *, #13825, .T. ) ;
#7207=DIRECTION ( 'NONE',  ( -1.000000000000000000, 0.000000000000000000, 0.000000000000000000 ) ) ;
#7208=DIRECTION ( 'NONE',  ( -1.000000000000000000, 0.000000000000000000, 0.000000000000000000 ) ) ;
#7218=EDGE_CURVE ( 'NONE', #8103, #14337, #31804, .T. ) ;
#7220=CYLINDRICAL_SURFACE ( 'NONE', #13920, 12.36707279061065101 ) ;
#7222=CIRCLE ( 'NONE', #5112, 0.1250000000000001110 ) ;
#7226=ORIENTED_EDGE ( 'NONE', *, *, #25212, .T. ) ;
#7228=DIRECTION ( 'NONE',  ( -1.000000000000000000, -1.101824276508909887E-16, 0.000000000000000000 ) ) ;
#7229=ADVANCED_FACE ( 'NONE', ( #7393 ), #8727, .T. ) ;
#7233=EDGE_CURVE ( 'NONE', #26085, #27014, #7699, .T. ) ;
#7243=AXIS2_PLACEMENT_3D ( 'NONE', #11468, #19167, #13781 ) ;
#7260=FACE_OUTER_BOUND ( 'NONE', #6685, .T. ) ;
#7264=FACE_OUTER_BOUND ( 'NONE', #19843, .T. ) ;
#7268=EDGE_LOOP ( 'NONE', ( #3605, #97, #2402, #30742 ) ) ;
#7269=DIRECTION ( 'NONE',  ( -1.101824276508909887E-16, 1.000000000000000000, -0.000000000000000000 ) ) ;
#7270=AXIS2_PLACEMENT_3D ( 'NONE', #23716, #1221, #11248 ) ;
#7274=VECTOR ( 'NONE', #8847, 1000.000000000000000 ) ;
#7280=LINE ( 'NONE', #17766, #13104 ) ;
#7281=TOROIDAL_SURFACE ( 'NONE', #25611, 12.40141737965285706, 0.1250000000000007494 ) ;
#7282=VERTEX_POINT ( 'NONE', #32173 ) ;
#7285=CARTESIAN_POINT ( 'NONE',  ( 33.50134396954519644, 31.09164230456639544, 47.04930799450051637 ) ) ;
#7286=CARTESIAN_POINT ( 'NONE',  ( 33.72499318558949000, 38.56284415653841791, 47.04930799450051637 ) ) ;
#7290=EDGE_LOOP ( 'NONE', ( #6033, #24864, #15076, #20773 ) ) ;
#7292=TOROIDAL_SURFACE ( 'NONE', #25125, 12.61792373059860495, 0.1250000000000008604 ) ;
#7295=CARTESIAN_POINT ( 'NONE',  ( 21.09992658989239089, 26.21664230456639899, 47.04930799450051637 ) ) ;
#7296=CARTESIAN_POINT ( 'NONE',  ( 33.72499318558949710, 26.84184655352419568, 47.04930799450051637 ) ) ;
#7297=ORIENTED_EDGE ( 'NONE', *, *, #4903, .F. ) ;
#7302=TOROIDAL_SURFACE ( 'NONE', #1525, 12.61792373059898686, 0.1249999999999964195 ) ;
#7307=DIRECTION ( 'NONE',  ( -1.000000000000000000, 0.000000000000000000, 0.000000000000000000 ) ) ;
#7308=CARTESIAN_POINT ( 'NONE',  ( 21.09992658989238734, 30.84164230456639544, 47.04930799450051637 ) ) ;
#7309=DIRECTION ( 'NONE',  ( -1.000000000000000000, -1.101824276508909887E-16, 0.000000000000000000 ) ) ;
#7310=EDGE_CURVE ( 'NONE', #3444, #20933, #25503, .T. ) ;
#7311=CARTESIAN_POINT ( 'NONE',  ( 21.09992658989239089, 24.84164230456639544, 47.04930799450051637 ) ) ;
#7316=ORIENTED_EDGE ( 'NONE', *, *, #5412, .T. ) ;
#7321=ORIENTED_EDGE ( 'NONE', *, *, #11634, .T. ) ;
#7323=VECTOR ( 'NONE', #27621, 1000.000000000000000 ) ;
#7324=CIRCLE ( 'NONE', #6799, 0.1250000000000001110 ) ;
#7326=AXIS2_PLACEMENT_3D ( 'NONE', #2107, #29529, #6879 ) ;
#7329=AXIS2_PLACEMENT_3D ( 'NONE', #29958, #12066, #30119 ) ;
#7333=DIRECTION ( 'NONE',  ( -1.101824276508909887E-16, 1.000000000000000000, -0.000000000000000000 ) ) ;
#7338=ORIENTED_EDGE ( 'NONE', *, *, #32176, .T. ) ;
#7339=DIRECTION ( 'NONE',  ( -1.224646799147353207E-16, -1.349345573449484691E-32, 1.000000000000000000 ) ) ;
#7342=FACE_OUTER_BOUND ( 'NONE', #7492, .T. ) ;
#7345=CARTESIAN_POINT ( 'NONE',  ( 33.50134396954523908, 27.34164230456639544, 47.04930799450051637 ) ) ;
#7346=CIRCLE ( 'NONE', #17288, 0.1249999999999983763 ) ;
#7352=EDGE_CURVE ( 'NONE', #15557, #14283, #20039, .T. ) ;
#7353=VECTOR ( 'NONE', #3980, 1000.000000000000000 ) ;
#7369=DIRECTION ( 'NONE',  ( 1.000000000000000000, 0.000000000000000000, 0.000000000000000000 ) ) ;
#7371=ORIENTED_EDGE ( 'NONE', *, *, #10587, .F. ) ;
#7372=CIRCLE ( 'NONE', #28845, 12.36707279061065101 ) ;
#7376=AXIS2_PLACEMENT_3D ( 'NONE', #11746, #6982, #26843 ) ;
#7379=EDGE_CURVE ( 'NONE', #19462, #31503, #28134, .T. ) ;
#7380=CARTESIAN_POINT ( 'NONE',  ( 21.09992658989239089, 25.34164230456639899, 47.04930799450051637 ) ) ;
#7382=CIRCLE ( 'NONE', #17850, 12.36707279061065101 ) ;
#7383=ORIENTED_EDGE ( 'NONE', *, *, #20755, .F. ) ;
#7385=DIRECTION ( 'NONE',  ( -1.101824276508909887E-16, 1.000000000000000000, -0.000000000000000000 ) ) ;
#7390=DIRECTION ( 'NONE',  ( -1.101824276508909887E-16, 1.000000000000000000, -0.000000000000000000 ) ) ;
#7391=TOROIDAL_SURFACE ( 'NONE', #59, 12.40141737965283220, 0.1250000000000002498 ) ;
#7393=FACE_OUTER_BOUND ( 'NONE', #6697, .T. ) ;
#7396=CARTESIAN_POINT ( 'NONE',  ( 8.732853799281734553, 38.56284415653841791, 47.04930799450051637 ) ) ;
#7404=CYLINDRICAL_SURFACE ( 'NONE', #10965, 12.36707279061065101 ) ;
#7407=VECTOR ( 'NONE', #17843, 1000.000000000000000 ) ;
#7411=DIRECTION ( 'NONE',  ( 0.000000000000000000, -0.000000000000000000, -1.000000000000000000 ) ) ;
#7418=ADVANCED_FACE ( 'NONE', ( #22172 ), #26551, .T. ) ;
#7419=CARTESIAN_POINT ( 'NONE',  ( 33.37634396954518934, 32.09164230456639899, 47.04930799450051637 ) ) ;
#7428=TOROIDAL_SURFACE ( 'NONE', #20808, 12.61792373059859607, 0.1249999999999979738 ) ;
#7429=DIRECTION ( 'NONE',  ( -1.101824276508909887E-16, 1.000000000000000000, -0.000000000000000000 ) ) ;
#7431=CARTESIAN_POINT ( 'NONE',  ( 21.09992658989238734, 31.72145308207317171, 47.04930799450051637 ) ) ;
#7436=DIRECTION ( 'NONE',  ( -1.101824276508909887E-16, 1.000000000000000000, -0.000000000000000000 ) ) ;
#7440=DIRECTION ( 'NONE',  ( -1.101824276508909887E-16, 1.000000000000000000, -0.000000000000000000 ) ) ;
#7442=CARTESIAN_POINT ( 'NONE',  ( 33.72499318558949710, 28.34184655352419213, 47.04930799450051637 ) ) ;
#7444=ORIENTED_EDGE ( 'NONE', *, *, #2119, .T. ) ;
#7449=ORIENTED_EDGE ( 'NONE', *, *, #16659, .T. ) ;
#7456=ORIENTED_EDGE ( 'NONE', *, *, #4334, .T. ) ;
#7458=EDGE_CURVE ( 'NONE', #18578, #13589, #14518, .T. ) ;
#7459=ORIENTED_EDGE ( 'NONE', *, *, #30696, .F. ) ;
#7460=DIRECTION ( 'NONE',  ( -1.101824276508909887E-16, 1.000000000000000000, -0.000000000000000000 ) ) ;
#7461=TOROIDAL_SURFACE ( 'NONE', #18454, 12.40141737965283575, 0.1250000000000000278 ) ;
#7462=EDGE_CURVE ( 'NONE', #13441, #19026, #6642, .T. ) ;
#7463=ORIENTED_EDGE ( 'NONE', *, *, #31023, .T. ) ;
#7464=EDGE_CURVE ( 'NONE', #29193, #21016, #9264, .T. ) ;
#7469=VERTEX_POINT ( 'NONE', #7419 ) ;
#7474=CIRCLE ( 'NONE', #28951, 0.1250000000000001110 ) ;
#7475=DIRECTION ( 'NONE',  ( -1.000000000000000000, 0.000000000000000000, 0.000000000000000000 ) ) ;
#7480=CARTESIAN_POINT ( 'NONE',  ( 21.09992658989239089, 28.47145308207318237, 47.04930799450051637 ) ) ;
#7482=EDGE_LOOP ( 'NONE', ( #14120, #15995, #8755, #21664 ) ) ;
#7483=DIRECTION ( 'NONE',  ( -1.101824276508909887E-16, 1.000000000000000000, -0.000000000000000000 ) ) ;
#7486=CARTESIAN_POINT ( 'NONE',  ( 21.09992658989239089, 24.09164230456639544, 47.04930799450051637 ) ) ;
#7487=CARTESIAN_POINT ( 'NONE',  ( 33.71785032049099584, 30.21664230456641675, 47.04930799450051637 ) ) ;
#7492=EDGE_LOOP ( 'NONE', ( #14636, #27706, #30064, #12888 ) ) ;
#7493=CIRCLE ( 'NONE', #25815, 12.51969897791880015 ) ;
#7496=ORIENTED_EDGE ( 'NONE', *, *, #3846, .F. ) ;
#7497=CIRCLE ( 'NONE', #8033, 12.27641737965283042 ) ;
#7498=ADVANCED_FACE ( 'NONE', ( #10852 ), #26037, .T. ) ;
#7500=EDGE_LOOP ( 'NONE', ( #26278, #14223, #12913, #14935 ) ) ;
#7503=CIRCLE ( 'NONE', #21114, 12.36707279061065279 ) ;
#7505=DIRECTION ( 'NONE',  ( -1.101824276508909887E-16, 1.000000000000000000, -0.000000000000000000 ) ) ;
#7506=CARTESIAN_POINT ( 'NONE',  ( 8.474859994195282908, 38.56284415653841791, 47.04930799450051637 ) ) ;
#7507=AXIS2_PLACEMENT_3D ( 'NONE', #3254, #30835, #8344 ) ;
#7508=DIRECTION ( 'NONE',  ( -1.000000000000000000, 0.000000000000000000, 0.000000000000000000 ) ) ;
#7509=EDGE_LOOP ( 'NONE', ( #29783, #23717, #16279, #30594 ) ) ;
#7511=EDGE_LOOP ( 'NONE', ( #14350, #16464, #523, #30144 ) ) ;
#7516=CARTESIAN_POINT ( 'NONE',  ( 8.698509210239517842, 25.34164230456639899, 47.04930799450051637 ) ) ;
#7523=DIRECTION ( 'NONE',  ( -1.101824276508909887E-16, 1.000000000000000000, -0.000000000000000000 ) ) ;
#7527=ORIENTED_EDGE ( 'NONE', *, *, #49, .T. ) ;
#7529=EDGE_LOOP ( 'NONE', ( #14736, #11136, #3751, #6824 ) ) ;
#7530=EDGE_LOOP ( 'NONE', ( #10527, #10428, #20939, #19662 ) ) ;
#7533=AXIS2_PLACEMENT_3D ( 'NONE', #7021, #32303, #9977 ) ;
#7536=AXIS2_PLACEMENT_3D ( 'NONE', #28782, #21707, #6624 ) ;
#7537=EDGE_CURVE ( 'NONE', #3694, #29832, #22983, .T. ) ;
#7541=ORIENTED_EDGE ( 'NONE', *, *, #17454, .T. ) ;
#7543=ADVANCED_FACE ( 'NONE', ( #17904 ), #2978, .T. ) ;
#7553=ORIENTED_EDGE ( 'NONE', *, *, #31181, .F. ) ;
#7554=FACE_OUTER_BOUND ( 'NONE', #15412, .T. ) ;
#7555=CARTESIAN_POINT ( 'NONE',  ( 21.09992658989239089, 26.96183152705960495, 47.04930799450051637 ) ) ;
#7557=CARTESIAN_POINT ( 'NONE',  ( 21.09992658989238734, 32.54735957529758394, 47.04930799450051637 ) ) ;
#7560=CARTESIAN_POINT ( 'NONE',  ( 8.698509210239549816, 28.34164230456639544, 47.04930799450051637 ) ) ;
#7561=DIRECTION ( 'NONE',  ( -1.101824276508909887E-16, 1.000000000000000000, -0.000000000000000000 ) ) ;
#7564=ORIENTED_EDGE ( 'NONE', *, *, #5127, .F. ) ;
#7567=DIRECTION ( 'NONE',  ( -1.101824276508909887E-16, 1.000000000000000000, -0.000000000000000000 ) ) ;
#7571=ORIENTED_EDGE ( 'NONE', *, *, #22901, .T. ) ;
#7572=TOROIDAL_SURFACE ( 'NONE', #22785, 12.61792373059893713, 0.1249999999999992506 ) ;
#7576=EDGE_CURVE ( 'NONE', #2178, #27701, #23373, .T. ) ;
#7578=CARTESIAN_POINT ( 'NONE',  ( 21.09992658989239089, 24.96664230456639899, 47.04930799450051637 ) ) ;
#7584=DIRECTION ( 'NONE',  ( -1.101824276508909887E-16, 1.000000000000000000, -0.000000000000000000 ) ) ;
#7586=DIRECTION ( 'NONE',  ( -1.101824276508909887E-16, 1.000000000000000000, -0.000000000000000000 ) ) ;
#7588=DIRECTION ( 'NONE',  ( -1.101824276508909887E-16, 1.000000000000000000, -0.000000000000000000 ) ) ;
#7597=LINE ( 'NONE', #2342, #3964 ) ;
#7598=DIRECTION ( 'NONE',  ( -1.000000000000000000, -1.101824276508909887E-16, 0.000000000000000000 ) ) ;
#7604=CARTESIAN_POINT ( 'NONE',  ( 21.09992658989239089, 23.59164230456639544, 47.04930799450051637 ) ) ;
#7606=VERTEX_POINT ( 'NONE', #5595 ) ;
#7611=EDGE_CURVE ( 'NONE', #4901, #11910, #18619, .T. ) ;
#7613=EDGE_CURVE ( 'NONE', #26283, #17205, #6081, .T. ) ;
#7616=DIRECTION ( 'NONE',  ( 1.000000000000000000, 0.000000000000000000, 0.000000000000000000 ) ) ;
#7618=CARTESIAN_POINT ( 'NONE',  ( 8.698509210239580014, 31.59164230456639544, 47.04930799450051637 ) ) ;
#7622=VERTEX_POINT ( 'NONE', #13475 ) ;
#7624=CARTESIAN_POINT ( 'NONE',  ( 21.09992658989239089, 27.34164230456639544, 47.04930799450051637 ) ) ;
#7625=CARTESIAN_POINT ( 'NONE',  ( 33.71785032049130137, 31.96664230456639544, 47.04930799450051637 ) ) ;
#7626=CIRCLE ( 'NONE', #24386, 12.36707279061065101 ) ;
#7628=AXIS2_PLACEMENT_3D ( 'NONE', #19760, #2383, #7475 ) ;
#7630=DIRECTION ( 'NONE',  ( -1.101824276508909887E-16, 1.000000000000000000, -0.000000000000000000 ) ) ;
#7632=TOROIDAL_SURFACE ( 'NONE', #30178, 12.40141737965283220, 0.1250000000000002498 ) ;
#7633=CARTESIAN_POINT ( 'NONE',  ( 8.474859994195286461, 26.34143805560860940, 47.04930799450051637 ) ) ;
#7634=CARTESIAN_POINT ( 'NONE',  ( 8.732853799281738105, 29.46183152705961206, 47.04930799450051637 ) ) ;
#7637=CYLINDRICAL_SURFACE ( 'NONE', #31195, 12.62506659569710266 ) ;
#7638=ORIENTED_EDGE ( 'NONE', *, *, #8851, .T. ) ;
#7640=DIRECTION ( 'NONE',  ( -1.000000000000000000, -1.101824276508909887E-16, 0.000000000000000000 ) ) ;
#7642=ADVANCED_FACE ( 'NONE', ( #8857 ), #314, .T. ) ;
#7645=ORIENTED_EDGE ( 'NONE', *, *, #7689, .F. ) ;
#7648=ORIENTED_EDGE ( 'NONE', *, *, #4793, .F. ) ;
#7655=DIRECTION ( 'NONE',  ( -1.000000000000000000, 0.000000000000000000, 0.000000000000000000 ) ) ;
#7658=EDGE_LOOP ( 'NONE', ( #17763, #13388, #21879, #16474 ) ) ;
#7659=CIRCLE ( 'NONE', #24437, 12.36707279061065101 ) ;
#7672=ORIENTED_EDGE ( 'NONE', *, *, #3249, .F. ) ;
#7675=CARTESIAN_POINT ( 'NONE',  ( 8.698509210239539158, 27.34164230456639544, 47.04930799450051637 ) ) ;
#7677=VERTEX_POINT ( 'NONE', #16079 ) ;
#7679=DIRECTION ( 'NONE',  ( 1.000000000000000000, 0.000000000000000000, 0.000000000000000000 ) ) ;
#7680=EDGE_CURVE ( 'NONE', #25242, #28129, #30198, .T. ) ;
#7681=FACE_OUTER_BOUND ( 'NONE', #30454, .T. ) ;
#7682=CARTESIAN_POINT ( 'NONE',  ( 8.474859994195281132, 31.34143805560860585, 47.04930799450051637 ) ) ;
#7685=CARTESIAN_POINT ( 'NONE',  ( 21.09992658989239089, 24.34184655352419213, 47.04930799450051637 ) ) ;
#7686=ORIENTED_EDGE ( 'NONE', *, *, #7233, .T. ) ;
#7689=EDGE_CURVE ( 'NONE', #13790, #1027, #16400, .T. ) ;
#7693=EDGE_LOOP ( 'NONE', ( #1700, #1637, #21075, #9308 ) ) ;
#7696=CIRCLE ( 'NONE', #5586, 12.62506659569710266 ) ;
#7699=CIRCLE ( 'NONE', #27063, 0.1250000000000001110 ) ;
#7706=ORIENTED_EDGE ( 'NONE', *, *, #6439, .T. ) ;
#7709=DIRECTION ( 'NONE',  ( -1.000000000000000000, 0.000000000000000000, 0.000000000000000000 ) ) ;
#7712=DIRECTION ( 'NONE',  ( -1.000000000000000000, 0.000000000000000000, 0.000000000000000000 ) ) ;
#7713=DIRECTION ( 'NONE',  ( 1.000000000000000000, 0.000000000000000000, 0.000000000000000000 ) ) ;
#7716=ORIENTED_EDGE ( 'NONE', *, *, #6713, .F. ) ;
#7719=DIRECTION ( 'NONE',  ( -1.000000000000000000, 0.000000000000000000, 0.000000000000000000 ) ) ;
#7723=EDGE_CURVE ( 'NONE', #29858, #15854, #14476, .T. ) ;
#7726=ORIENTED_EDGE ( 'NONE', *, *, #1538, .T. ) ;
#7736=DIRECTION ( 'NONE',  ( -1.000000000000000000, -1.101824276508909887E-16, 0.000000000000000000 ) ) ;
#7738=EDGE_LOOP ( 'NONE', ( #22970, #3313, #12139, #13491 ) ) ;
#7741=CARTESIAN_POINT ( 'NONE',  ( 8.823509210239574685, 31.34164230456639544, 47.04930799450051637 ) ) ;
#7755=DIRECTION ( 'NONE',  ( -1.224646799147353207E-16, -1.349345573449484691E-32, 1.000000000000000000 ) ) ;
#7757=EDGE_CURVE ( 'NONE', #3066, #30310, #19015, .T. ) ;
#7771=CIRCLE ( 'NONE', #26090, 0.1250000000000001110 ) ;
#7773=DIRECTION ( 'NONE',  ( -1.000000000000000000, 0.000000000000000000, 0.000000000000000000 ) ) ;
#7776=EDGE_LOOP ( 'NONE', ( #13833, #10102, #266, #341 ) ) ;
#7778=ORIENTED_EDGE ( 'NONE', *, *, #3227, .F. ) ;
#7779=FACE_OUTER_BOUND ( 'NONE', #14924, .T. ) ;
#7781=EDGE_CURVE ( 'NONE', #27701, #2178, #5556, .T. ) ;
#7782=CIRCLE ( 'NONE', #26119, 12.36707279061065279 ) ;
#7784=AXIS2_PLACEMENT_3D ( 'NONE', #25935, #29544, #14446 ) ;
#7785=VECTOR ( 'NONE', #4288, 1000.000000000000000 ) ;
#7789=TOROIDAL_SURFACE ( 'NONE', #19294, 12.40141737965281266, 0.1249999999999994865 ) ;
#7790=CARTESIAN_POINT ( 'NONE',  ( 33.46699938050304013, 24.71183152705960140, 47.04930799450051637 ) ) ;
#7793=EDGE_LOOP ( 'NONE', ( #22041, #4773, #15470, #31336 ) ) ;
#7795=DIRECTION ( 'NONE',  ( -1.101824276508909887E-16, 1.000000000000000000, -0.000000000000000000 ) ) ;
#7802=CARTESIAN_POINT ( 'NONE',  ( 8.482002859293395147, 23.96664230456639899, 47.04930799450051637 ) ) ;
#7803=ORIENTED_EDGE ( 'NONE', *, *, #583, .F. ) ;
#7804=DIRECTION ( 'NONE',  ( -1.000000000000000000, 0.000000000000000000, 0.000000000000000000 ) ) ;
#7806=CARTESIAN_POINT ( 'NONE',  ( 21.09992658989239089, 29.21183152705961206, 47.04930799450051637 ) ) ;
#7810=EDGE_LOOP ( 'NONE', ( #1497, #26885, #7199, #15683 ) ) ;
#7811=AXIS2_PLACEMENT_3D ( 'NONE', #26579, #11484, #7207 ) ;
#7820=EDGE_CURVE ( 'NONE', #19596, #25250, #18647, .T. ) ;
#7821=EDGE_CURVE ( 'NONE', #2064, #13790, #23875, .T. ) ;
#7824=ADVANCED_FACE ( 'NONE', ( #7042 ), #26503, .T. ) ;
#7833=DIRECTION ( 'NONE',  ( -1.000000000000000000, 0.000000000000000000, 0.000000000000000000 ) ) ;
#7837=CIRCLE ( 'NONE', #24068, 12.36707279061065101 ) ;
#7840=DIRECTION ( 'NONE',  ( -1.101824276508909887E-16, 1.000000000000000000, -0.000000000000000000 ) ) ;
#7844=DIRECTION ( 'NONE',  ( -1.000000000000000000, 0.000000000000000000, 0.000000000000000000 ) ) ;
#7848=VERTEX_POINT ( 'NONE', #26908 ) ;
#7856=EDGE_CURVE ( 'NONE', #893, #31932, #31229, .T. ) ;
#7857=AXIS2_PLACEMENT_3D ( 'NONE', #23523, #555, #21048 ) ;
#7858=AXIS2_PLACEMENT_3D ( 'NONE', #29893, #4118, #4606 ) ;
#7860=VERTEX_POINT ( 'NONE', #19668 ) ;
#7862=ADVANCED_FACE ( 'NONE', ( #29699 ), #25459, .T. ) ;
#7870=CARTESIAN_POINT ( 'NONE',  ( 8.823509210239549816, 28.34164230456639544, 47.04930799450051637 ) ) ;
#7872=CIRCLE ( 'NONE', #11536, 12.36707279061065101 ) ;
#7875=ORIENTED_EDGE ( 'NONE', *, *, #9157, .T. ) ;
#7876=FACE_OUTER_BOUND ( 'NONE', #7482, .T. ) ;
#7879=DIRECTION ( 'NONE',  ( -1.101824276508909887E-16, 1.000000000000000000, -0.000000000000000000 ) ) ;
#7882=DIRECTION ( 'NONE',  ( -1.101824276508909887E-16, 1.000000000000000000, -0.000000000000000000 ) ) ;
#7884=ORIENTED_EDGE ( 'NONE', *, *, #24255, .T. ) ;
#7886=AXIS2_PLACEMENT_3D ( 'NONE', #1190, #13842, #11370 ) ;
#7888=FACE_OUTER_BOUND ( 'NONE', #30860, .T. ) ;
#7890=EDGE_LOOP ( 'NONE', ( #19502, #2252, #30965, #22226 ) ) ;
#7891=DIRECTION ( 'NONE',  ( -1.000000000000000000, 0.000000000000000000, 0.000000000000000000 ) ) ;
#7893=AXIS2_PLACEMENT_3D ( 'NONE', #8200, #28218, #16056 ) ;
#7894=AXIS2_PLACEMENT_3D ( 'NONE', #23473, #10361, #8544 ) ;
#7900=VERTEX_POINT ( 'NONE', #30633 ) ;
#7902=FACE_OUTER_BOUND ( 'NONE', #18385, .T. ) ;
#7904=CARTESIAN_POINT ( 'NONE',  ( 21.09992658989239089, 27.59143805560860940, 47.04930799450051637 ) ) ;
#7911=CARTESIAN_POINT ( 'NONE',  ( 33.37634396954524618, 26.84164230456639899, 47.04930799450051637 ) ) ;
#7925=DIRECTION ( 'NONE',  ( -1.101824276508909887E-16, 1.000000000000000000, -0.000000000000000000 ) ) ;
#7941=CARTESIAN_POINT ( 'NONE',  ( 8.698509210239507183, 24.09164230456639544, 47.04930799450051637 ) ) ;
#7942=ORIENTED_EDGE ( 'NONE', *, *, #25758, .F. ) ;
#7945=DIRECTION ( 'NONE',  ( -1.101824276508909887E-16, 1.000000000000000000, -0.000000000000000000 ) ) ;
#7946=TOROIDAL_SURFACE ( 'NONE', #26280, 12.40141737965280022, 0.1249999999999992228 ) ;
#7948=VERTEX_POINT ( 'NONE', #23067 ) ;
#7949=EDGE_CURVE ( 'NONE', #14608, #17110, #20768, .T. ) ;
#7950=EDGE_CURVE ( 'NONE', #20619, #24757, #13435, .T. ) ;
#7951=EDGE_CURVE ( 'NONE', #14963, #13965, #7659, .T. ) ;
#7954=ADVANCED_FACE ( 'NONE', ( #23714 ), #11868, .T. ) ;
#7957=DIRECTION ( 'NONE',  ( -1.000000000000000000, 0.000000000000000000, 0.000000000000000000 ) ) ;
#7958=DIRECTION ( 'NONE',  ( -1.000000000000000000, 0.000000000000000000, 0.000000000000000000 ) ) ;
#7959=CARTESIAN_POINT ( 'NONE',  ( 21.09992658989239089, 23.59164230456639544, 47.04930799450051637 ) ) ;
#7962=ORIENTED_EDGE ( 'NONE', *, *, #32323, .T. ) ;
#7966=DIRECTION ( 'NONE',  ( -1.101824276508909887E-16, 1.000000000000000000, -0.000000000000000000 ) ) ;
#7967=AXIS2_PLACEMENT_3D ( 'NONE', #25669, #3012, #21053 ) ;
#7970=CIRCLE ( 'NONE', #16874, 0.1250000000000001110 ) ;
#7973=ORIENTED_EDGE ( 'NONE', *, *, #6236, .F. ) ;
#7975=CARTESIAN_POINT ( 'NONE',  ( 21.09992658989239089, 26.34184655352419213, 47.04930799450051637 ) ) ;
#7976=DIRECTION ( 'NONE',  ( -1.101824276508909887E-16, 1.000000000000000000, -0.000000000000000000 ) ) ;
#7982=AXIS2_PLACEMENT_3D ( 'NONE', #27367, #24742, #17175 ) ;
#7984=TOROIDAL_SURFACE ( 'NONE', #2757, 12.61792373059897621, 0.1249999999999970163 ) ;
#7990=VERTEX_POINT ( 'NONE', #3523 ) ;
#7998=ORIENTED_EDGE ( 'NONE', *, *, #16622, .T. ) ;
#8001=ORIENTED_EDGE ( 'NONE', *, *, #20077, .T. ) ;
#8002=DIRECTION ( 'NONE',  ( -1.000000000000000000, 0.000000000000000000, 0.000000000000000000 ) ) ;
#8005=DIRECTION ( 'NONE',  ( -1.000000000000000000, 0.000000000000000000, 0.000000000000000000 ) ) ;
#8009=CARTESIAN_POINT ( 'NONE',  ( 21.09992658989239089, 30.59164230456639544, 47.04930799450051637 ) ) ;
#8010=ADVANCED_FACE ( 'NONE', ( #18136 ), #12392, .T. ) ;
#8016=DIRECTION ( 'NONE',  ( 0.000000000000000000, -0.000000000000000000, -1.000000000000000000 ) ) ;
#8019=ORIENTED_EDGE ( 'NONE', *, *, #4418, .F. ) ;
#8020=DIRECTION ( 'NONE',  ( -1.000000000000000000, 0.000000000000000000, 0.000000000000000000 ) ) ;
#8025=CIRCLE ( 'NONE', #17969, 12.36707279061065101 ) ;
#8027=ORIENTED_EDGE ( 'NONE', *, *, #17297, .F. ) ;
#8032=CARTESIAN_POINT ( 'NONE',  ( 33.46699938050303302, 38.56284415653841791, 47.04930799450051637 ) ) ;
#8033=AXIS2_PLACEMENT_3D ( 'NONE', #18959, #21911, #11425 ) ;
#8035=CIRCLE ( 'NONE', #2264, 0.1249999999999966416 ) ;
#8040=ORIENTED_EDGE ( 'NONE', *, *, #29353, .T. ) ;
#8041=DIRECTION ( 'NONE',  ( 0.000000000000000000, -0.000000000000000000, -1.000000000000000000 ) ) ;
#8045=DIRECTION ( 'NONE',  ( -1.101824276508909887E-16, 1.000000000000000000, -0.000000000000000000 ) ) ;
#8050=FACE_OUTER_BOUND ( 'NONE', #27214, .T. ) ;
#8052=ADVANCED_FACE ( 'NONE', ( #21562 ), #30746, .T. ) ;
#8060=EDGE_CURVE ( 'NONE', #4648, #31644, #858, .T. ) ;
#8062=EDGE_CURVE ( 'NONE', #28626, #21972, #26986, .T. ) ;
#8063=ORIENTED_EDGE ( 'NONE', *, *, #6595, .T. ) ;
#8064=AXIS2_PLACEMENT_3D ( 'NONE', #28959, #11879, #3838 ) ;
#8065=AXIS2_PLACEMENT_3D ( 'NONE', #25555, #9816, #25073 ) ;
#8069=CARTESIAN_POINT ( 'NONE',  ( 21.09992658989239089, 26.46664230456639899, 47.04930799450051637 ) ) ;
#8071=AXIS2_PLACEMENT_3D ( 'NONE', #25652, #13199, #3323 ) ;
#8073=DIRECTION ( 'NONE',  ( -1.101824276508909887E-16, 1.000000000000000000, -0.000000000000000000 ) ) ;
#8074=CARTESIAN_POINT ( 'NONE',  ( 8.474859994195286461, 27.34184655352419568, 47.04930799450051637 ) ) ;
#8078=FACE_OUTER_BOUND ( 'NONE', #31960, .T. ) ;
#8084=DIRECTION ( 'NONE',  ( -1.101824276508909887E-16, 1.000000000000000000, -0.000000000000000000 ) ) ;
#8088=FACE_OUTER_BOUND ( 'NONE', #23912, .T. ) ;
#8089=ADVANCED_FACE ( 'NONE', ( #4172 ), #28803, .T. ) ;
#8090=CARTESIAN_POINT ( 'NONE',  ( 21.09992658989238734, 31.71664230456639544, 47.04930799450051637 ) ) ;
#8091=ORIENTED_EDGE ( 'NONE', *, *, #26981, .F. ) ;
#8092=FACE_OUTER_BOUND ( 'NONE', #6759, .T. ) ;
#8095=VERTEX_POINT ( 'NONE', #6966 ) ;
#8099=EDGE_CURVE ( 'NONE', #5841, #28361, #11328, .T. ) ;
#8103=VERTEX_POINT ( 'NONE', #21392 ) ;
#8110=ORIENTED_EDGE ( 'NONE', *, *, #1214, .F. ) ;
#8114=VECTOR ( 'NONE', #18217, 1000.000000000000000 ) ;
#8124=CIRCLE ( 'NONE', #8659, 12.27641737965282687 ) ;
#8130=ORIENTED_EDGE ( 'NONE', *, *, #11685, .T. ) ;
#8135=DIRECTION ( 'NONE',  ( -1.000000000000000000, 0.000000000000000000, 0.000000000000000000 ) ) ;
#8144=AXIS2_PLACEMENT_3D ( 'NONE', #31126, #31281, #25867 ) ;
#8148=CARTESIAN_POINT ( 'NONE',  ( 8.474859994195286461, 27.84184655352419568, 47.04930799450051637 ) ) ;
#8152=DIRECTION ( 'NONE',  ( -1.000000000000000000, 0.000000000000000000, 0.000000000000000000 ) ) ;
#8164=DIRECTION ( 'NONE',  ( -1.000000000000000000, 0.000000000000000000, 0.000000000000000000 ) ) ;
#8167=DIRECTION ( 'NONE',  ( -1.101824276508909887E-16, 1.000000000000000000, -0.000000000000000000 ) ) ;
#8172=AXIS2_PLACEMENT_3D ( 'NONE', #6286, #1354, #5977 ) ;
#8173=CIRCLE ( 'NONE', #22776, 0.1250000000000001110 ) ;
#8175=EDGE_CURVE ( 'NONE', #29193, #29823, #2436, .T. ) ;
#8177=ORIENTED_EDGE ( 'NONE', *, *, #13597, .T. ) ;
#8178=EDGE_CURVE ( 'NONE', #24565, #12553, #21811, .T. ) ;
#8179=ORIENTED_EDGE ( 'NONE', *, *, #2718, .F. ) ;
#8181=ADVANCED_FACE ( 'NONE', ( #7779 ), #4505, .T. ) ;
#8182=AXIS2_PLACEMENT_3D ( 'NONE', #1949, #14280, #11968 ) ;
#8187=AXIS2_PLACEMENT_3D ( 'NONE', #18230, #26109, #20705 ) ;
#8191=DIRECTION ( 'NONE',  ( -1.101824276508909887E-16, 1.000000000000000000, -0.000000000000000000 ) ) ;
#8198=EDGE_LOOP ( 'NONE', ( #30412, #20913, #9673, #26979 ) ) ;
#8199=AXIS2_PLACEMENT_3D ( 'NONE', #9267, #28967, #16633 ) ;
#8200=CARTESIAN_POINT ( 'NONE',  ( 33.50134396954523908, 27.84164230456639544, 47.04930799450051637 ) ) ;
#8205=VERTEX_POINT ( 'NONE', #9595 ) ;
#8207=DIRECTION ( 'NONE',  ( 1.000000000000000000, 0.000000000000000000, 0.000000000000000000 ) ) ;
#8211=LINE ( 'NONE', #22966, #30901 ) ;
#8212=DIRECTION ( 'NONE',  ( 0.000000000000000000, -0.000000000000000000, -1.000000000000000000 ) ) ;
#8225=ORIENTED_EDGE ( 'NONE', *, *, #7820, .F. ) ;
#8229=EDGE_CURVE ( 'NONE', #12341, #15078, #12915, .T. ) ;
#8230=CIRCLE ( 'NONE', #3508, 12.36707279061065101 ) ;
#8235=DIRECTION ( 'NONE',  ( -1.000000000000000000, -1.101824276508909887E-16, 0.000000000000000000 ) ) ;
#8237=CARTESIAN_POINT ( 'NONE',  ( 8.732853799281732776, 32.47145308207317527, 47.04930799450051637 ) ) ;
#8241=ORIENTED_EDGE ( 'NONE', *, *, #13066, .T. ) ;
#8243=CARTESIAN_POINT ( 'NONE',  ( 21.09992658989238734, 38.56284415653841791, 47.04930799450051637 ) ) ;
#8244=CIRCLE ( 'NONE', #30782, 12.62506659569710266 ) ;
#8245=DIRECTION ( 'NONE',  ( -1.000000000000000000, -1.101824276508910010E-16, 0.000000000000000000 ) ) ;
#8246=ORIENTED_EDGE ( 'NONE', *, *, #5594, .T. ) ;
#8250=FACE_OUTER_BOUND ( 'NONE', #21328, .T. ) ;
#8257=CIRCLE ( 'NONE', #28705, 0.1250000000000001110 ) ;
#8266=ADVANCED_FACE ( 'NONE', ( #12390 ), #15010, .T. ) ;
#8269=EDGE_CURVE ( 'NONE', #16793, #3554, #23393, .T. ) ;
#8271=CARTESIAN_POINT ( 'NONE',  ( 8.732853799281738105, 28.21183152705961206, 47.04930799450051637 ) ) ;
#8272=DIRECTION ( 'NONE',  ( 0.000000000000000000, -0.000000000000000000, -1.000000000000000000 ) ) ;
#8273=LINE ( 'NONE', #28297, #29416 ) ;
#8274=ORIENTED_EDGE ( 'NONE', *, *, #21152, .T. ) ;
#8282=AXIS2_PLACEMENT_3D ( 'NONE', #31660, #9167, #9986 ) ;
#8283=EDGE_LOOP ( 'NONE', ( #19216, #3017, #23475, #14545 ) ) ;
#8292=EDGE_LOOP ( 'NONE', ( #18475, #25919, #28695, #14084 ) ) ;
#8294=TOROIDAL_SURFACE ( 'NONE', #8820, 12.40141737965287838, 0.1249999999999998335 ) ;
#8296=AXIS2_PLACEMENT_3D ( 'NONE', #18745, #23692, #1360 ) ;
#8303=DIRECTION ( 'NONE',  ( 0.000000000000000000, -0.000000000000000000, -1.000000000000000000 ) ) ;
#8306=LINE ( 'NONE', #25861, #9940 ) ;
#8313=DIRECTION ( 'NONE',  ( -1.224646799147353207E-16, -1.349345573449484691E-32, 1.000000000000000000 ) ) ;
#8321=ORIENTED_EDGE ( 'NONE', *, *, #5169, .T. ) ;
#8325=CARTESIAN_POINT ( 'NONE',  ( 33.71785032049130137, 31.71664230456639544, 47.04930799450051637 ) ) ;
#8326=CIRCLE ( 'NONE', #14599, 12.36707279061065279 ) ;
#8340=ADVANCED_FACE ( 'NONE', ( #25656 ), #3160, .T. ) ;
#8344=DIRECTION ( 'NONE',  ( -1.000000000000000000, 0.000000000000000000, 0.000000000000000000 ) ) ;
#8353=CARTESIAN_POINT ( 'NONE',  ( 8.474859994195286461, 28.59184655352419213, 47.04930799450051637 ) ) ;
#8355=CARTESIAN_POINT ( 'NONE',  ( 21.09992658989238734, 32.22145308207317527, 47.04930799450051637 ) ) ;
#8357=DIRECTION ( 'NONE',  ( -1.000000000000000000, 0.000000000000000000, 0.000000000000000000 ) ) ;
#8360=CARTESIAN_POINT ( 'NONE',  ( 21.09992658989238734, 31.34143805560860585, 47.04930799450051637 ) ) ;
#8368=CIRCLE ( 'NONE', #26695, 0.1250000000000001110 ) ;
#8369=VERTEX_POINT ( 'NONE', #5966 ) ;
#8384=DIRECTION ( 'NONE',  ( -1.101824276508909887E-16, 1.000000000000000000, -0.000000000000000000 ) ) ;
#8388=TOROIDAL_SURFACE ( 'NONE', #4700, 12.40141737965288726, 0.1250000000000003331 ) ;
#8399=CARTESIAN_POINT ( 'NONE',  ( 33.72499318558949000, 38.56284415653841791, 47.04930799450051637 ) ) ;
#8401=CIRCLE ( 'NONE', #12055, 12.36707279061065101 ) ;
#8402=CARTESIAN_POINT ( 'NONE',  ( 21.09992658989239089, 29.09164230456639899, 47.04930799450051637 ) ) ;
#8404=CARTESIAN_POINT ( 'NONE',  ( 21.09992658989238734, 31.34164230456639544, 47.04930799450051637 ) ) ;
#8428=CIRCLE ( 'NONE', #15679, 12.36707279061065101 ) ;
#8430=AXIS2_PLACEMENT_3D ( 'NONE', #11906, #24049, #21905 ) ;
#8432=DIRECTION ( 'NONE',  ( -1.000000000000000000, -1.101824276508910010E-16, 0.000000000000000000 ) ) ;
#8441=DIRECTION ( 'NONE',  ( -1.000000000000000000, 0.000000000000000000, 0.000000000000000000 ) ) ;
#8446=FACE_OUTER_BOUND ( 'NONE', #29279, .T. ) ;
#8449=DIRECTION ( 'NONE',  ( 1.000000000000000000, 0.000000000000000000, 0.000000000000000000 ) ) ;
#8450=FACE_OUTER_BOUND ( 'NONE', #29835, .T. ) ;
#8456=ORIENTED_EDGE ( 'NONE', *, *, #27085, .F. ) ;
#8457=( GEOMETRIC_REPRESENTATION_CONTEXT ( 3 ) GLOBAL_UNCERTAINTY_ASSIGNED_CONTEXT ( ( #9465 ) ) GLOBAL_UNIT_ASSIGNED_CONTEXT ( ( #11738, #29629, #2536 ) ) REPRESENTATION_CONTEXT ( 'NONE', 'WORKASPACE' ) );
#8460=VERTEX_POINT ( 'NONE', #23990 ) ;
#8468=ORIENTED_EDGE ( 'NONE', *, *, #25650, .F. ) ;
#8469=CIRCLE ( 'NONE', #16838, 0.1250000000000001110 ) ;
#8476=ORIENTED_EDGE ( 'NONE', *, *, #26462, .T. ) ;
#8478=DIRECTION ( 'NONE',  ( -1.101824276508909887E-16, 1.000000000000000000, -0.000000000000000000 ) ) ;
#8482=DIRECTION ( 'NONE',  ( -1.000000000000000000, 0.000000000000000000, 0.000000000000000000 ) ) ;
#8484=CARTESIAN_POINT ( 'NONE',  ( 33.37634396954523197, 28.34164230456639544, 47.04930799450051637 ) ) ;
#8485=FACE_OUTER_BOUND ( 'NONE', #11900, .T. ) ;
#8486=DIRECTION ( 'NONE',  ( -1.101824276508909887E-16, 1.000000000000000000, -0.000000000000000000 ) ) ;
#8492=DIRECTION ( 'NONE',  ( -1.000000000000000000, 0.000000000000000000, 0.000000000000000000 ) ) ;
#8499=ADVANCED_FACE ( 'NONE', ( #1503 ), #10726, .T. ) ;
#8503=ORIENTED_EDGE ( 'NONE', *, *, #15415, .F. ) ;
#8504=CARTESIAN_POINT ( 'NONE',  ( 21.09992658989239089, 28.59143805560861296, 47.04930799450051637 ) ) ;
#8509=CARTESIAN_POINT ( 'NONE',  ( 21.09992658989239089, 28.96664230456639899, 47.04930799450051637 ) ) ;
#8510=FACE_OUTER_BOUND ( 'NONE', #22203, .T. ) ;
#8522=VERTEX_POINT ( 'NONE', #31715 ) ;
#8534=EDGE_CURVE ( 'NONE', #11505, #14982, #31165, .T. ) ;
#8539=AXIS2_PLACEMENT_3D ( 'NONE', #6404, #16406, #29212 ) ;
#8540=AXIS2_PLACEMENT_3D ( 'NONE', #28190, #18489, #6344 ) ;
#8541=ORIENTED_EDGE ( 'NONE', *, *, #11781, .F. ) ;
#8544=DIRECTION ( 'NONE',  ( -1.000000000000000000, 0.000000000000000000, 0.000000000000000000 ) ) ;
#8548=CARTESIAN_POINT ( 'NONE',  ( 33.46699938050304013, 27.22145308207318593, 47.04930799450050927 ) ) ;
#8549=ORIENTED_EDGE ( 'NONE', *, *, #31907, .T. ) ;
#8551=ORIENTED_EDGE ( 'NONE', *, *, #23594, .T. ) ;
#8556=DIRECTION ( 'NONE',  ( -1.101824276508909887E-16, 1.000000000000000000, -0.000000000000000000 ) ) ;
#8560=EDGE_CURVE ( 'NONE', #12904, #10473, #21182, .T. ) ;
#8564=ORIENTED_EDGE ( 'NONE', *, *, #17938, .F. ) ;
#8566=CARTESIAN_POINT ( 'NONE',  ( 33.46699938050304013, 26.47145308207318593, 47.04930799450050927 ) ) ;
#8567=CIRCLE ( 'NONE', #15388, 12.62506659569710266 ) ;
#8574=EDGE_CURVE ( 'NONE', #16617, #22868, #6442, .T. ) ;
#8575=ORIENTED_EDGE ( 'NONE', *, *, #4213, .T. ) ;
#8577=DIRECTION ( 'NONE',  ( -1.101824276508909887E-16, 1.000000000000000000, -0.000000000000000000 ) ) ;
#8578=CARTESIAN_POINT ( 'NONE',  ( 21.09992658989239089, 30.34143805560860585, 47.04930799450051637 ) ) ;
#8581=CIRCLE ( 'NONE', #12251, 12.36707279061065101 ) ;
#8582=AXIS2_PLACEMENT_3D ( 'NONE', #12713, #24679, #17450 ) ;
#8585=CARTESIAN_POINT ( 'NONE',  ( 21.09992658989239089, 23.84164230456639544, 47.04930799450051637 ) ) ;
#8587=ORIENTED_EDGE ( 'NONE', *, *, #30401, .F. ) ;
#8588=CARTESIAN_POINT ( 'NONE',  ( 21.09992658989239089, 29.09164230456639899, 47.04930799450051637 ) ) ;
#8595=CARTESIAN_POINT ( 'NONE',  ( 21.09992658989239089, 24.71183152705960140, 47.04930799450051637 ) ) ;
#8596=DIRECTION ( 'NONE',  ( -1.101824276508909887E-16, 1.000000000000000000, -0.000000000000000000 ) ) ;
#8598=CARTESIAN_POINT ( 'NONE',  ( 8.732853799281734553, 29.72145308207318237, 47.04930799450051637 ) ) ;
#8599=LINE ( 'NONE', #16132, #10365 ) ;
#8601=CIRCLE ( 'NONE', #28078, 12.27641737965282687 ) ;
#8602=VERTEX_POINT ( 'NONE', #7741 ) ;
#8610=DIRECTION ( 'NONE',  ( -1.101824276508909887E-16, 1.000000000000000000, -0.000000000000000000 ) ) ;
#8616=AXIS2_PLACEMENT_3D ( 'NONE', #13997, #18898, #16445 ) ;
#8618=EDGE_CURVE ( 'NONE', #8369, #31649, #9134, .T. ) ;
#8624=AXIS2_PLACEMENT_3D ( 'NONE', #28075, #658, #2950 ) ;
#8625=ADVANCED_FACE ( 'NONE', ( #22497 ), #17251, .F. ) ;
#8628=ORIENTED_EDGE ( 'NONE', *, *, #11440, .F. ) ;
#8630=DIRECTION ( 'NONE',  ( -1.101824276508909887E-16, 1.000000000000000000, -0.000000000000000000 ) ) ;
#8631=FACE_OUTER_BOUND ( 'NONE', #20778, .T. ) ;
#8634=ADVANCED_FACE ( 'NONE', ( #10049 ), #7572, .T. ) ;
#8642=DIRECTION ( 'NONE',  ( -1.000000000000000000, 0.000000000000000000, 0.000000000000000000 ) ) ;
#8644=DIRECTION ( 'NONE',  ( -1.101824276508909887E-16, 1.000000000000000000, -0.000000000000000000 ) ) ;
#8651=CARTESIAN_POINT ( 'NONE',  ( 33.72499318558949710, 30.09184655352422411, 47.04930799450051637 ) ) ;
#8654=AXIS2_PLACEMENT_3D ( 'NONE', #23952, #3612, #21483 ) ;
#8656=ADVANCED_FACE ( 'NONE', ( #32367 ), #27439, .F. ) ;
#8657=AXIS2_PLACEMENT_3D ( 'NONE', #26873, #29172, #22099 ) ;
#8659=AXIS2_PLACEMENT_3D ( 'NONE', #21963, #24112, #9512 ) ;
#8662=EDGE_CURVE ( 'NONE', #21925, #3138, #15465, .T. ) ;
#8663=FACE_OUTER_BOUND ( 'NONE', #8292, .T. ) ;
#8669=DIRECTION ( 'NONE',  ( -1.000000000000000000, -1.101824276508909764E-16, 0.000000000000000000 ) ) ;
#8671=AXIS2_PLACEMENT_3D ( 'NONE', #17881, #12967, #10675 ) ;
#8678=CARTESIAN_POINT ( 'NONE',  ( 8.732853799281738105, 23.71183152705959429, 47.04930799450051637 ) ) ;
#8680=CIRCLE ( 'NONE', #27018, 0.1249999999999983763 ) ;
#8682=DIRECTION ( 'NONE',  ( -1.101824276508909887E-16, 1.000000000000000000, -0.000000000000000000 ) ) ;
#8686=DIRECTION ( 'NONE',  ( -1.101824276508909887E-16, 1.000000000000000000, -0.000000000000000000 ) ) ;
#8688=DIRECTION ( 'NONE',  ( -1.000000000000000000, 0.000000000000000000, 0.000000000000000000 ) ) ;
#8689=AXIS2_PLACEMENT_3D ( 'NONE', #4573, #9345, #19342 ) ;
#8692=FACE_OUTER_BOUND ( 'NONE', #5255, .T. ) ;
#8695=DIRECTION ( 'NONE',  ( -1.101824276508909887E-16, 1.000000000000000000, -0.000000000000000000 ) ) ;
#8697=CIRCLE ( 'NONE', #2401, 12.36707279061065101 ) ;
#8701=DIRECTION ( 'NONE',  ( -1.101824276508909887E-16, 1.000000000000000000, -0.000000000000000000 ) ) ;
#8704=CARTESIAN_POINT ( 'NONE',  ( 8.482002859293478636, 32.46664230456639899, 47.04930799450051637 ) ) ;
#8708=DIRECTION ( 'NONE',  ( -1.000000000000000000, 0.000000000000000000, 0.000000000000000000 ) ) ;
#8709=EDGE_CURVE ( 'NONE', #32275, #7848, #19091, .T. ) ;
#8713=CARTESIAN_POINT ( 'NONE',  ( 21.09992658989238734, 38.56284415653841791, 47.04930799450051637 ) ) ;
#8715=ORIENTED_EDGE ( 'NONE', *, *, #12798, .F. ) ;
#8722=CARTESIAN_POINT ( 'NONE',  ( 21.09992658989239089, 30.59164230456639544, 47.04930799450051637 ) ) ;
#8727=TOROIDAL_SURFACE ( 'NONE', #10848, 12.40141737965279667, 0.1249999999999991951 ) ;
#8729=ORIENTED_EDGE ( 'NONE', *, *, #16184, .T. ) ;
#8730=FACE_OUTER_BOUND ( 'NONE', #13903, .T. ) ;
#8731=AXIS2_PLACEMENT_3D ( 'NONE', #21458, #23769, #4400 ) ;
#8737=AXIS2_PLACEMENT_3D ( 'NONE', #7941, #30260, #7773 ) ;
#8739=DIRECTION ( 'NONE',  ( -1.101824276508909887E-16, 1.000000000000000000, -0.000000000000000000 ) ) ;
#8740=EDGE_CURVE ( 'NONE', #7606, #8522, #9675, .T. ) ;
#8746=EDGE_CURVE ( 'NONE', #13651, #11753, #10704, .T. ) ;
#8748=DIRECTION ( 'NONE',  ( -1.000000000000000000, 0.000000000000000000, 0.000000000000000000 ) ) ;
#8755=ORIENTED_EDGE ( 'NONE', *, *, #25817, .T. ) ;
#8756=DIRECTION ( 'NONE',  ( -1.101824276508909887E-16, 1.000000000000000000, -0.000000000000000000 ) ) ;
#8757=DIRECTION ( 'NONE',  ( -1.000000000000000000, 0.000000000000000000, 0.000000000000000000 ) ) ;
#8769=DIRECTION ( 'NONE',  ( -1.000000000000000000, 0.000000000000000000, 0.000000000000000000 ) ) ;
#8778=CIRCLE ( 'NONE', #20311, 12.62506659569710266 ) ;
#8783=DIRECTION ( 'NONE',  ( -1.101824276508909887E-16, 1.000000000000000000, -0.000000000000000000 ) ) ;
#8784=CARTESIAN_POINT ( 'NONE',  ( 33.46699938050303302, 38.56284415653841791, 47.04930799450051637 ) ) ;
#8785=CYLINDRICAL_SURFACE ( 'NONE', #31550, 12.62506659569710266 ) ;
#8787=DIRECTION ( 'NONE',  ( 1.000000000000000000, 0.000000000000000000, 0.000000000000000000 ) ) ;
#8788=DIRECTION ( 'NONE',  ( 1.000000000000000000, 0.000000000000000000, 0.000000000000000000 ) ) ;
#8790=CARTESIAN_POINT ( 'NONE',  ( 33.71785032049139375, 23.71664230456639899, 47.04930799450051637 ) ) ;
#8797=CYLINDRICAL_SURFACE ( 'NONE', #8540, 12.62506659569710443 ) ;
#8798=ORIENTED_EDGE ( 'NONE', *, *, #15128, .T. ) ;
#8801=CIRCLE ( 'NONE', #24002, 0.1250000000000001110 ) ;
#8802=VECTOR ( 'NONE', #28844, 1000.000000000000000 ) ;
#8804=EDGE_LOOP ( 'NONE', ( #28884, #13302, #11609, #798 ) ) ;
#8805=VECTOR ( 'NONE', #16456, 1000.000000000000000 ) ;
#8806=VECTOR ( 'NONE', #17436, 1000.000000000000000 ) ;
#8811=ORIENTED_EDGE ( 'NONE', *, *, #30815, .F. ) ;
#8820=AXIS2_PLACEMENT_3D ( 'NONE', #10402, #7945, #16275 ) ;
#8821=EDGE_LOOP ( 'NONE', ( #1523, #11736, #5553, #31302 ) ) ;
#8823=CIRCLE ( 'NONE', #4119, 12.27641737965285706 ) ;
#8826=AXIS2_PLACEMENT_3D ( 'NONE', #31821, #27665, #7655 ) ;
#8832=TOROIDAL_SURFACE ( 'NONE', #16157, 12.40141737965284108, 0.1249999999999997918 ) ;
#8835=EDGE_LOOP ( 'NONE', ( #246, #30647, #29242, #30986 ) ) ;
#8837=CARTESIAN_POINT ( 'NONE',  ( 33.60959714501833417, 23.65414230456639544, 47.04930799450051637 ) ) ;
#8839=AXIS2_PLACEMENT_3D ( 'NONE', #22847, #25794, #5783 ) ;
#8840=FACE_OUTER_BOUND ( 'NONE', #464, .T. ) ;
#8841=CARTESIAN_POINT ( 'NONE',  ( 21.09992658989239089, 29.34143805560861296, 47.04930799450051637 ) ) ;
#8842=EDGE_LOOP ( 'NONE', ( #5592, #17706, #4279, #8091 ) ) ;
#8843=DIRECTION ( 'NONE',  ( -1.101824276508909887E-16, 1.000000000000000000, -0.000000000000000000 ) ) ;
#8846=DIRECTION ( 'NONE',  ( 0.000000000000000000, -0.000000000000000000, -1.000000000000000000 ) ) ;
#8847=DIRECTION ( 'NONE',  ( -1.101824276508909887E-16, 1.000000000000000000, -0.000000000000000000 ) ) ;
#8849=ORIENTED_EDGE ( 'NONE', *, *, #24563, .F. ) ;
#8851=EDGE_CURVE ( 'NONE', #460, #4474, #10534, .T. ) ;
#8853=EDGE_CURVE ( 'NONE', #11099, #11910, #5600, .T. ) ;
#8854=AXIS2_PLACEMENT_3D ( 'NONE', #10681, #3430, #26070 ) ;
#8857=FACE_OUTER_BOUND ( 'NONE', #3996, .T. ) ;
#8859=AXIS2_PLACEMENT_3D ( 'NONE', #9173, #4074, #18679 ) ;
#8861=DIRECTION ( 'NONE',  ( -1.000000000000000000, 0.000000000000000000, 0.000000000000000000 ) ) ;
#8865=CARTESIAN_POINT ( 'NONE',  ( 21.09992658989239089, 29.21183152705961206, 47.04930799450051637 ) ) ;
#8866=ORIENTED_EDGE ( 'NONE', *, *, #16245, .F. ) ;
#8871=ORIENTED_EDGE ( 'NONE', *, *, #18612, .T. ) ;
#8872=ORIENTED_EDGE ( 'NONE', *, *, #10655, .T. ) ;
#8873=DIRECTION ( 'NONE',  ( -1.101824276508909887E-16, 1.000000000000000000, -0.000000000000000000 ) ) ;
#8874=AXIS2_PLACEMENT_3D ( 'NONE', #18623, #26177, #20929 ) ;
#8880=DIRECTION ( 'NONE',  ( -1.101824276508909887E-16, 1.000000000000000000, -0.000000000000000000 ) ) ;
#8882=ORIENTED_EDGE ( 'NONE', *, *, #3589, .F. ) ;
#8887=CARTESIAN_POINT ( 'NONE',  ( 8.474859994195286461, 29.09143805560861296, 47.04930799450051637 ) ) ;
#8890=EDGE_CURVE ( 'NONE', #4682, #10687, #12301, .T. ) ;
#8893=CARTESIAN_POINT ( 'NONE',  ( 33.72499318558949710, 23.84143805560861296, 47.04930799450050927 ) ) ;
#8894=DIRECTION ( 'NONE',  ( -1.000000000000000000, -1.101824276508910010E-16, 0.000000000000000000 ) ) ;
#8897=CIRCLE ( 'NONE', #30957, 0.1250000000000001110 ) ;
#8903=CARTESIAN_POINT ( 'NONE',  ( 21.09992658989239089, 28.59164230456639544, 47.04930799450051637 ) ) ;
#8913=CARTESIAN_POINT ( 'NONE',  ( 8.698509210239558698, 29.09164230456639899, 47.04930799450051637 ) ) ;
#8929=ORIENTED_EDGE ( 'NONE', *, *, #16516, .T. ) ;
#8932=TOROIDAL_SURFACE ( 'NONE', #20996, 12.61792373059895311, 0.1249999999999983485 ) ;
#8933=ADVANCED_FACE ( 'NONE', ( #6084 ), #1297, .T. ) ;
#8937=AXIS2_PLACEMENT_3D ( 'NONE', #30975, #18004, #30809 ) ;
#8939=CARTESIAN_POINT ( 'NONE',  ( 21.09992658989239089, 25.09164230456639899, 47.04930799450051637 ) ) ;
#8940=DIRECTION ( 'NONE',  ( -1.224646799147353207E-16, -1.349345573449484691E-32, 1.000000000000000000 ) ) ;
#8941=TOROIDAL_SURFACE ( 'NONE', #10531, 12.40141737965285174, 0.1249999999999993200 ) ;
#8942=ORIENTED_EDGE ( 'NONE', *, *, #15824, .T. ) ;
#8943=DIRECTION ( 'NONE',  ( 0.000000000000000000, -0.000000000000000000, -1.000000000000000000 ) ) ;
#8944=ORIENTED_EDGE ( 'NONE', *, *, #22002, .F. ) ;
#8945=DIRECTION ( 'NONE',  ( -1.224646799147353207E-16, -1.349345573449484691E-32, 1.000000000000000000 ) ) ;
#8949=DIRECTION ( 'NONE',  ( -1.101824276508909887E-16, 1.000000000000000000, -0.000000000000000000 ) ) ;
#8950=DIRECTION ( 'NONE',  ( -1.000000000000000000, 0.000000000000000000, 0.000000000000000000 ) ) ;
#8955=DIRECTION ( 'NONE',  ( -1.000000000000000000, 0.000000000000000000, 0.000000000000000000 ) ) ;
#8965=VECTOR ( 'NONE', #26664, 1000.000000000000000 ) ;
#8969=DIRECTION ( 'NONE',  ( -1.101824276508909887E-16, 1.000000000000000000, -0.000000000000000000 ) ) ;
#8973=ORIENTED_EDGE ( 'NONE', *, *, #30886, .T. ) ;
#8974=EDGE_CURVE ( 'NONE', #11669, #14845, #24886, .T. ) ;
#8980=EDGE_LOOP ( 'NONE', ( #4662, #24894, #1785, #31811 ) ) ;
#8982=CYLINDRICAL_SURFACE ( 'NONE', #31912, 12.62506659569710266 ) ;
#8990=ORIENTED_EDGE ( 'NONE', *, *, #20565, .F. ) ;
#8991=CARTESIAN_POINT ( 'NONE',  ( 33.72499318558949710, 29.59143805560861296, 47.04930799450051637 ) ) ;
#8996=CARTESIAN_POINT ( 'NONE',  ( 8.474859994195286461, 28.34184655352419213, 47.04930799450051637 ) ) ;
#8999=DIRECTION ( 'NONE',  ( -1.101824276508909887E-16, 1.000000000000000000, -0.000000000000000000 ) ) ;
#9002=DIRECTION ( 'NONE',  ( -1.000000000000000000, -1.101824276508909887E-16, 0.000000000000000000 ) ) ;
#9007=CARTESIAN_POINT ( 'NONE',  ( 33.46699938050304013, 24.22145308207319303, 47.04930799450050927 ) ) ;
#9008=DIRECTION ( 'NONE',  ( -1.000000000000000000, 0.000000000000000000, 0.000000000000000000 ) ) ;
#9009=VERTEX_POINT ( 'NONE', #24772 ) ;
#9016=ADVANCED_FACE ( 'NONE', ( #20003 ), #11789, .T. ) ;
#9022=CIRCLE ( 'NONE', #31572, 0.1250000000000001110 ) ;
#9029=ORIENTED_EDGE ( 'NONE', *, *, #9535, .T. ) ;
#9034=FACE_OUTER_BOUND ( 'NONE', #14746, .T. ) ;
#9042=DIRECTION ( 'NONE',  ( -1.000000000000000000, 0.000000000000000000, 0.000000000000000000 ) ) ;
#9043=AXIS2_PLACEMENT_3D ( 'NONE', #30043, #17389, #27236 ) ;
#9045=DIRECTION ( 'NONE',  ( -1.000000000000000000, 0.000000000000000000, 0.000000000000000000 ) ) ;
#9052=DIRECTION ( 'NONE',  ( -1.000000000000000000, 0.000000000000000000, 0.000000000000000000 ) ) ;
#9059=ORIENTED_EDGE ( 'NONE', *, *, #20670, .F. ) ;
#9060=TOROIDAL_SURFACE ( 'NONE', #3810, 12.40141737965283575, 0.1250000000000000278 ) ;
#9064=EDGE_CURVE ( 'NONE', #27697, #16912, #10250, .T. ) ;
#9073=CARTESIAN_POINT ( 'NONE',  ( 33.46699938050304013, 28.96183152705961206, 47.04930799450051637 ) ) ;
#9079=CARTESIAN_POINT ( 'NONE',  ( 21.09992658989238734, 32.46664230456639899, 47.04930799450051637 ) ) ;
#9081=VERTEX_POINT ( 'NONE', #11978 ) ;
#9092=DIRECTION ( 'NONE',  ( -1.101824276508909887E-16, 1.000000000000000000, -0.000000000000000000 ) ) ;
#9096=ORIENTED_EDGE ( 'NONE', *, *, #20338, .T. ) ;
#9099=AXIS2_PLACEMENT_3D ( 'NONE', #4820, #20075, #7616 ) ;
#9101=DIRECTION ( 'NONE',  ( -1.101824276508909887E-16, 1.000000000000000000, -0.000000000000000000 ) ) ;
#9108=DIRECTION ( 'NONE',  ( -1.101824276508909887E-16, 1.000000000000000000, -0.000000000000000000 ) ) ;
#9112=FACE_OUTER_BOUND ( 'NONE', #9734, .T. ) ;
#9114=ORIENTED_EDGE ( 'NONE', *, *, #25213, .F. ) ;
#9116=EDGE_CURVE ( 'NONE', #28525, #23085, #3410, .T. ) ;
#9123=ADVANCED_FACE ( 'NONE', ( #150 ), #16893, .T. ) ;
#9125=DIRECTION ( 'NONE',  ( -1.101824276508909887E-16, 1.000000000000000000, -0.000000000000000000 ) ) ;
#9126=CARTESIAN_POINT ( 'NONE',  ( 21.09992658989238734, 32.09164230456639899, 47.04930799450051637 ) ) ;
#9128=CARTESIAN_POINT ( 'NONE',  ( 21.09992658989239089, 27.21664230456639899, 47.04930799450051637 ) ) ;
#9129=CARTESIAN_POINT ( 'NONE',  ( 21.09992658989239089, 27.34164230456639544, 47.04930799450051637 ) ) ;
#9130=ORIENTED_EDGE ( 'NONE', *, *, #10502, .F. ) ;
#9134=CIRCLE ( 'NONE', #27486, 12.62506659569710266 ) ;
#9140=ORIENTED_EDGE ( 'NONE', *, *, #25255, .T. ) ;
#9141=CARTESIAN_POINT ( 'NONE',  ( 21.09992658989238734, 32.46183152705962272, 47.04930799450051637 ) ) ;
#9157=EDGE_CURVE ( 'NONE', #12851, #26804, #15997, .T. ) ;
#9163=TOROIDAL_SURFACE ( 'NONE', #30679, 12.61792373059895844, 0.1249999999999980571 ) ;
#9167=DIRECTION ( 'NONE',  ( -1.101824276508909887E-16, 1.000000000000000000, -0.000000000000000000 ) ) ;
#9173=CARTESIAN_POINT ( 'NONE',  ( 21.09992658989239089, 25.59164230456639899, 47.04930799450051637 ) ) ;
#9174=ORIENTED_EDGE ( 'NONE', *, *, #31123, .T. ) ;
#9176=ORIENTED_EDGE ( 'NONE', *, *, #17454, .F. ) ;
#9177=CYLINDRICAL_SURFACE ( 'NONE', #21454, 12.36707279061065101 ) ;
#9180=EDGE_LOOP ( 'NONE', ( #444, #31837, #11917, #28031 ) ) ;
#9183=EDGE_CURVE ( 'NONE', #25724, #5204, #28045, .T. ) ;
#9185=CIRCLE ( 'NONE', #8144, 12.62506659569710266 ) ;
#9186=DIRECTION ( 'NONE',  ( -1.101824276508909887E-16, 1.000000000000000000, -0.000000000000000000 ) ) ;
#9194=ORIENTED_EDGE ( 'NONE', *, *, #17037, .T. ) ;
#9198=CARTESIAN_POINT ( 'NONE',  ( 33.46699938050304013, 30.21183152705961561, 47.04930799450051637 ) ) ;
#9199=LINE ( 'NONE', #24291, #39 ) ;
#9204=DIRECTION ( 'NONE',  ( -1.101824276508909887E-16, 1.000000000000000000, -0.000000000000000000 ) ) ;
#9211=ORIENTED_EDGE ( 'NONE', *, *, #9674, .F. ) ;
#9212=LINE ( 'NONE', #32193, #7785 ) ;
#9213=AXIS2_PLACEMENT_3D ( 'NONE', #27940, #22842, #22191 ) ;
#9215=CIRCLE ( 'NONE', #29127, 0.1250000000000001110 ) ;
#9216=EDGE_CURVE ( 'NONE', #13562, #19299, #24915, .T. ) ;
#9218=VECTOR ( 'NONE', #21647, 1000.000000000000000 ) ;
#9223=CARTESIAN_POINT ( 'NONE',  ( 33.50134396954526750, 24.84164230456639544, 47.04930799450051637 ) ) ;
#9226=VERTEX_POINT ( 'NONE', #13290 ) ;
#9230=AXIS2_PLACEMENT_3D ( 'NONE', #12160, #32345, #7228 ) ;
#9239=ORIENTED_EDGE ( 'NONE', *, *, #7039, .F. ) ;
#9240=LINE ( 'NONE', #19228, #14984 ) ;
#9244=CARTESIAN_POINT ( 'NONE',  ( 21.09992658989238734, 38.56284415653841791, 47.04930799450051637 ) ) ;
#9250=VERTEX_POINT ( 'NONE', #17697 ) ;
#9253=CARTESIAN_POINT ( 'NONE',  ( 21.09992658989239089, 27.34184655352419568, 47.04930799450051637 ) ) ;
#9257=EDGE_LOOP ( 'NONE', ( #30820, #14550, #412, #20656 ) ) ;
#9261=ORIENTED_EDGE ( 'NONE', *, *, #11523, .T. ) ;
#9264=CIRCLE ( 'NONE', #360, 0.1249999999999931721 ) ;
#9265=ADVANCED_FACE ( 'NONE', ( #5891 ), #5404, .F. ) ;
#9267=CARTESIAN_POINT ( 'NONE',  ( 21.09992658989238734, 38.56284415653841791, 47.04930799450051637 ) ) ;
#9274=CARTESIAN_POINT ( 'NONE',  ( 8.732853799281732776, 24.97145308207319303, 47.04930799450051637 ) ) ;
#9276=DIRECTION ( 'NONE',  ( -1.000000000000000000, 0.000000000000000000, 0.000000000000000000 ) ) ;
#9281=DIRECTION ( 'NONE',  ( -1.000000000000000000, -1.101824276508909887E-16, 0.000000000000000000 ) ) ;
#9283=DIRECTION ( 'NONE',  ( -1.000000000000000000, 0.000000000000000000, 0.000000000000000000 ) ) ;
#9286=CARTESIAN_POINT ( 'NONE',  ( 33.50134396954524618, 26.84164230456639899, 47.04930799450051637 ) ) ;
#9290=DIRECTION ( 'NONE',  ( -1.101824276508909887E-16, 1.000000000000000000, -0.000000000000000000 ) ) ;
#9293=CIRCLE ( 'NONE', #18716, 12.36707279061065101 ) ;
#9295=AXIS2_PLACEMENT_3D ( 'NONE', #6755, #31384, #16590 ) ;
#9296=ADVANCED_FACE ( 'NONE', ( #28047 ), #29094, .T. ) ;
#9298=AXIS2_PLACEMENT_3D ( 'NONE', #18434, #13847, #28466 ) ;
#9308=ORIENTED_EDGE ( 'NONE', *, *, #9535, .F. ) ;
#9311=DIRECTION ( 'NONE',  ( -1.000000000000000000, -1.101824276508909887E-16, 0.000000000000000000 ) ) ;
#9321=ORIENTED_EDGE ( 'NONE', *, *, #26227, .T. ) ;
#9323=FACE_OUTER_BOUND ( 'NONE', #14434, .T. ) ;
#9326=AXIS2_PLACEMENT_3D ( 'NONE', #15203, #32118, #22409 ) ;
#9328=CARTESIAN_POINT ( 'NONE',  ( 8.732853799281732776, 32.46183152705962272, 47.04930799450051637 ) ) ;
#9330=CYLINDRICAL_SURFACE ( 'NONE', #11428, 12.62506659569710443 ) ;
#9331=TOROIDAL_SURFACE ( 'NONE', #10398, 12.61792373059893535, 0.1249999999999994033 ) ;
#9333=CARTESIAN_POINT ( 'NONE',  ( 21.09992658989239089, 30.34184655352422411, 47.04930799450051637 ) ) ;
#9338=ADVANCED_FACE ( 'NONE', ( #23599 ), #11809, .T. ) ;
#9341=EDGE_CURVE ( 'NONE', #12012, #25631, #1844, .T. ) ;
#9344=TOROIDAL_SURFACE ( 'NONE', #18764, 12.40141737965285706, 0.1250000000000007494 ) ;
#9345=DIRECTION ( 'NONE',  ( -1.224646799147353207E-16, -1.349345573449484691E-32, 1.000000000000000000 ) ) ;
#9346=FACE_OUTER_BOUND ( 'NONE', #7738, .T. ) ;
#9349=ORIENTED_EDGE ( 'NONE', *, *, #28269, .F. ) ;
#9354=FACE_OUTER_BOUND ( 'NONE', #31339, .T. ) ;
#9361=DIRECTION ( 'NONE',  ( -1.101824276508909887E-16, 1.000000000000000000, -0.000000000000000000 ) ) ;
#9363=ADVANCED_FACE ( 'NONE', ( #20968 ), #12880, .T. ) ;
#9368=LINE ( 'NONE', #2145, #4147 ) ;
#9369=ORIENTED_EDGE ( 'NONE', *, *, #5434, .F. ) ;
#9373=CARTESIAN_POINT ( 'NONE',  ( 21.09992658989238734, 38.56284415653841791, 47.04930799450051637 ) ) ;
#9377=CIRCLE ( 'NONE', #23005, 12.36707279061065101 ) ;
#9381=CARTESIAN_POINT ( 'NONE',  ( 21.09992658989239089, 23.84143805560861296, 47.04930799450051637 ) ) ;
#9382=ADVANCED_FACE ( 'NONE', ( #16048 ), #30705, .T. ) ;
#9388=CARTESIAN_POINT ( 'NONE',  ( 8.732853799281732776, 38.56284415653841791, 47.04930799450051637 ) ) ;
#9393=DIRECTION ( 'NONE',  ( -1.000000000000000000, 0.000000000000000000, 0.000000000000000000 ) ) ;
#9397=DIRECTION ( 'NONE',  ( -1.224646799147353207E-16, -1.349345573449484691E-32, 1.000000000000000000 ) ) ;
#9405=TOROIDAL_SURFACE ( 'NONE', #11482, 12.40141737965279667, 0.1249999999999991951 ) ;
#9407=EDGE_LOOP ( 'NONE', ( #10607, #10486, #11875, #25472 ) ) ;
#9411=CARTESIAN_POINT ( 'NONE',  ( 21.09992658989238734, 32.34164230456639899, 47.04930799450051637 ) ) ;
#9412=ORIENTED_EDGE ( 'NONE', *, *, #8853, .F. ) ;
#9418=DIRECTION ( 'NONE',  ( -1.224646799147353207E-16, -1.349345573449484691E-32, 1.000000000000000000 ) ) ;
#9419=CARTESIAN_POINT ( 'NONE',  ( 21.09992658989238734, 30.84184655352422411, 47.04930799450051637 ) ) ;
#9420=VERTEX_POINT ( 'NONE', #18976 ) ;
#9422=EDGE_LOOP ( 'NONE', ( #20927, #3158, #141, #30503 ) ) ;
#9423=CIRCLE ( 'NONE', #16229, 0.1250000000000001110 ) ;
#9425=EDGE_LOOP ( 'NONE', ( #3513, #13446, #24116, #17809 ) ) ;
#9427=DIRECTION ( 'NONE',  ( -1.000000000000000000, -1.101824276508909764E-16, 0.000000000000000000 ) ) ;
#9429=AXIS2_PLACEMENT_3D ( 'NONE', #12540, #19907, #12379 ) ;
#9430=EDGE_LOOP ( 'NONE', ( #28123, #20991, #32343, #7297 ) ) ;
#9432=DIRECTION ( 'NONE',  ( -1.101824276508909887E-16, 1.000000000000000000, -0.000000000000000000 ) ) ;
#9441=LINE ( 'NONE', #32258, #11088 ) ;
#9451=CARTESIAN_POINT ( 'NONE',  ( 33.72499318558949710, 28.84184655352418858, 47.04930799450051637 ) ) ;
#9453=DIRECTION ( 'NONE',  ( -1.224646799147353207E-16, -1.349345573449484691E-32, 1.000000000000000000 ) ) ;
#9459=EDGE_CURVE ( 'NONE', #28129, #25242, #19136, .T. ) ;
#9460=ORIENTED_EDGE ( 'NONE', *, *, #10487, .T. ) ;
#9463=CIRCLE ( 'NONE', #18881, 0.1250000000000001110 ) ;
#9465=UNCERTAINTY_MEASURE_WITH_UNIT (LENGTH_MEASURE( 1.000000000000000082E-05 ), #11738, 'distance_accuracy_value', 'NONE');
#9467=CIRCLE ( 'NONE', #15746, 12.27641737965283575 ) ;
#9469=AXIS2_PLACEMENT_3D ( 'NONE', #10140, #23413, #13095 ) ;
#9472=DIRECTION ( 'NONE',  ( -1.101824276508909887E-16, 1.000000000000000000, -0.000000000000000000 ) ) ;
#9479=AXIS2_PLACEMENT_3D ( 'NONE', #29294, #28647, #18780 ) ;
#9481=CARTESIAN_POINT ( 'NONE',  ( 8.823509210239501854, 23.59164230456639544, 47.04930799450051637 ) ) ;
#9484=VECTOR ( 'NONE', #26317, 1000.000000000000000 ) ;
#9487=FACE_OUTER_BOUND ( 'NONE', #6280, .T. ) ;
#9488=DIRECTION ( 'NONE',  ( -1.000000000000000000, 0.000000000000000000, 0.000000000000000000 ) ) ;
#9497=VECTOR ( 'NONE', #29017, 1000.000000000000000 ) ;
#9499=ADVANCED_FACE ( 'NONE', ( #29991 ), #26868, .T. ) ;
#9501=CARTESIAN_POINT ( 'NONE',  ( 33.50134396954525329, 25.84164230456639899, 47.04930799450051637 ) ) ;
#9502=EDGE_LOOP ( 'NONE', ( #14669, #11914, #15074, #8019 ) ) ;
#9503=ORIENTED_EDGE ( 'NONE', *, *, #8662, .T. ) ;
#9505=VERTEX_POINT ( 'NONE', #4381 ) ;
#9507=AXIS2_PLACEMENT_3D ( 'NONE', #13883, #14695, #25021 ) ;
#9508=CIRCLE ( 'NONE', #24715, 12.27641737965281976 ) ;
#9509=AXIS2_PLACEMENT_3D ( 'NONE', #922, #28183, #770 ) ;
#9510=EDGE_LOOP ( 'NONE', ( #2956, #12509, #797, #20751 ) ) ;
#9511=PRODUCT_DEFINITION ( 'UNKNOWN', '', #15008, #31149 ) ;
#9512=DIRECTION ( 'NONE',  ( -1.000000000000000000, 0.000000000000000000, 0.000000000000000000 ) ) ;
#9516=ORIENTED_EDGE ( 'NONE', *, *, #30807, .T. ) ;
#9523=ORIENTED_EDGE ( 'NONE', *, *, #29916, .T. ) ;
#9526=CARTESIAN_POINT ( 'NONE',  ( 21.09992658989239089, 30.09164230456639544, 47.04930799450051637 ) ) ;
#9528=AXIS2_PLACEMENT_3D ( 'NONE', #4034, #9125, #19116 ) ;
#9529=DIRECTION ( 'NONE',  ( -1.101824276508909887E-16, 1.000000000000000000, -0.000000000000000000 ) ) ;
#9531=EDGE_LOOP ( 'NONE', ( #20759, #15621, #8027, #21384 ) ) ;
#9532=ORIENTED_EDGE ( 'NONE', *, *, #335, .T. ) ;
#9535=EDGE_CURVE ( 'NONE', #27500, #5504, #22294, .T. ) ;
#9537=DIRECTION ( 'NONE',  ( -1.000000000000000000, -1.101824276508909887E-16, 0.000000000000000000 ) ) ;
#9538=EDGE_CURVE ( 'NONE', #11991, #24621, #16466, .T. ) ;
#9547=AXIS2_PLACEMENT_3D ( 'NONE', #23922, #26393, #3902 ) ;
#9549=ORIENTED_EDGE ( 'NONE', *, *, #5945, .F. ) ;
#9564=PRODUCT ( 'Coil', 'Coil', '', ( #27574 ) ) ;
#9570=AXIS2_PLACEMENT_3D ( 'NONE', #4232, #16682, #9311 ) ;
#9571=DIRECTION ( 'NONE',  ( -1.000000000000000000, 0.000000000000000000, 0.000000000000000000 ) ) ;
#9577=CARTESIAN_POINT ( 'NONE',  ( 21.09992658989239089, 25.21183152705960140, 47.04930799450051637 ) ) ;
#9581=ORIENTED_EDGE ( 'NONE', *, *, #5152, .T. ) ;
#9589=ORIENTED_EDGE ( 'NONE', *, *, #8740, .T. ) ;
#9590=AXIS2_PLACEMENT_3D ( 'NONE', #21940, #26880, #24413 ) ;
#9593=VERTEX_POINT ( 'NONE', #22259 ) ;
#9594=AXIS2_PLACEMENT_3D ( 'NONE', #20952, #618, #18168 ) ;
#9595=CARTESIAN_POINT ( 'NONE',  ( 33.46699938050304013, 28.47145308207318237, 47.04930799450050927 ) ) ;
#9597=EDGE_CURVE ( 'NONE', #16953, #20581, #10728, .T. ) ;
#9598=ADVANCED_FACE ( 'NONE', ( #597 ), #4427, .T. ) ;
#9606=DIRECTION ( 'NONE',  ( -1.000000000000000000, -1.101824276508909887E-16, 0.000000000000000000 ) ) ;
#9607=CARTESIAN_POINT ( 'NONE',  ( 8.823509210239574685, 30.59164230456639544, 47.04930799450051637 ) ) ;
#9610=CIRCLE ( 'NONE', #27958, 0.1250000000000001110 ) ;
#9615=AXIS2_PLACEMENT_3D ( 'NONE', #6683, #1758, #21123 ) ;
#9616=ORIENTED_EDGE ( 'NONE', *, *, #13826, .T. ) ;
#9619=CARTESIAN_POINT ( 'NONE',  ( 21.09992658989239089, 26.72145308207318948, 47.04930799450051637 ) ) ;
#9621=ORIENTED_EDGE ( 'NONE', *, *, #32083, .F. ) ;
#9624=ORIENTED_EDGE ( 'NONE', *, *, #1621, .T. ) ;
#9633=ORIENTED_EDGE ( 'NONE', *, *, #4301, .T. ) ;
#9634=FACE_OUTER_BOUND ( 'NONE', #9713, .T. ) ;
#9639=DIRECTION ( 'NONE',  ( -1.000000000000000000, 0.000000000000000000, 0.000000000000000000 ) ) ;
#9640=ORIENTED_EDGE ( 'NONE', *, *, #11266, .F. ) ;
#9661=ORIENTED_EDGE ( 'NONE', *, *, #10730, .F. ) ;
#9663=ORIENTED_EDGE ( 'NONE', *, *, #21357, .T. ) ;
#9665=CIRCLE ( 'NONE', #6515, 12.36707279061065101 ) ;
#9667=EDGE_CURVE ( 'NONE', #3138, #4416, #19619, .T. ) ;
#9673=ORIENTED_EDGE ( 'NONE', *, *, #976, .T. ) ;
#9674=EDGE_CURVE ( 'NONE', #13651, #30857, #30666, .T. ) ;
#9675=CIRCLE ( 'NONE', #30663, 0.1250000000000001110 ) ;
#9702=DIRECTION ( 'NONE',  ( -1.101824276508909887E-16, 1.000000000000000000, -0.000000000000000000 ) ) ;
#9708=CIRCLE ( 'NONE', #20167, 12.62506659569710266 ) ;
#9710=TOROIDAL_SURFACE ( 'NONE', #19127, 12.40141737965283575, 0.1250000000000000278 ) ;
#9711=AXIS2_PLACEMENT_3D ( 'NONE', #7041, #28890, #17044 ) ;
#9713=EDGE_LOOP ( 'NONE', ( #6244, #15193, #4596, #12695 ) ) ;
#9716=DIRECTION ( 'NONE',  ( -1.000000000000000000, -1.101824276508909764E-16, 0.000000000000000000 ) ) ;
#9725=DIRECTION ( 'NONE',  ( -1.000000000000000000, 0.000000000000000000, 0.000000000000000000 ) ) ;
#9732=AXIS2_PLACEMENT_3D ( 'NONE', #29216, #11336, #24124 ) ;
#9733=ORIENTED_EDGE ( 'NONE', *, *, #11167, .T. ) ;
#9734=EDGE_LOOP ( 'NONE', ( #17920, #24811, #14750, #5245 ) ) ;
#9746=ORIENTED_EDGE ( 'NONE', *, *, #20568, .F. ) ;
#9747=FACE_OUTER_BOUND ( 'NONE', #28582, .T. ) ;
#9749=DIRECTION ( 'NONE',  ( -1.101824276508909887E-16, 1.000000000000000000, -0.000000000000000000 ) ) ;
#9750=AXIS2_PLACEMENT_3D ( 'NONE', #21964, #4419, #19831 ) ;
#9751=FACE_OUTER_BOUND ( 'NONE', #19615, .T. ) ;
#9756=CIRCLE ( 'NONE', #28109, 12.62506659569710266 ) ;
#9758=VERTEX_POINT ( 'NONE', #16166 ) ;
#9761=ADVANCED_FACE ( 'NONE', ( #26178 ), #14918, .T. ) ;
#9766=ORIENTED_EDGE ( 'NONE', *, *, #13633, .F. ) ;
#9769=DIRECTION ( 'NONE',  ( -1.000000000000000000, -1.101824276508910010E-16, 0.000000000000000000 ) ) ;
#9774=CARTESIAN_POINT ( 'NONE',  ( 33.46699938050304013, 29.97145308207317527, 47.04930799450050927 ) ) ;
#9779=EDGE_LOOP ( 'NONE', ( #21840, #28367, #30816, #27592 ) ) ;
#9783=CARTESIAN_POINT ( 'NONE',  ( 33.71785032049137243, 25.46664230456640254, 47.04930799450051637 ) ) ;
#9784=AXIS2_PLACEMENT_3D ( 'NONE', #10991, #16696, #19160 ) ;
#9787=ORIENTED_EDGE ( 'NONE', *, *, #15564, .F. ) ;
#9788=ADVANCED_FACE ( 'NONE', ( #8631 ), #24337, .T. ) ;
#9790=EDGE_CURVE ( 'NONE', #19469, #5687, #16993, .T. ) ;
#9794=EDGE_CURVE ( 'NONE', #12904, #14845, #750, .T. ) ;
#9795=CIRCLE ( 'NONE', #13993, 12.62506659569710266 ) ;
#9810=CARTESIAN_POINT ( 'NONE',  ( 8.732853799281720342, 30.97145308207317171, 47.04930799450051637 ) ) ;
#9816=DIRECTION ( 'NONE',  ( -1.101824276508909887E-16, 1.000000000000000000, -0.000000000000000000 ) ) ;
#9818=ORIENTED_EDGE ( 'NONE', *, *, #30903, .F. ) ;
#9824=ORIENTED_EDGE ( 'NONE', *, *, #18018, .F. ) ;
#9825=ORIENTED_EDGE ( 'NONE', *, *, #19983, .F. ) ;
#9826=CARTESIAN_POINT ( 'NONE',  ( 21.09992658989239089, 25.34164230456639899, 47.04930799450051637 ) ) ;
#9836=EDGE_LOOP ( 'NONE', ( #27006, #24567, #9633, #2075 ) ) ;
#9838=DIRECTION ( 'NONE',  ( -1.101824276508909887E-16, 1.000000000000000000, -0.000000000000000000 ) ) ;
#9842=CIRCLE ( 'NONE', #31862, 12.36707279061065101 ) ;
#9843=ORIENTED_EDGE ( 'NONE', *, *, #27936, .T. ) ;
#9844=TOROIDAL_SURFACE ( 'NONE', #30283, 12.61792373059899397, 0.1249999999999959616 ) ;
#9857=ADVANCED_FACE ( 'NONE', ( #7260 ), #30235, .T. ) ;
#9859=CARTESIAN_POINT ( 'NONE',  ( 33.46699938050304013, 23.71183152705959429, 47.04930799450051637 ) ) ;
#9867=EDGE_CURVE ( 'NONE', #11837, #17879, #32249, .T. ) ;
#9884=DIRECTION ( 'NONE',  ( -1.101824276508909887E-16, 1.000000000000000000, -0.000000000000000000 ) ) ;
#9887=FACE_OUTER_BOUND ( 'NONE', #16254, .T. ) ;
#9892=AXIS2_PLACEMENT_3D ( 'NONE', #18616, #23874, #4345 ) ;
#9899=CARTESIAN_POINT ( 'NONE',  ( 21.09992658989239089, 27.09184655352419568, 47.04930799450051637 ) ) ;
#9901=FACE_OUTER_BOUND ( 'NONE', #4614, .T. ) ;
#9908=CIRCLE ( 'NONE', #18775, 12.36707279061065101 ) ;
#9911=ADVANCED_FACE ( 'NONE', ( #7092 ), #30078, .T. ) ;
#9914=ORIENTED_EDGE ( 'NONE', *, *, #4584, .F. ) ;
#9918=ORIENTED_EDGE ( 'NONE', *, *, #26671, .T. ) ;
#9922=AXIS2_PLACEMENT_3D ( 'NONE', #18837, #11314, #21302 ) ;
#9923=CARTESIAN_POINT ( 'NONE',  ( 21.09992658989239089, 29.96664230456641675, 47.04930799450051637 ) ) ;
#9924=ORIENTED_EDGE ( 'NONE', *, *, #4301, .F. ) ;
#9926=AXIS2_PLACEMENT_3D ( 'NONE', #25442, #30541, #17565 ) ;
#9929=ORIENTED_EDGE ( 'NONE', *, *, #13788, .F. ) ;
#9931=CYLINDRICAL_SURFACE ( 'NONE', #17387, 12.62506659569710266 ) ;
#9936=VERTEX_POINT ( 'NONE', #14650 ) ;
#9939=DIRECTION ( 'NONE',  ( -1.000000000000000000, 0.000000000000000000, 0.000000000000000000 ) ) ;
#9940=VECTOR ( 'NONE', #23555, 1000.000000000000000 ) ;
#9943=CARTESIAN_POINT ( 'NONE',  ( 21.09992658989238734, 31.59164230456639544, 47.04930799450051637 ) ) ;
#9946=ADVANCED_FACE ( 'NONE', ( #32209 ), #24887, .T. ) ;
#9948=VERTEX_POINT ( 'NONE', #19718 ) ;
#9950=EDGE_CURVE ( 'NONE', #112, #4576, #29073, .T. ) ;
#9953=AXIS2_PLACEMENT_3D ( 'NONE', #28956, #29113, #8449 ) ;
#9956=AXIS2_PLACEMENT_3D ( 'NONE', #21197, #18577, #1186 ) ;
#9961=DIRECTION ( 'NONE',  ( 0.000000000000000000, -0.000000000000000000, -1.000000000000000000 ) ) ;
#9963=DIRECTION ( 'NONE',  ( -1.101824276508909887E-16, 1.000000000000000000, -0.000000000000000000 ) ) ;
#9964=EDGE_CURVE ( 'NONE', #30197, #12497, #9708, .T. ) ;
#9967=ORIENTED_EDGE ( 'NONE', *, *, #4398, .F. ) ;
#9970=VERTEX_POINT ( 'NONE', #12688 ) ;
#9973=AXIS2_PLACEMENT_3D ( 'NONE', #7180, #119, #19314 ) ;
#9974=AXIS2_PLACEMENT_3D ( 'NONE', #17248, #27264, #14808 ) ;
#9975=DIRECTION ( 'NONE',  ( -1.000000000000000000, 0.000000000000000000, 0.000000000000000000 ) ) ;
#9976=DIRECTION ( 'NONE',  ( -1.101824276508909887E-16, 1.000000000000000000, -0.000000000000000000 ) ) ;
#9977=DIRECTION ( 'NONE',  ( -1.000000000000000000, 0.000000000000000000, 0.000000000000000000 ) ) ;
#9979=AXIS2_PLACEMENT_3D ( 'NONE', #30441, #17469, #7958 ) ;
#9980=DIRECTION ( 'NONE',  ( -1.000000000000000000, 0.000000000000000000, 0.000000000000000000 ) ) ;
#9981=CARTESIAN_POINT ( 'NONE',  ( 8.698509210239574685, 30.59164230456639544, 47.04930799450051637 ) ) ;
#9983=AXIS2_PLACEMENT_3D ( 'NONE', #8578, #28757, #3972 ) ;
#9986=DIRECTION ( 'NONE',  ( -1.000000000000000000, -1.101824276508909887E-16, 0.000000000000000000 ) ) ;
#9987=ORIENTED_EDGE ( 'NONE', *, *, #21170, .T. ) ;
#9993=EDGE_CURVE ( 'NONE', #14845, #11669, #16512, .T. ) ;
#9998=AXIS2_PLACEMENT_3D ( 'NONE', #31047, #8556, #18545 ) ;
#10000=CIRCLE ( 'NONE', #13678, 12.36707279061065101 ) ;
#10004=ADVANCED_FACE ( 'NONE', ( #20363 ), #20715, .T. ) ;
#10007=CARTESIAN_POINT ( 'NONE',  ( 21.09992658989239089, 26.34164230456639899, 47.04930799450051637 ) ) ;
#10012=EDGE_LOOP ( 'NONE', ( #19434, #16526, #19649, #12978 ) ) ;
#10018=DIRECTION ( 'NONE',  ( -1.101824276508909887E-16, 1.000000000000000000, -0.000000000000000000 ) ) ;
#10025=LINE ( 'NONE', #19855, #20843 ) ;
#10026=DIRECTION ( 'NONE',  ( -1.101824276508909887E-16, 1.000000000000000000, -0.000000000000000000 ) ) ;
#10031=FACE_OUTER_BOUND ( 'NONE', #19331, .T. ) ;
#10041=CARTESIAN_POINT ( 'NONE',  ( 21.09992658989239089, 27.97145308207318237, 47.04930799450051637 ) ) ;
#10049=FACE_OUTER_BOUND ( 'NONE', #28338, .T. ) ;
#10059=FACE_OUTER_BOUND ( 'NONE', #7890, .T. ) ;
#10061=( LENGTH_UNIT ( ) NAMED_UNIT ( * ) SI_UNIT ( .MILLI., .METRE. ) );
#10062=EDGE_LOOP ( 'NONE', ( #16715, #11502, #26600, #2459 ) ) ;
#10065=CIRCLE ( 'NONE', #26823, 0.1250000000000001110 ) ;
#10066=DIRECTION ( 'NONE',  ( 1.000000000000000000, 0.000000000000000000, 0.000000000000000000 ) ) ;
#10069=VERTEX_POINT ( 'NONE', #30723 ) ;
#10074=VERTEX_POINT ( 'NONE', #25782 ) ;
#10081=DIRECTION ( 'NONE',  ( 0.000000000000000000, -0.000000000000000000, -1.000000000000000000 ) ) ;
#10084=ADVANCED_FACE ( 'NONE', ( #18389 ), #9163, .T. ) ;
#10085=DIRECTION ( 'NONE',  ( -1.000000000000000000, -1.101824276508909764E-16, 0.000000000000000000 ) ) ;
#10086=AXIS2_PLACEMENT_3D ( 'NONE', #16975, #21741, #7309 ) ;
#10090=DIRECTION ( 'NONE',  ( -1.101824276508909887E-16, 1.000000000000000000, -0.000000000000000000 ) ) ;
#10092=ADVANCED_FACE ( 'NONE', ( #28419 ), #25421, .T. ) ;
#10093=TOROIDAL_SURFACE ( 'NONE', #135, 12.61792373059899752, 0.1250000000000005274 ) ;
#10096=EDGE_LOOP ( 'NONE', ( #11120, #30438, #30015, #18816 ) ) ;
#10098=FACE_OUTER_BOUND ( 'NONE', #2920, .T. ) ;
#10099=CARTESIAN_POINT ( 'NONE',  ( 33.50134396954519644, 31.34164230456639544, 47.04930799450051637 ) ) ;
#10100=AXIS2_PLACEMENT_3D ( 'NONE', #2437, #8016, #12453 ) ;
#10102=ORIENTED_EDGE ( 'NONE', *, *, #18733, .T. ) ;
#10110=DIRECTION ( 'NONE',  ( -1.000000000000000000, 0.000000000000000000, 0.000000000000000000 ) ) ;
#10112=DIRECTION ( 'NONE',  ( -1.101824276508909887E-16, 1.000000000000000000, -0.000000000000000000 ) ) ;
#10115=VERTEX_POINT ( 'NONE', #15934 ) ;
#10116=CARTESIAN_POINT ( 'NONE',  ( 8.823509210239532052, 26.59164230456639899, 47.04930799450051637 ) ) ;
#10121=CARTESIAN_POINT ( 'NONE',  ( 8.698509210239564027, 29.59164230456639899, 47.04930799450051637 ) ) ;
#10126=DIRECTION ( 'NONE',  ( -1.000000000000000000, 0.000000000000000000, 0.000000000000000000 ) ) ;
#10133=CARTESIAN_POINT ( 'NONE',  ( 21.09992658989238734, 32.34143805560860585, 47.04930799450051637 ) ) ;
#10135=ORIENTED_EDGE ( 'NONE', *, *, #29541, .T. ) ;
#10140=CARTESIAN_POINT ( 'NONE',  ( 8.698509210239516065, 25.09164230456639899, 47.04930799450051637 ) ) ;
#10148=CARTESIAN_POINT ( 'NONE',  ( 8.698509210239571132, 30.34164230456639544, 47.04930799450051637 ) ) ;
#10150=CARTESIAN_POINT ( 'NONE',  ( 21.09992658989239089, 26.09164230456639899, 47.04930799450051637 ) ) ;
#10154=ORIENTED_EDGE ( 'NONE', *, *, #22616, .F. ) ;
#10157=TOROIDAL_SURFACE ( 'NONE', #16950, 12.40141737965280022, 0.1249999999999992228 ) ;
#10160=CIRCLE ( 'NONE', #31639, 12.62506659569710266 ) ;
#10184=ORIENTED_EDGE ( 'NONE', *, *, #2716, .F. ) ;
#10192=DIRECTION ( 'NONE',  ( -1.000000000000000000, 0.000000000000000000, 0.000000000000000000 ) ) ;
#10194=CARTESIAN_POINT ( 'NONE',  ( 33.46699938050303302, 38.56284415653841791, 47.04930799450051637 ) ) ;
#10200=AXIS2_PLACEMENT_3D ( 'NONE', #23401, #20930, #31278 ) ;
#10208=DIRECTION ( 'NONE',  ( -1.000000000000000000, 0.000000000000000000, 0.000000000000000000 ) ) ;
#10209=DIRECTION ( 'NONE',  ( -1.101824276508909887E-16, 1.000000000000000000, -0.000000000000000000 ) ) ;
#10210=ADVANCED_FACE ( 'NONE', ( #31688 ), #1314, .F. ) ;
#10218=CARTESIAN_POINT ( 'NONE',  ( 8.823509210239517842, 25.34164230456639899, 47.04930799450051637 ) ) ;
#10220=ORIENTED_EDGE ( 'NONE', *, *, #9674, .T. ) ;
#10222=DIRECTION ( 'NONE',  ( -1.101824276508909887E-16, 1.000000000000000000, -0.000000000000000000 ) ) ;
#10229=CARTESIAN_POINT ( 'NONE',  ( 8.474859994195286461, 29.09184655352418858, 47.04930799450051637 ) ) ;
#10230=CARTESIAN_POINT ( 'NONE',  ( 33.37634396954526750, 24.59164230456639544, 47.04930799450051637 ) ) ;
#10235=AXIS2_PLACEMENT_3D ( 'NONE', #7431, #14974, #17423 ) ;
#10238=CIRCLE ( 'NONE', #18062, 0.1250000000000001110 ) ;
#10246=ORIENTED_EDGE ( 'NONE', *, *, #10487, .F. ) ;
#10247=EDGE_CURVE ( 'NONE', #14930, #7136, #8601, .T. ) ;
#10250=CIRCLE ( 'NONE', #5540, 12.27641737965286062 ) ;
#10252=DIRECTION ( 'NONE',  ( -1.101824276508909887E-16, 1.000000000000000000, -0.000000000000000000 ) ) ;
#10253=VECTOR ( 'NONE', #28691, 1000.000000000000000 ) ;
#10255=TOROIDAL_SURFACE ( 'NONE', #2883, 12.61792373059858896, 0.1250000000000002220 ) ;
#10263=CARTESIAN_POINT ( 'NONE',  ( 21.09992658989238734, 38.56284415653841791, 47.04930799450051637 ) ) ;
#10266=LINE ( 'NONE', #31087, #24405 ) ;
#10269=CARTESIAN_POINT ( 'NONE',  ( 21.09992658989239089, 29.84143805560861296, 47.04930799450051637 ) ) ;
#10274=EDGE_CURVE ( 'NONE', #24129, #18133, #17060, .T. ) ;
#10277=DIRECTION ( 'NONE',  ( -1.101824276508909887E-16, 1.000000000000000000, -0.000000000000000000 ) ) ;
#10278=EDGE_CURVE ( 'NONE', #4416, #3138, #11812, .T. ) ;
#10279=CARTESIAN_POINT ( 'NONE',  ( 21.09992658989238734, 38.56284415653841791, 47.04930799450051637 ) ) ;
#10283=AXIS2_PLACEMENT_3D ( 'NONE', #16776, #26799, #4314 ) ;
#10293=CARTESIAN_POINT ( 'NONE',  ( 33.71785032049138664, 24.21664230456639899, 47.04930799450051637 ) ) ;
#10296=DIRECTION ( 'NONE',  ( -1.000000000000000000, 0.000000000000000000, 0.000000000000000000 ) ) ;
#10297=ORIENTED_EDGE ( 'NONE', *, *, #6214, .T. ) ;
#10310=DIRECTION ( 'NONE',  ( -1.000000000000000000, 0.000000000000000000, 0.000000000000000000 ) ) ;
#10312=FACE_OUTER_BOUND ( 'NONE', #16966, .T. ) ;
#10314=AXIS2_PLACEMENT_3D ( 'NONE', #13871, #16803, #6315 ) ;
#10316=ORIENTED_EDGE ( 'NONE', *, *, #14277, .F. ) ;
#10317=ORIENTED_EDGE ( 'NONE', *, *, #16585, .T. ) ;
#10322=AXIS2_PLACEMENT_3D ( 'NONE', #18194, #3270, #28066 ) ;
#10325=AXIS2_PLACEMENT_3D ( 'NONE', #7578, #15123, #6921 ) ;
#10329=DIRECTION ( 'NONE',  ( -1.101824276508909887E-16, 1.000000000000000000, -0.000000000000000000 ) ) ;
#10331=ORIENTED_EDGE ( 'NONE', *, *, #9667, .F. ) ;
#10344=DIRECTION ( 'NONE',  ( -1.000000000000000000, 0.000000000000000000, 0.000000000000000000 ) ) ;
#10348=CARTESIAN_POINT ( 'NONE',  ( 8.698509210239569356, 30.09164230456639544, 47.04930799450051637 ) ) ;
#10350=CARTESIAN_POINT ( 'NONE',  ( 8.474859994195281132, 31.59143805560860585, 47.04930799450051637 ) ) ;
#10352=ADVANCED_FACE ( 'NONE', ( #15259 ), #7220, .F. ) ;
#10353=ADVANCED_FACE ( 'NONE', ( #17221 ), #13394, .T. ) ;
#10355=EDGE_LOOP ( 'NONE', ( #10732, #12402, #16198, #8575 ) ) ;
#10356=VECTOR ( 'NONE', #16087, 1000.000000000000000 ) ;
#10359=AXIS2_PLACEMENT_3D ( 'NONE', #28741, #693, #23178 ) ;
#10361=DIRECTION ( 'NONE',  ( -1.101824276508909887E-16, 1.000000000000000000, -0.000000000000000000 ) ) ;
#10365=VECTOR ( 'NONE', #18591, 1000.000000000000000 ) ;
#10368=DIRECTION ( 'NONE',  ( -1.000000000000000000, 0.000000000000000000, 0.000000000000000000 ) ) ;
#10370=CIRCLE ( 'NONE', #409, 12.62506659569710266 ) ;
#10379=ADVANCED_FACE ( 'NONE', ( #7554 ), #15998, .T. ) ;
#10383=CARTESIAN_POINT ( 'NONE',  ( 21.09992658989239089, 28.21664230456639899, 47.04930799450051637 ) ) ;
#10384=ORIENTED_EDGE ( 'NONE', *, *, #12418, .T. ) ;
#10385=CARTESIAN_POINT ( 'NONE',  ( 8.698509210239542710, 27.59164230456639544, 47.04930799450051637 ) ) ;
#10394=CIRCLE ( 'NONE', #28720, 12.62506659569710266 ) ;
#10396=TOROIDAL_SURFACE ( 'NONE', #28722, 12.61792373059858541, 0.1250000000000004996 ) ;
#10397=DIRECTION ( 'NONE',  ( -1.101824276508909887E-16, 1.000000000000000000, -0.000000000000000000 ) ) ;
#10398=AXIS2_PLACEMENT_3D ( 'NONE', #26560, #14261, #9002 ) ;
#10399=ADVANCED_FACE ( 'NONE', ( #27732 ), #1330, .T. ) ;
#10402=CARTESIAN_POINT ( 'NONE',  ( 21.09992658989239089, 24.59164230456639544, 47.04930799450051637 ) ) ;
#10406=FACE_OUTER_BOUND ( 'NONE', #29476, .T. ) ;
#10410=AXIS2_PLACEMENT_3D ( 'NONE', #30058, #25123, #5265 ) ;
#10412=DIRECTION ( 'NONE',  ( -1.101824276508909887E-16, 1.000000000000000000, -0.000000000000000000 ) ) ;
#10415=CARTESIAN_POINT ( 'NONE',  ( 8.698509210239501854, 23.59164230456639544, 47.04930799450051637 ) ) ;
#10420=EDGE_CURVE ( 'NONE', #414, #17658, #22743, .T. ) ;
#10423=EDGE_CURVE ( 'NONE', #32103, #1121, #11225, .T. ) ;
#10428=ORIENTED_EDGE ( 'NONE', *, *, #20755, .T. ) ;
#10435=FACE_OUTER_BOUND ( 'NONE', #8198, .T. ) ;
#10436=ORIENTED_EDGE ( 'NONE', *, *, #19337, .F. ) ;
#10437=DIRECTION ( 'NONE',  ( -1.000000000000000000, -1.101824276508909887E-16, 0.000000000000000000 ) ) ;
#10439=EDGE_CURVE ( 'NONE', #21770, #13402, #31151, .T. ) ;
#10452=CYLINDRICAL_SURFACE ( 'NONE', #8874, 12.36707279061065101 ) ;
#10454=DIRECTION ( 'NONE',  ( -1.101824276508909887E-16, 1.000000000000000000, -0.000000000000000000 ) ) ;
#10455=DIRECTION ( 'NONE',  ( -1.224646799147353207E-16, -1.349345573449484691E-32, 1.000000000000000000 ) ) ;
#10458=DIRECTION ( 'NONE',  ( -1.101824276508909887E-16, 1.000000000000000000, -0.000000000000000000 ) ) ;
#10461=AXIS2_PLACEMENT_3D ( 'NONE', #19301, #1754, #18811 ) ;
#10473=VERTEX_POINT ( 'NONE', #16689 ) ;
#10474=DIRECTION ( 'NONE',  ( -1.101824276508909887E-16, 1.000000000000000000, -0.000000000000000000 ) ) ;
#10475=EDGE_LOOP ( 'NONE', ( #10943, #7638, #20279, #11380 ) ) ;
#10480=TOROIDAL_SURFACE ( 'NONE', #7326, 12.40141737965281266, 0.1249999999999994865 ) ;
#10482=DIRECTION ( 'NONE',  ( -1.101824276508909887E-16, 1.000000000000000000, -0.000000000000000000 ) ) ;
#10483=CIRCLE ( 'NONE', #19379, 0.1250000000000001110 ) ;
#10486=ORIENTED_EDGE ( 'NONE', *, *, #26716, .F. ) ;
#10487=EDGE_CURVE ( 'NONE', #9009, #13651, #7626, .T. ) ;
#10489=CIRCLE ( 'NONE', #9973, 12.36707279061065101 ) ;
#10494=DIRECTION ( 'NONE',  ( -1.000000000000000000, 0.000000000000000000, 0.000000000000000000 ) ) ;
#10495=DIRECTION ( 'NONE',  ( -1.000000000000000000, 0.000000000000000000, 0.000000000000000000 ) ) ;
#10497=TOROIDAL_SURFACE ( 'NONE', #14690, 12.61792373059893713, 0.1249999999999992506 ) ;
#10498=TOROIDAL_SURFACE ( 'NONE', #31993, 12.40141737965287305, 0.1250000000000000833 ) ;
#10499=ORIENTED_EDGE ( 'NONE', *, *, #13989, .T. ) ;
#10501=CARTESIAN_POINT ( 'NONE',  ( 21.09992658989239089, 25.34164230456639899, 47.04930799450051637 ) ) ;
#10502=EDGE_CURVE ( 'NONE', #27701, #30925, #26232, .T. ) ;
#10516=ORIENTED_EDGE ( 'NONE', *, *, #27802, .F. ) ;
#10518=CYLINDRICAL_SURFACE ( 'NONE', #13039, 12.62506659569710266 ) ;
#10524=AXIS2_PLACEMENT_3D ( 'NONE', #8790, #23731, #6021 ) ;
#10527=ORIENTED_EDGE ( 'NONE', *, *, #15821, .F. ) ;
#10530=DIRECTION ( 'NONE',  ( -1.101824276508909887E-16, 1.000000000000000000, -0.000000000000000000 ) ) ;
#10531=AXIS2_PLACEMENT_3D ( 'NONE', #17916, #20698, #25784 ) ;
#10534=LINE ( 'NONE', #30558, #1825 ) ;
#10536=DIRECTION ( 'NONE',  ( -1.000000000000000000, 0.000000000000000000, 0.000000000000000000 ) ) ;
#10538=CIRCLE ( 'NONE', #14708, 12.36707279061065279 ) ;
#10544=DIRECTION ( 'NONE',  ( -1.000000000000000000, 0.000000000000000000, 0.000000000000000000 ) ) ;
#10549=DIRECTION ( 'NONE',  ( -1.000000000000000000, -1.101824276508910010E-16, 0.000000000000000000 ) ) ;
#10552=ORIENTED_EDGE ( 'NONE', *, *, #18773, .T. ) ;
#10557=FACE_OUTER_BOUND ( 'NONE', #16144, .T. ) ;
#10558=ORIENTED_EDGE ( 'NONE', *, *, #25932, .F. ) ;
#10561=ORIENTED_EDGE ( 'NONE', *, *, #8853, .T. ) ;
#10565=TOROIDAL_SURFACE ( 'NONE', #19988, 12.40141737965285706, 0.1250000000000007494 ) ;
#10569=CIRCLE ( 'NONE', #14236, 12.36707279061065101 ) ;
#10570=AXIS2_PLACEMENT_3D ( 'NONE', #10263, #20411, #20250 ) ;
#10571=FACE_OUTER_BOUND ( 'NONE', #568, .T. ) ;
#10577=CARTESIAN_POINT ( 'NONE',  ( 33.46699938050304013, 23.72145308207319658, 47.04930799450050927 ) ) ;
#10578=CIRCLE ( 'NONE', #7982, 12.62506659569710266 ) ;
#10586=FACE_OUTER_BOUND ( 'NONE', #10823, .T. ) ;
#10587=EDGE_CURVE ( 'NONE', #22169, #154, #26395, .T. ) ;
#10589=EDGE_LOOP ( 'NONE', ( #4231, #32243, #8476, #15110 ) ) ;
#10590=CARTESIAN_POINT ( 'NONE',  ( 8.732853799281729223, 26.47145308207318593, 47.04930799450051637 ) ) ;
#10591=LINE ( 'NONE', #30928, #2707 ) ;
#10592=ADVANCED_FACE ( 'NONE', ( #21451 ), #31487, .F. ) ;
#10598=CIRCLE ( 'NONE', #26833, 0.1250000000000001110 ) ;
#10604=DIRECTION ( 'NONE',  ( -1.000000000000000000, -1.101824276508909887E-16, 0.000000000000000000 ) ) ;
#10607=ORIENTED_EDGE ( 'NONE', *, *, #22624, .F. ) ;
#10616=TOROIDAL_SURFACE ( 'NONE', #23713, 12.40141737965282154, 0.1250000000000006939 ) ;
#10618=CARTESIAN_POINT ( 'NONE',  ( 21.09992658989238734, 31.09164230456639544, 47.04930799450051637 ) ) ;
#10621=CARTESIAN_POINT ( 'NONE',  ( 33.72499318558949000, 38.56284415653841791, 47.04930799450051637 ) ) ;
#10626=DIRECTION ( 'NONE',  ( -1.000000000000000000, 0.000000000000000000, 0.000000000000000000 ) ) ;
#10629=CARTESIAN_POINT ( 'NONE',  ( 21.09992658989239089, 29.21664230456640254, 47.04930799450051637 ) ) ;
#10640=DIRECTION ( 'NONE',  ( -1.000000000000000000, 0.000000000000000000, 0.000000000000000000 ) ) ;
#10642=AXIS2_PLACEMENT_3D ( 'NONE', #14771, #12472, #29869 ) ;
#10643=EDGE_LOOP ( 'NONE', ( #9914, #24050, #1133, #6024 ) ) ;
#10645=AXIS2_PLACEMENT_3D ( 'NONE', #3380, #21253, #30800 ) ;
#10649=ADVANCED_FACE ( 'NONE', ( #4554 ), #120, .F. ) ;
#10655=EDGE_CURVE ( 'NONE', #17361, #1375, #7872, .T. ) ;
#10657=VECTOR ( 'NONE', #281, 1000.000000000000000 ) ;
#10660=DIRECTION ( 'NONE',  ( -1.000000000000000000, 0.000000000000000000, 0.000000000000000000 ) ) ;
#10661=VERTEX_POINT ( 'NONE', #4392 ) ;
#10666=CARTESIAN_POINT ( 'NONE',  ( 21.09992658989239089, 26.96664230456639899, 47.04930799450051637 ) ) ;
#10670=ORIENTED_EDGE ( 'NONE', *, *, #20568, .T. ) ;
#10671=EDGE_LOOP ( 'NONE', ( #27517, #1020, #18088, #12924 ) ) ;
#10675=DIRECTION ( 'NONE',  ( -1.000000000000000000, 0.000000000000000000, 0.000000000000000000 ) ) ;
#10679=ORIENTED_EDGE ( 'NONE', *, *, #15375, .F. ) ;
#10680=DIRECTION ( 'NONE',  ( -1.101824276508909887E-16, 1.000000000000000000, -0.000000000000000000 ) ) ;
#10681=CARTESIAN_POINT ( 'NONE',  ( 8.698509210239560474, 29.34164230456639899, 47.04930799450051637 ) ) ;
#10684=CARTESIAN_POINT ( 'NONE',  ( 8.698509210239555145, 28.84164230456639544, 47.04930799450051637 ) ) ;
#10687=VERTEX_POINT ( 'NONE', #29675 ) ;
#10689=CARTESIAN_POINT ( 'NONE',  ( 8.732853799281734553, 38.56284415653841791, 47.04930799450051637 ) ) ;
#10692=CIRCLE ( 'NONE', #11207, 0.1250000000000001110 ) ;
#10697=VERTEX_POINT ( 'NONE', #11944 ) ;
#10700=DIRECTION ( 'NONE',  ( -1.000000000000000000, 0.000000000000000000, 0.000000000000000000 ) ) ;
#10702=VERTEX_POINT ( 'NONE', #29514 ) ;
#10704=LINE ( 'NONE', #13159, #8114 ) ;
#10707=DIRECTION ( 'NONE',  ( -1.101824276508909887E-16, 1.000000000000000000, -0.000000000000000000 ) ) ;
#10708=CIRCLE ( 'NONE', #16444, 0.1250000000000001110 ) ;
#10711=CYLINDRICAL_SURFACE ( 'NONE', #6833, 12.62506659569710266 ) ;
#10712=CARTESIAN_POINT ( 'NONE',  ( 21.09992658989239089, 27.84184655352419568, 47.04930799450051637 ) ) ;
#10716=DIRECTION ( 'NONE',  ( -1.000000000000000000, -1.101824276508909887E-16, 0.000000000000000000 ) ) ;
#10719=DIRECTION ( 'NONE',  ( -1.101824276508909887E-16, 1.000000000000000000, -0.000000000000000000 ) ) ;
#10726=TOROIDAL_SURFACE ( 'NONE', #29594, 12.40141737965286772, 0.1250000000000003331 ) ;
#10728=CIRCLE ( 'NONE', #2322, 12.36707279061065279 ) ;
#10729=CIRCLE ( 'NONE', #15954, 0.1250000000000001110 ) ;
#10730=EDGE_CURVE ( 'NONE', #13336, #21573, #32137, .T. ) ;
#10732=ORIENTED_EDGE ( 'NONE', *, *, #20720, .F. ) ;
#10734=CARTESIAN_POINT ( 'NONE',  ( 8.698509210239544487, 27.84164230456639544, 47.04930799450051637 ) ) ;
#10735=DIRECTION ( 'NONE',  ( 1.000000000000000000, 0.000000000000000000, 0.000000000000000000 ) ) ;
#10739=CARTESIAN_POINT ( 'NONE',  ( 8.474859994195286461, 27.84143805560860940, 47.04930799450051637 ) ) ;
#10740=ORIENTED_EDGE ( 'NONE', *, *, #18692, .T. ) ;
#10750=DIRECTION ( 'NONE',  ( -1.224646799147353207E-16, -1.349345573449484691E-32, 1.000000000000000000 ) ) ;
#10754=CARTESIAN_POINT ( 'NONE',  ( 33.46699938050303302, 38.56284415653841791, 47.04930799450051637 ) ) ;
#10766=EDGE_LOOP ( 'NONE', ( #9140, #8729, #24408, #8503 ) ) ;
#10769=ORIENTED_EDGE ( 'NONE', *, *, #19661, .F. ) ;
#10770=ADVANCED_FACE ( 'NONE', ( #2427 ), #10497, .T. ) ;
#10775=CIRCLE ( 'NONE', #23345, 12.36707279061065101 ) ;
#10780=DIRECTION ( 'NONE',  ( -1.101824276508909887E-16, 1.000000000000000000, -0.000000000000000000 ) ) ;
#10785=CARTESIAN_POINT ( 'NONE',  ( 8.474859994195282908, 38.56284415653841791, 47.04930799450051637 ) ) ;
#10790=DIRECTION ( 'NONE',  ( -1.101824276508909887E-16, 1.000000000000000000, -0.000000000000000000 ) ) ;
#10791=ORIENTED_EDGE ( 'NONE', *, *, #16067, .T. ) ;
#10792=CARTESIAN_POINT ( 'NONE',  ( 33.72499318558949710, 28.59143805560861296, 47.04930799450051637 ) ) ;
#10794=DIRECTION ( 'NONE',  ( -1.000000000000000000, 0.000000000000000000, 0.000000000000000000 ) ) ;
#10801=VERTEX_POINT ( 'NONE', #7682 ) ;
#10805=EDGE_CURVE ( 'NONE', #4648, #24129, #6359, .T. ) ;
#10807=DIRECTION ( 'NONE',  ( -1.000000000000000000, 0.000000000000000000, 0.000000000000000000 ) ) ;
#10812=AXIS2_PLACEMENT_3D ( 'NONE', #25615, #3117, #13154 ) ;
#10814=EDGE_CURVE ( 'NONE', #20369, #3968, #20293, .T. ) ;
#10815=ORIENTED_EDGE ( 'NONE', *, *, #14277, .T. ) ;
#10817=AXIS2_PLACEMENT_3D ( 'NONE', #31368, #8873, #31693 ) ;
#10820=CARTESIAN_POINT ( 'NONE',  ( 21.09992658989239089, 24.09164230456639544, 47.04930799450051637 ) ) ;
#10823=EDGE_LOOP ( 'NONE', ( #16705, #20310, #20252, #8866 ) ) ;
#10825=DIRECTION ( 'NONE',  ( 1.000000000000000000, 0.000000000000000000, 0.000000000000000000 ) ) ;
#10831=CARTESIAN_POINT ( 'NONE',  ( 21.09992658989239089, 26.84164230456639899, 47.04930799450051637 ) ) ;
#10832=CARTESIAN_POINT ( 'NONE',  ( 8.823509210239537381, 27.09164230456639899, 47.04930799450051637 ) ) ;
#10835=CARTESIAN_POINT ( 'NONE',  ( 21.09992658989239089, 30.59164230456639544, 47.04930799450051637 ) ) ;
#10837=CARTESIAN_POINT ( 'NONE',  ( 21.09992658989238734, 38.56284415653841791, 47.04930799450051637 ) ) ;
#10838=EDGE_CURVE ( 'NONE', #15078, #25895, #5213, .T. ) ;
#10841=ORIENTED_EDGE ( 'NONE', *, *, #11394, .F. ) ;
#10844=TOROIDAL_SURFACE ( 'NONE', #10322, 12.61792373059894601, 0.1249999999999988065 ) ;
#10847=EDGE_CURVE ( 'NONE', #20651, #15854, #17367, .T. ) ;
#10848=AXIS2_PLACEMENT_3D ( 'NONE', #22313, #17386, #5084 ) ;
#10852=FACE_OUTER_BOUND ( 'NONE', #7529, .T. ) ;
#10860=CARTESIAN_POINT ( 'NONE',  ( 8.474859994195281132, 32.34184655352418503, 47.04930799450051637 ) ) ;
#10865=DIRECTION ( 'NONE',  ( -1.000000000000000000, -1.101824276508910010E-16, 0.000000000000000000 ) ) ;
#10873=AXIS2_PLACEMENT_3D ( 'NONE', #21739, #29140, #23725 ) ;
#10874=ADVANCED_FACE ( 'NONE', ( #15700 ), #15732, .T. ) ;
#10883=CIRCLE ( 'NONE', #11918, 0.1249999999999983763 ) ;
#10891=CYLINDRICAL_SURFACE ( 'NONE', #4620, 12.62506659569710443 ) ;
#10892=EDGE_CURVE ( 'NONE', #27923, #16423, #13709, .T. ) ;
#10902=CARTESIAN_POINT ( 'NONE',  ( 33.50134396954522487, 28.84164230456639544, 47.04930799450051637 ) ) ;
#10904=DIRECTION ( 'NONE',  ( -1.000000000000000000, 0.000000000000000000, 0.000000000000000000 ) ) ;
#10909=CARTESIAN_POINT ( 'NONE',  ( 8.474859994195286461, 28.59143805560861296, 47.04930799450051637 ) ) ;
#10910=CARTESIAN_POINT ( 'NONE',  ( 8.823509210239517842, 25.09164230456639899, 47.04930799450051637 ) ) ;
#10912=CIRCLE ( 'NONE', #11432, 12.36707279061065101 ) ;
#10917=CARTESIAN_POINT ( 'NONE',  ( 21.09992658989238734, 38.56284415653841791, 47.04930799450051637 ) ) ;
#10918=CARTESIAN_POINT ( 'NONE',  ( 21.09992658989239089, 28.97145308207318237, 47.04930799450051637 ) ) ;
#10922=VERTEX_POINT ( 'NONE', #8484 ) ;
#10923=CIRCLE ( 'NONE', #31377, 12.62506659569710266 ) ;
#10929=CARTESIAN_POINT ( 'NONE',  ( 21.09992658989239089, 24.84164230456639544, 47.04930799450051637 ) ) ;
#10934=DIRECTION ( 'NONE',  ( 0.000000000000000000, -0.000000000000000000, -1.000000000000000000 ) ) ;
#10936=CARTESIAN_POINT ( 'NONE',  ( 8.474859994195281132, 31.59184655352418503, 47.04930799450051637 ) ) ;
#10941=CARTESIAN_POINT ( 'NONE',  ( 8.573509210239590672, 32.59164230456639899, 47.04930799450051637 ) ) ;
#10943=ORIENTED_EDGE ( 'NONE', *, *, #22450, .F. ) ;
#10945=EDGE_CURVE ( 'NONE', #19345, #8205, #6658, .T. ) ;
#10946=CARTESIAN_POINT ( 'NONE',  ( 21.09992658989238734, 30.97145308207317171, 47.04930799450051637 ) ) ;
#10949=ADVANCED_FACE ( 'NONE', ( #20943 ), #7946, .T. ) ;
#10951=EDGE_CURVE ( 'NONE', #29220, #104, #4795, .T. ) ;
#10952=EDGE_LOOP ( 'NONE', ( #10978, #24728, #20216, #18278 ) ) ;
#10953=CARTESIAN_POINT ( 'NONE',  ( 33.72499318558949710, 27.34143805560860940, 47.04930799450051637 ) ) ;
#10958=CIRCLE ( 'NONE', #29256, 0.1250000000000001110 ) ;
#10965=AXIS2_PLACEMENT_3D ( 'NONE', #29392, #29562, #11836 ) ;
#10969=CARTESIAN_POINT ( 'NONE',  ( 21.09992658989239089, 27.46183152705960850, 47.04930799450051637 ) ) ;
#10978=ORIENTED_EDGE ( 'NONE', *, *, #14168, .F. ) ;
#10981=CARTESIAN_POINT ( 'NONE',  ( 33.37634396954528171, 23.84164230456639544, 47.04930799450051637 ) ) ;
#10985=EDGE_CURVE ( 'NONE', #5223, #272, #31477, .T. ) ;
#10987=DIRECTION ( 'NONE',  ( -1.224646799147353207E-16, -1.349345573449484691E-32, 1.000000000000000000 ) ) ;
#10991=CARTESIAN_POINT ( 'NONE',  ( 21.09992658989239089, 24.84184655352419213, 47.04930799450051637 ) ) ;
#10996=ORIENTED_EDGE ( 'NONE', *, *, #4018, .T. ) ;
#11004=CIRCLE ( 'NONE', #18821, 0.1250000000000001110 ) ;
#11010=DIRECTION ( 'NONE',  ( -1.000000000000000000, 0.000000000000000000, 0.000000000000000000 ) ) ;
#11012=EDGE_CURVE ( 'NONE', #16025, #28129, #26518, .T. ) ;
#11013=ORIENTED_EDGE ( 'NONE', *, *, #18640, .F. ) ;
#11017=VERTEX_POINT ( 'NONE', #16336 ) ;
#11020=EDGE_LOOP ( 'NONE', ( #11488, #19697, #21229, #9239 ) ) ;
#11021=DIRECTION ( 'NONE',  ( -1.000000000000000000, 0.000000000000000000, 0.000000000000000000 ) ) ;
#11024=CARTESIAN_POINT ( 'NONE',  ( 33.37634396954523908, 27.34164230456639544, 47.04930799450051637 ) ) ;
#11027=ORIENTED_EDGE ( 'NONE', *, *, #27505, .T. ) ;
#11028=ORIENTED_EDGE ( 'NONE', *, *, #14276, .F. ) ;
#11029=CARTESIAN_POINT ( 'NONE',  ( 33.72499318558949000, 38.56284415653841791, 47.04930799450051637 ) ) ;
#11030=CARTESIAN_POINT ( 'NONE',  ( 8.698509210239564027, 29.59164230456639899, 47.04930799450051637 ) ) ;
#11031=AXIS2_PLACEMENT_3D ( 'NONE', #27369, #26878, #4391 ) ;
#11032=TOROIDAL_SURFACE ( 'NONE', #9974, 12.61792373059894601, 0.1249999999999988065 ) ;
#11033=DIRECTION ( 'NONE',  ( -1.101824276508909887E-16, 1.000000000000000000, -0.000000000000000000 ) ) ;
#11034=ORIENTED_EDGE ( 'NONE', *, *, #19704, .F. ) ;
#11038=EDGE_LOOP ( 'NONE', ( #25315, #20747, #13087, #213 ) ) ;
#11039=FACE_OUTER_BOUND ( 'NONE', #28908, .T. ) ;
#11040=CIRCLE ( 'NONE', #18347, 12.27641737965287838 ) ;
#11048=CARTESIAN_POINT ( 'NONE',  ( 33.72499318558949000, 38.56284415653841791, 47.04930799450051637 ) ) ;
#11049=EDGE_CURVE ( 'NONE', #14608, #12345, #28326, .T. ) ;
#11054=ADVANCED_FACE ( 'NONE', ( #19275 ), #14714, .T. ) ;
#11057=DIRECTION ( 'NONE',  ( -1.000000000000000000, 0.000000000000000000, 0.000000000000000000 ) ) ;
#11059=DIRECTION ( 'NONE',  ( 1.000000000000000000, 0.000000000000000000, 0.000000000000000000 ) ) ;
#11063=CARTESIAN_POINT ( 'NONE',  ( 8.482002859293391595, 23.71664230456639899, 47.04930799450051637 ) ) ;
#11068=CARTESIAN_POINT ( 'NONE',  ( 33.72499318558949710, 31.34184655352422766, 47.04930799450051637 ) ) ;
#11079=LINE ( 'NONE', #1369, #32494 ) ;
#11080=DIRECTION ( 'NONE',  ( -1.000000000000000000, 0.000000000000000000, 0.000000000000000000 ) ) ;
#11086=ORIENTED_EDGE ( 'NONE', *, *, #4202, .T. ) ;
#11087=ADVANCED_FACE ( 'NONE', ( #11905 ), #5808, .T. ) ;
#11088=VECTOR ( 'NONE', #19438, 1000.000000000000000 ) ;
#11091=EDGE_CURVE ( 'NONE', #20897, #22868, #25725, .T. ) ;
#11093=AXIS2_PLACEMENT_3D ( 'NONE', #17425, #25309, #27446 ) ;
#11096=CARTESIAN_POINT ( 'NONE',  ( 21.09992658989239089, 27.84164230456639544, 47.04930799450051637 ) ) ;
#11097=DIRECTION ( 'NONE',  ( -1.000000000000000000, -1.101824276508909887E-16, 0.000000000000000000 ) ) ;
#11099=VERTEX_POINT ( 'NONE', #31386 ) ;
#11103=AXIS2_PLACEMENT_3D ( 'NONE', #28662, #926, #3059 ) ;
#11107=DIRECTION ( 'NONE',  ( -1.101824276508909887E-16, 1.000000000000000000, -0.000000000000000000 ) ) ;
#11108=ORIENTED_EDGE ( 'NONE', *, *, #21432, .F. ) ;
#11110=FACE_OUTER_BOUND ( 'NONE', #25376, .T. ) ;
#11118=CARTESIAN_POINT ( 'NONE',  ( 33.46699938050303302, 38.56284415653841791, 47.04930799450051637 ) ) ;
#11120=ORIENTED_EDGE ( 'NONE', *, *, #12358, .F. ) ;
#11123=DIRECTION ( 'NONE',  ( -1.101824276508909887E-16, 1.000000000000000000, -0.000000000000000000 ) ) ;
#11125=ORIENTED_EDGE ( 'NONE', *, *, #3172, .F. ) ;
#11127=CIRCLE ( 'NONE', #6916, 0.1249999999999983763 ) ;
#11136=ORIENTED_EDGE ( 'NONE', *, *, #11565, .T. ) ;
#11137=TOROIDAL_SURFACE ( 'NONE', #20566, 12.61792373059895667, 0.1249999999999982098 ) ;
#11139=DIRECTION ( 'NONE',  ( -1.000000000000000000, -1.101824276508909764E-16, 0.000000000000000000 ) ) ;
#11155=DIRECTION ( 'NONE',  ( -1.101824276508909887E-16, 1.000000000000000000, -0.000000000000000000 ) ) ;
#11156=FACE_OUTER_BOUND ( 'NONE', #24348, .T. ) ;
#11161=DIRECTION ( 'NONE',  ( -1.101824276508909887E-16, 1.000000000000000000, -0.000000000000000000 ) ) ;
#11164=CIRCLE ( 'NONE', #29505, 12.62506659569710266 ) ;
#11167=EDGE_CURVE ( 'NONE', #11099, #26330, #27808, .T. ) ;
#11169=ORIENTED_EDGE ( 'NONE', *, *, #519, .T. ) ;
#11177=ORIENTED_EDGE ( 'NONE', *, *, #8746, .T. ) ;
#11179=ORIENTED_EDGE ( 'NONE', *, *, #30945, .T. ) ;
#11184=CIRCLE ( 'NONE', #15373, 0.1249999999999966416 ) ;
#11185=ORIENTED_EDGE ( 'NONE', *, *, #15240, .F. ) ;
#11188=FACE_OUTER_BOUND ( 'NONE', #11726, .T. ) ;
#11190=ORIENTED_EDGE ( 'NONE', *, *, #17068, .F. ) ;
#11197=EDGE_CURVE ( 'NONE', #9081, #10697, #26740, .T. ) ;
#11198=EDGE_CURVE ( 'NONE', #19299, #9250, #13662, .T. ) ;
#11201=CIRCLE ( 'NONE', #5425, 0.1250000000000001110 ) ;
#11207=AXIS2_PLACEMENT_3D ( 'NONE', #22889, #27502, #25362 ) ;
#11210=FACE_OUTER_BOUND ( 'NONE', #17218, .T. ) ;
#11217=DIRECTION ( 'NONE',  ( -1.000000000000000000, 0.000000000000000000, 0.000000000000000000 ) ) ;
#11219=FACE_OUTER_BOUND ( 'NONE', #13766, .T. ) ;
#11225=CIRCLE ( 'NONE', #26939, 12.62506659569710443 ) ;
#11227=DIRECTION ( 'NONE',  ( -1.101824276508909887E-16, 1.000000000000000000, -0.000000000000000000 ) ) ;
#11228=DIRECTION ( 'NONE',  ( -1.000000000000000000, 0.000000000000000000, 0.000000000000000000 ) ) ;
#11230=ORIENTED_EDGE ( 'NONE', *, *, #28933, .T. ) ;
#11243=EDGE_CURVE ( 'NONE', #2021, #22668, #6312, .T. ) ;
#11248=DIRECTION ( 'NONE',  ( -1.000000000000000000, 0.000000000000000000, 0.000000000000000000 ) ) ;
#11249=AXIS2_PLACEMENT_3D ( 'NONE', #602, #24902, #18944 ) ;
#11250=AXIS2_PLACEMENT_3D ( 'NONE', #25127, #1981, #4941 ) ;
#11254=AXIS2_PLACEMENT_3D ( 'NONE', #20522, #338, #20353 ) ;
#11255=DIRECTION ( 'NONE',  ( -1.000000000000000000, -1.101824276508909887E-16, 0.000000000000000000 ) ) ;
#11256=DIRECTION ( 'NONE',  ( 0.000000000000000000, -0.000000000000000000, -1.000000000000000000 ) ) ;
#11257=EDGE_CURVE ( 'NONE', #3723, #3559, #11040, .T. ) ;
#11266=EDGE_CURVE ( 'NONE', #30099, #16025, #4210, .T. ) ;
#11267=CARTESIAN_POINT ( 'NONE',  ( 33.50134396954521065, 29.84164230456639899, 47.04930799450051637 ) ) ;
#11269=FACE_OUTER_BOUND ( 'NONE', #12536, .T. ) ;
#11274=CARTESIAN_POINT ( 'NONE',  ( 8.732853799281738105, 25.46183152705960140, 47.04930799450051637 ) ) ;
#11276=FACE_OUTER_BOUND ( 'NONE', #5282, .T. ) ;
#11283=AXIS2_PLACEMENT_3D ( 'NONE', #25414, #24933, #25094 ) ;
#11287=ORIENTED_EDGE ( 'NONE', *, *, #29250, .F. ) ;
#11291=CARTESIAN_POINT ( 'NONE',  ( 21.09992658989239089, 24.34164230456639544, 47.04930799450051637 ) ) ;
#11295=ORIENTED_EDGE ( 'NONE', *, *, #15240, .T. ) ;
#11296=EDGE_LOOP ( 'NONE', ( #14898, #7884, #7875, #15270 ) ) ;
#11298=CARTESIAN_POINT ( 'NONE',  ( 8.474859994195286461, 26.84143805560860940, 47.04930799450051637 ) ) ;
#11302=AXIS2_PLACEMENT_3D ( 'NONE', #12887, #32253, #22545 ) ;
#11314=DIRECTION ( 'NONE',  ( -1.101824276508909887E-16, 1.000000000000000000, -0.000000000000000000 ) ) ;
#11315=EDGE_CURVE ( 'NONE', #27701, #21385, #9463, .T. ) ;
#11318=EDGE_LOOP ( 'NONE', ( #14954, #5911, #22965, #9369 ) ) ;
#11320=DIRECTION ( 'NONE',  ( -1.101824276508909887E-16, 1.000000000000000000, -0.000000000000000000 ) ) ;
#11322=CIRCLE ( 'NONE', #20241, 12.27641737965283930 ) ;
#11327=DIRECTION ( 'NONE',  ( -1.101824276508909887E-16, 1.000000000000000000, -0.000000000000000000 ) ) ;
#11328=CIRCLE ( 'NONE', #29685, 12.36707279061065101 ) ;
#11336=DIRECTION ( 'NONE',  ( -1.101824276508909887E-16, 1.000000000000000000, -0.000000000000000000 ) ) ;
#11340=ORIENTED_EDGE ( 'NONE', *, *, #9459, .F. ) ;
#11345=DIRECTION ( 'NONE',  ( -1.000000000000000000, -1.101824276508909887E-16, 0.000000000000000000 ) ) ;
#11346=ADVANCED_FACE ( 'NONE', ( #32127 ), #19424, .T. ) ;
#11349=ADVANCED_FACE ( 'NONE', ( #29663 ), #27184, .T. ) ;
#11352=EDGE_CURVE ( 'NONE', #1319, #9226, #30981, .T. ) ;
#11354=AXIS2_PLACEMENT_3D ( 'NONE', #30041, #27731, #11986 ) ;
#11358=FACE_OUTER_BOUND ( 'NONE', #18451, .T. ) ;
#11364=CARTESIAN_POINT ( 'NONE',  ( 8.698509210239501854, 23.59164230456639544, 47.04930799450051637 ) ) ;
#11365=EDGE_CURVE ( 'NONE', #63, #16672, #14195, .T. ) ;
#11370=DIRECTION ( 'NONE',  ( -1.000000000000000000, 0.000000000000000000, 0.000000000000000000 ) ) ;
#11373=ORIENTED_EDGE ( 'NONE', *, *, #19838, .F. ) ;
#11377=CYLINDRICAL_SURFACE ( 'NONE', #9298, 12.36707279061065101 ) ;
#11378=CYLINDRICAL_SURFACE ( 'NONE', #25232, 12.62506659569710266 ) ;
#11380=ORIENTED_EDGE ( 'NONE', *, *, #15759, .F. ) ;
#11392=EDGE_LOOP ( 'NONE', ( #403, #15879, #9787, #767 ) ) ;
#11394=EDGE_CURVE ( 'NONE', #29823, #29193, #12632, .T. ) ;
#11396=CARTESIAN_POINT ( 'NONE',  ( 21.09992658989238734, 31.47145308207317171, 47.04930799450051637 ) ) ;
#11400=AXIS2_PLACEMENT_3D ( 'NONE', #20828, #3097, #18834 ) ;
#11403=ORIENTED_EDGE ( 'NONE', *, *, #13989, .F. ) ;
#11406=AXIS2_PLACEMENT_3D ( 'NONE', #968, #30408, #29929 ) ;
#11410=DIRECTION ( 'NONE',  ( -1.101824276508909887E-16, 1.000000000000000000, -0.000000000000000000 ) ) ;
#11414=FACE_OUTER_BOUND ( 'NONE', #10766, .T. ) ;
#11415=CARTESIAN_POINT ( 'NONE',  ( 21.09992658989238734, 31.97145308207317171, 47.04930799450051637 ) ) ;
#11416=AXIS2_PLACEMENT_3D ( 'NONE', #21393, #3202, #1068 ) ;
#11424=DIRECTION ( 'NONE',  ( -1.000000000000000000, 0.000000000000000000, 0.000000000000000000 ) ) ;
#11425=DIRECTION ( 'NONE',  ( -1.000000000000000000, 0.000000000000000000, 0.000000000000000000 ) ) ;
#11428=AXIS2_PLACEMENT_3D ( 'NONE', #31337, #15855, #6158 ) ;
#11432=AXIS2_PLACEMENT_3D ( 'NONE', #25319, #31330, #11462 ) ;
#11433=EDGE_CURVE ( 'NONE', #28828, #23509, #23558, .T. ) ;
#11435=AXIS2_PLACEMENT_3D ( 'NONE', #4623, #26461, #26619 ) ;
#11439=CARTESIAN_POINT ( 'NONE',  ( 8.732853799281734553, 38.56284415653841791, 47.04930799450051637 ) ) ;
#11440=EDGE_CURVE ( 'NONE', #3369, #28743, #18304, .T. ) ;
#11445=ORIENTED_EDGE ( 'NONE', *, *, #1580, .F. ) ;
#11446=ORIENTED_EDGE ( 'NONE', *, *, #19881, .T. ) ;
#11450=CARTESIAN_POINT ( 'NONE',  ( 33.72499318558949710, 25.34184655352419213, 47.04930799450051637 ) ) ;
#11451=AXIS2_PLACEMENT_3D ( 'NONE', #13311, #11320, #13947 ) ;
#11454=DIRECTION ( 'NONE',  ( -1.000000000000000000, 0.000000000000000000, 0.000000000000000000 ) ) ;
#11457=CIRCLE ( 'NONE', #29818, 12.27641737965287660 ) ;
#11459=LINE ( 'NONE', #28224, #3312 ) ;
#11460=ORIENTED_EDGE ( 'NONE', *, *, #2072, .F. ) ;
#11461=DIRECTION ( 'NONE',  ( -1.000000000000000000, 0.000000000000000000, 0.000000000000000000 ) ) ;
#11462=DIRECTION ( 'NONE',  ( -1.000000000000000000, 0.000000000000000000, 0.000000000000000000 ) ) ;
#11466=FACE_OUTER_BOUND ( 'NONE', #23941, .T. ) ;
#11468=CARTESIAN_POINT ( 'NONE',  ( 21.09992658989239089, 26.09143805560860940, 47.04930799450051637 ) ) ;
#11470=CARTESIAN_POINT ( 'NONE',  ( 8.698509210239542710, 27.59164230456639544, 47.04930799450051637 ) ) ;
#11471=DIRECTION ( 'NONE',  ( -1.000000000000000000, 0.000000000000000000, 0.000000000000000000 ) ) ;
#11472=ORIENTED_EDGE ( 'NONE', *, *, #6435, .F. ) ;
#11474=AXIS2_PLACEMENT_3D ( 'NONE', #30350, #5239, #25418 ) ;
#11475=CIRCLE ( 'NONE', #20917, 0.1250000000000001110 ) ;
#11480=DIRECTION ( 'NONE',  ( -1.224646799147353207E-16, -1.349345573449484691E-32, 1.000000000000000000 ) ) ;
#11481=EDGE_CURVE ( 'NONE', #27575, #17665, #10000, .T. ) ;
#11482=AXIS2_PLACEMENT_3D ( 'NONE', #5742, #25117, #12976 ) ;
#11484=DIRECTION ( 'NONE',  ( -1.101824276508909887E-16, 1.000000000000000000, -0.000000000000000000 ) ) ;
#11485=AXIS2_PLACEMENT_3D ( 'NONE', #9373, #24795, #14141 ) ;
#11486=DIRECTION ( 'NONE',  ( -1.000000000000000000, -1.101824276508909887E-16, 0.000000000000000000 ) ) ;
#11488=ORIENTED_EDGE ( 'NONE', *, *, #5988, .T. ) ;
#11489=DIRECTION ( 'NONE',  ( -1.101824276508909887E-16, 1.000000000000000000, -0.000000000000000000 ) ) ;
#11493=DIRECTION ( 'NONE',  ( -1.000000000000000000, 0.000000000000000000, 0.000000000000000000 ) ) ;
#11495=EDGE_LOOP ( 'NONE', ( #6735, #30385, #6253, #17592 ) ) ;
#11496=ORIENTED_EDGE ( 'NONE', *, *, #31432, .F. ) ;
#11499=DIRECTION ( 'NONE',  ( -1.101824276508909887E-16, 1.000000000000000000, -0.000000000000000000 ) ) ;
#11502=ORIENTED_EDGE ( 'NONE', *, *, #19280, .T. ) ;
#11505=VERTEX_POINT ( 'NONE', #30482 ) ;
#11508=CIRCLE ( 'NONE', #27222, 0.1250000000000001110 ) ;
#11509=AXIS2_PLACEMENT_3D ( 'NONE', #10917, #7976, #3186 ) ;
#11510=DIRECTION ( 'NONE',  ( -1.101824276508909887E-16, 1.000000000000000000, -0.000000000000000000 ) ) ;
#11511=AXIS2_PLACEMENT_3D ( 'NONE', #25407, #295, #20477 ) ;
#11513=ORIENTED_EDGE ( 'NONE', *, *, #31859, .T. ) ;
#11514=CARTESIAN_POINT ( 'NONE',  ( 21.09992658989239089, 28.34164230456639544, 47.04930799450051637 ) ) ;
#11519=AXIS2_PLACEMENT_3D ( 'NONE', #23360, #23683, #5969 ) ;
#11520=ADVANCED_FACE ( 'NONE', ( #17827 ), #25864, .F. ) ;
#11523=EDGE_CURVE ( 'NONE', #14337, #8103, #22048, .T. ) ;
#11526=CARTESIAN_POINT ( 'NONE',  ( 21.09992658989238734, 38.56284415653841791, 47.04930799450051637 ) ) ;
#11528=CARTESIAN_POINT ( 'NONE',  ( 21.09992658989239089, 29.34143805560861296, 47.04930799450051637 ) ) ;
#11535=CARTESIAN_POINT ( 'NONE',  ( 21.09992658989238734, 31.21183152705961206, 47.04930799450051637 ) ) ;
#11536=AXIS2_PLACEMENT_3D ( 'NONE', #19642, #17518, #27534 ) ;
#11541=FACE_OUTER_BOUND ( 'NONE', #7031, .T. ) ;
#11542=CARTESIAN_POINT ( 'NONE',  ( 8.732853799281729223, 30.72145308207317882, 47.04930799450051637 ) ) ;
#11547=CYLINDRICAL_SURFACE ( 'NONE', #25876, 12.36707279061065101 ) ;
#11552=AXIS2_PLACEMENT_3D ( 'NONE', #11864, #23687, #28608 ) ;
#11564=EDGE_CURVE ( 'NONE', #30197, #20645, #27311, .T. ) ;
#11565=EDGE_CURVE ( 'NONE', #12497, #30197, #5296, .T. ) ;
#11566=EDGE_CURVE ( 'NONE', #23085, #7282, #23630, .T. ) ;
#11569=DIRECTION ( 'NONE',  ( -1.000000000000000000, 0.000000000000000000, 0.000000000000000000 ) ) ;
#11573=AXIS2_PLACEMENT_3D ( 'NONE', #14900, #22425, #20135 ) ;
#11574=EDGE_LOOP ( 'NONE', ( #21870, #31828, #30935, #9029 ) ) ;
#11576=ORIENTED_EDGE ( 'NONE', *, *, #17408, .T. ) ;
#11578=ORIENTED_EDGE ( 'NONE', *, *, #19556, .F. ) ;
#11580=CARTESIAN_POINT ( 'NONE',  ( 21.09992658989239089, 25.84164230456639899, 47.04930799450051637 ) ) ;
#11581=LINE ( 'NONE', #22348, #18611 ) ;
#11585=DIRECTION ( 'NONE',  ( -1.101824276508909887E-16, 1.000000000000000000, -0.000000000000000000 ) ) ;
#11588=DIRECTION ( 'NONE',  ( -1.000000000000000000, -1.101824276508910010E-16, 0.000000000000000000 ) ) ;
#11592=LINE ( 'NONE', #31615, #32186 ) ;
#11597=CARTESIAN_POINT ( 'NONE',  ( 21.09992658989239089, 23.97145308207319658, 47.04930799450051637 ) ) ;
#11605=CIRCLE ( 'NONE', #26817, 12.36707279061065101 ) ;
#11609=ORIENTED_EDGE ( 'NONE', *, *, #22476, .T. ) ;
#11610=DIRECTION ( 'NONE',  ( -1.101824276508909887E-16, 1.000000000000000000, -0.000000000000000000 ) ) ;
#11615=ORIENTED_EDGE ( 'NONE', *, *, #24557, .F. ) ;
#11618=CARTESIAN_POINT ( 'NONE',  ( 33.46699938050303302, 38.56284415653841791, 47.04930799450051637 ) ) ;
#11619=CIRCLE ( 'NONE', #16316, 0.1249999999999983763 ) ;
#11620=ORIENTED_EDGE ( 'NONE', *, *, #6304, .T. ) ;
#11629=EDGE_CURVE ( 'NONE', #16953, #27014, #1391, .T. ) ;
#11634=EDGE_CURVE ( 'NONE', #21015, #16985, #13172, .T. ) ;
#11645=FACE_OUTER_BOUND ( 'NONE', #22262, .T. ) ;
#11658=TOROIDAL_SURFACE ( 'NONE', #2761, 12.61792373059897265, 0.1249999999999971551 ) ;
#11665=DIRECTION ( 'NONE',  ( -1.000000000000000000, 0.000000000000000000, 0.000000000000000000 ) ) ;
#11669=VERTEX_POINT ( 'NONE', #31279 ) ;
#11675=AXIS2_PLACEMENT_3D ( 'NONE', #25783, #679, #5933 ) ;
#11678=LINE ( 'NONE', #16265, #24082 ) ;
#11685=EDGE_CURVE ( 'NONE', #19299, #22139, #580, .T. ) ;
#11686=CIRCLE ( 'NONE', #26365, 12.62506659569710266 ) ;
#11688=MANIFOLD_SOLID_BREP ( 'Stock-MAT-060-1', #3216 ) ;
#11693=ORIENTED_EDGE ( 'NONE', *, *, #26223, .F. ) ;
#11699=DIRECTION ( 'NONE',  ( -1.224646799147353207E-16, -1.349345573449484691E-32, 1.000000000000000000 ) ) ;
#11700=LINE ( 'NONE', #23557, #1680 ) ;
#11702=DIRECTION ( 'NONE',  ( -1.000000000000000000, 0.000000000000000000, 0.000000000000000000 ) ) ;
#11703=TOROIDAL_SURFACE ( 'NONE', #16424, 12.40141737965279667, 0.1249999999999991951 ) ;
#11706=ORIENTED_EDGE ( 'NONE', *, *, #19702, .T. ) ;
#11707=DIRECTION ( 'NONE',  ( -1.000000000000000000, 0.000000000000000000, 0.000000000000000000 ) ) ;
#11709=DIRECTION ( 'NONE',  ( -1.101824276508909887E-16, 1.000000000000000000, -0.000000000000000000 ) ) ;
#11715=EDGE_LOOP ( 'NONE', ( #25334, #17328, #28575, #12056 ) ) ;
#11716=DIRECTION ( 'NONE',  ( -1.000000000000000000, 0.000000000000000000, 0.000000000000000000 ) ) ;
#11718=CARTESIAN_POINT ( 'NONE',  ( 33.71785032049097453, 31.46664230456641675, 47.04930799450051637 ) ) ;
#11719=EDGE_CURVE ( 'NONE', #7469, #21385, #29973, .T. ) ;
#11723=EDGE_LOOP ( 'NONE', ( #29078, #2600, #4870, #12100 ) ) ;
#11724=CIRCLE ( 'NONE', #17483, 12.36707279061065101 ) ;
#11726=EDGE_LOOP ( 'NONE', ( #11028, #9211, #6832, #16968 ) ) ;
#11732=DIRECTION ( 'NONE',  ( -1.000000000000000000, 0.000000000000000000, 0.000000000000000000 ) ) ;
#11734=ORIENTED_EDGE ( 'NONE', *, *, #20888, .F. ) ;
#11736=ORIENTED_EDGE ( 'NONE', *, *, #5837, .T. ) ;
#11738=( LENGTH_UNIT ( ) NAMED_UNIT ( * ) SI_UNIT ( .MILLI., .METRE. ) );
#11742=DIRECTION ( 'NONE',  ( -1.000000000000000000, 0.000000000000000000, 0.000000000000000000 ) ) ;
#11744=DIRECTION ( 'NONE',  ( -1.000000000000000000, 0.000000000000000000, 0.000000000000000000 ) ) ;
#11746=CARTESIAN_POINT ( 'NONE',  ( 21.09992658989239089, 23.84164230456639544, 47.04930799450051637 ) ) ;
#11748=AXIS2_PLACEMENT_3D ( 'NONE', #6987, #4362, #31457 ) ;
#11749=DIRECTION ( 'NONE',  ( -1.101824276508909887E-16, 1.000000000000000000, -0.000000000000000000 ) ) ;
#11750=EDGE_LOOP ( 'NONE', ( #21315, #27379, #30571, #13237 ) ) ;
#11752=DIRECTION ( 'NONE',  ( 0.000000000000000000, -0.000000000000000000, -1.000000000000000000 ) ) ;
#11753=VERTEX_POINT ( 'NONE', #17131 ) ;
#11755=DIRECTION ( 'NONE',  ( -1.101824276508909887E-16, 1.000000000000000000, -0.000000000000000000 ) ) ;
#11772=DIRECTION ( 'NONE',  ( -1.000000000000000000, 0.000000000000000000, 0.000000000000000000 ) ) ;
#11777=ORIENTED_EDGE ( 'NONE', *, *, #8178, .T. ) ;
#11779=ORIENTED_EDGE ( 'NONE', *, *, #3551, .F. ) ;
#11781=EDGE_CURVE ( 'NONE', #29845, #23862, #9441, .T. ) ;
#11786=DIRECTION ( 'NONE',  ( -1.101824276508909887E-16, 1.000000000000000000, -0.000000000000000000 ) ) ;
#11789=TOROIDAL_SURFACE ( 'NONE', #14414, 12.61792373059896555, 0.1249999999999975853 ) ;
#11794=DIRECTION ( 'NONE',  ( -1.224646799147353207E-16, -1.349345573449484691E-32, 1.000000000000000000 ) ) ;
#11795=DIRECTION ( 'NONE',  ( -1.224646799147353207E-16, -1.349345573449484691E-32, 1.000000000000000000 ) ) ;
#11797=DIRECTION ( 'NONE',  ( 0.000000000000000000, -0.000000000000000000, -1.000000000000000000 ) ) ;
#11798=AXIS2_PLACEMENT_3D ( 'NONE', #20131, #27188, #32456 ) ;
#11802=ORIENTED_EDGE ( 'NONE', *, *, #590, .T. ) ;
#11803=CARTESIAN_POINT ( 'NONE',  ( 33.37634396954528171, 23.59164230456639544, 47.04930799450051637 ) ) ;
#11806=DIRECTION ( 'NONE',  ( -1.101824276508909887E-16, 1.000000000000000000, -0.000000000000000000 ) ) ;
#11809=TOROIDAL_SURFACE ( 'NONE', #31215, 12.40141737965286595, 0.1249999999999979183 ) ;
#11810=VERTEX_POINT ( 'NONE', #32417 ) ;
#11812=CIRCLE ( 'NONE', #14438, 12.62506659569710443 ) ;
#11813=LINE ( 'NONE', #21646, #1306 ) ;
#11818=ADVANCED_FACE ( 'NONE', ( #14527 ), #4673, .F. ) ;
#11819=CIRCLE ( 'NONE', #23349, 0.1250000000000018319 ) ;
#11828=ORIENTED_EDGE ( 'NONE', *, *, #19045, .F. ) ;
#11836=DIRECTION ( 'NONE',  ( -1.000000000000000000, 0.000000000000000000, 0.000000000000000000 ) ) ;
#11837=VERTEX_POINT ( 'NONE', #14857 ) ;
#11840=ORIENTED_EDGE ( 'NONE', *, *, #10502, .T. ) ;
#11843=ADVANCED_FACE ( 'NONE', ( #29959 ), #2168, .T. ) ;
#11848=ADVANCED_FACE ( 'NONE', ( #24861 ), #14757, .T. ) ;
#11852=EDGE_CURVE ( 'NONE', #28587, #7860, #8273, .T. ) ;
#11856=CIRCLE ( 'NONE', #10817, 12.62506659569710266 ) ;
#11858=STYLED_ITEM ( 'NONE', ( #13649 ), #12811 ) ;
#11864=CARTESIAN_POINT ( 'NONE',  ( 21.09992658989238734, 38.56284415653841791, 47.04930799450051637 ) ) ;
#11865=ORIENTED_EDGE ( 'NONE', *, *, #17828, .T. ) ;
#11866=DIRECTION ( 'NONE',  ( -1.000000000000000000, -1.101824276508909887E-16, 0.000000000000000000 ) ) ;
#11867=DIRECTION ( 'NONE',  ( -1.101824276508909887E-16, 1.000000000000000000, -0.000000000000000000 ) ) ;
#11868=TOROIDAL_SURFACE ( 'NONE', #16055, 12.40141737965281976, 0.1249999999999999722 ) ;
#11869=CARTESIAN_POINT ( 'NONE',  ( 21.09992658989239089, 29.59184655352418858, 47.04930799450051637 ) ) ;
#11871=DIRECTION ( 'NONE',  ( -1.101824276508909887E-16, 1.000000000000000000, -0.000000000000000000 ) ) ;
#11873=DIRECTION ( 'NONE',  ( -1.000000000000000000, -1.101824276508909887E-16, 0.000000000000000000 ) ) ;
#11875=ORIENTED_EDGE ( 'NONE', *, *, #714, .T. ) ;
#11876=CARTESIAN_POINT ( 'NONE',  ( 21.09992658989239089, 30.59164230456639544, 47.04930799450051637 ) ) ;
#11877=DIRECTION ( 'NONE',  ( 1.000000000000000000, 0.000000000000000000, 0.000000000000000000 ) ) ;
#11879=DIRECTION ( 'NONE',  ( -1.101824276508909887E-16, 1.000000000000000000, -0.000000000000000000 ) ) ;
#11883=CIRCLE ( 'NONE', #25522, 12.62506659569710443 ) ;
#11886=EDGE_CURVE ( 'NONE', #25156, #3119, #28140, .T. ) ;
#11887=CIRCLE ( 'NONE', #8737, 0.1250000000000001110 ) ;
#11889=CARTESIAN_POINT ( 'NONE',  ( 21.09992658989239089, 24.59184655352419213, 47.04930799450051637 ) ) ;
#11891=CARTESIAN_POINT ( 'NONE',  ( 21.09992658989238734, 32.59164230456639899, 47.04930799450051637 ) ) ;
#11900=EDGE_LOOP ( 'NONE', ( #26229, #25009, #11179, #16857 ) ) ;
#11905=FACE_OUTER_BOUND ( 'NONE', #26225, .T. ) ;
#11906=CARTESIAN_POINT ( 'NONE',  ( 21.09992658989238734, 32.09143805560860585, 47.04930799450051637 ) ) ;
#11910=VERTEX_POINT ( 'NONE', #25508 ) ;
#11911=CARTESIAN_POINT ( 'NONE',  ( 21.09992658989239089, 25.34164230456639899, 47.04930799450051637 ) ) ;
#11912=DIRECTION ( 'NONE',  ( -1.000000000000000000, -1.101824276508909764E-16, 0.000000000000000000 ) ) ;
#11914=ORIENTED_EDGE ( 'NONE', *, *, #22197, .T. ) ;
#11916=AXIS2_PLACEMENT_3D ( 'NONE', #22500, #31, #17584 ) ;
#11917=ORIENTED_EDGE ( 'NONE', *, *, #7950, .T. ) ;
#11918=AXIS2_PLACEMENT_3D ( 'NONE', #19211, #6598, #29238 ) ;
#11923=ADVANCED_FACE ( 'NONE', ( #10586 ), #25982, .F. ) ;
#11926=LINE ( 'NONE', #18255, #4293 ) ;
#11935=ORIENTED_EDGE ( 'NONE', *, *, #23234, .T. ) ;
#11937=EDGE_CURVE ( 'NONE', #9226, #32103, #20579, .T. ) ;
#11938=VERTEX_POINT ( 'NONE', #5816 ) ;
#11944=CARTESIAN_POINT ( 'NONE',  ( 33.72499318558949710, 30.34143805560860585, 47.04930799450051637 ) ) ;
#11951=FACE_OUTER_BOUND ( 'NONE', #28446, .T. ) ;
#11954=AXIS2_PLACEMENT_3D ( 'NONE', #10929, #20608, #30956 ) ;
#11959=AXIS2_PLACEMENT_3D ( 'NONE', #27047, #14910, #20143 ) ;
#11961=CYLINDRICAL_SURFACE ( 'NONE', #23549, 12.36707279061065279 ) ;
#11964=ORIENTED_EDGE ( 'NONE', *, *, #3227, .T. ) ;
#11968=DIRECTION ( 'NONE',  ( -1.000000000000000000, 0.000000000000000000, 0.000000000000000000 ) ) ;
#11972=ORIENTED_EDGE ( 'NONE', *, *, #4133, .T. ) ;
#11974=ADVANCED_FACE ( 'NONE', ( #21359 ), #30995, .T. ) ;
#11978=CARTESIAN_POINT ( 'NONE',  ( 8.474859994195286461, 30.34143805560860585, 47.04930799450051637 ) ) ;
#11979=CYLINDRICAL_SURFACE ( 'NONE', #28449, 12.62506659569710266 ) ;
#11980=EDGE_CURVE ( 'NONE', #20581, #16953, #3214, .T. ) ;
#11986=DIRECTION ( 'NONE',  ( -1.000000000000000000, 0.000000000000000000, 0.000000000000000000 ) ) ;
#11987=CARTESIAN_POINT ( 'NONE',  ( 21.09992658989238734, 38.56284415653841791, 47.04930799450051637 ) ) ;
#11988=DIRECTION ( 'NONE',  ( -1.000000000000000000, 0.000000000000000000, 0.000000000000000000 ) ) ;
#11991=VERTEX_POINT ( 'NONE', #28611 ) ;
#12001=CARTESIAN_POINT ( 'NONE',  ( 21.09992658989238734, 38.56284415653841791, 47.04930799450051637 ) ) ;
#12003=AXIS2_PLACEMENT_3D ( 'NONE', #12214, #31905, #22368 ) ;
#12012=VERTEX_POINT ( 'NONE', #9073 ) ;
#12017=AXIS2_PLACEMENT_3D ( 'NONE', #28170, #5683, #25705 ) ;
#12020=DIRECTION ( 'NONE',  ( -1.000000000000000000, 0.000000000000000000, 0.000000000000000000 ) ) ;
#12021=DIRECTION ( 'NONE',  ( -1.101824276508909887E-16, 1.000000000000000000, -0.000000000000000000 ) ) ;
#12023=FACE_OUTER_BOUND ( 'NONE', #26750, .T. ) ;
#12025=ORIENTED_EDGE ( 'NONE', *, *, #27201, .T. ) ;
#12026=FACE_OUTER_BOUND ( 'NONE', #28847, .T. ) ;
#12028=DIRECTION ( 'NONE',  ( -1.000000000000000000, 0.000000000000000000, 0.000000000000000000 ) ) ;
#12032=DIRECTION ( 'NONE',  ( 0.000000000000000000, -0.000000000000000000, -1.000000000000000000 ) ) ;
#12033=CIRCLE ( 'NONE', #2609, 12.62506659569710266 ) ;
#12035=CARTESIAN_POINT ( 'NONE',  ( 21.09992658989238734, 38.56284415653841791, 47.04930799450051637 ) ) ;
#12038=ORIENTED_EDGE ( 'NONE', *, *, #5434, .T. ) ;
#12049=ADVANCED_FACE ( 'NONE', ( #13843 ), #18927, .T. ) ;
#12050=VECTOR ( 'NONE', #22328, 1000.000000000000000 ) ;
#12051=EDGE_LOOP ( 'NONE', ( #13370, #8274, #32378, #8944 ) ) ;
#12053=FACE_OUTER_BOUND ( 'NONE', #28839, .T. ) ;
#12055=AXIS2_PLACEMENT_3D ( 'NONE', #24843, #17448, #22366 ) ;
#12056=ORIENTED_EDGE ( 'NONE', *, *, #11564, .F. ) ;
#12065=ORIENTED_EDGE ( 'NONE', *, *, #590, .F. ) ;
#12066=DIRECTION ( 'NONE',  ( -1.101824276508909887E-16, 1.000000000000000000, -0.000000000000000000 ) ) ;
#12067=DIRECTION ( 'NONE',  ( -1.101824276508909887E-16, 1.000000000000000000, -0.000000000000000000 ) ) ;
#12068=CARTESIAN_POINT ( 'NONE',  ( 21.09992658989239089, 24.72145308207319303, 47.04930799450051637 ) ) ;
#12070=CARTESIAN_POINT ( 'NONE',  ( 21.09992658989239089, 29.34164230456639899, 47.04930799450051637 ) ) ;
#12071=DIRECTION ( 'NONE',  ( 0.000000000000000000, -0.000000000000000000, -1.000000000000000000 ) ) ;
#12078=VERTEX_POINT ( 'NONE', #4800 ) ;
#12081=EDGE_CURVE ( 'NONE', #31932, #17073, #16935, .T. ) ;
#12089=AXIS2_PLACEMENT_3D ( 'NONE', #31167, #3266, #31009 ) ;
#12090=ORIENTED_EDGE ( 'NONE', *, *, #18520, .T. ) ;
#12096=TOROIDAL_SURFACE ( 'NONE', #14203, 12.40141737965281621, 0.1249999999999985428 ) ;
#12100=ORIENTED_EDGE ( 'NONE', *, *, #24470, .T. ) ;
#12102=DIRECTION ( 'NONE',  ( -1.101824276508909887E-16, 1.000000000000000000, -0.000000000000000000 ) ) ;
#12103=AXIS2_PLACEMENT_3D ( 'NONE', #31293, #8167, #28515 ) ;
#12105=DIRECTION ( 'NONE',  ( -1.101824276508909887E-16, 1.000000000000000000, -0.000000000000000000 ) ) ;
#12106=CIRCLE ( 'NONE', #2150, 0.1250000000000001110 ) ;
#12111=CARTESIAN_POINT ( 'NONE',  ( 33.46699938050304013, 28.97145308207318237, 47.04930799450050927 ) ) ;
#12119=DIRECTION ( 'NONE',  ( -1.101824276508909887E-16, 1.000000000000000000, -0.000000000000000000 ) ) ;
#12124=DIRECTION ( 'NONE',  ( 0.000000000000000000, -0.000000000000000000, -1.000000000000000000 ) ) ;
#12131=ORIENTED_EDGE ( 'NONE', *, *, #21747, .T. ) ;
#12134=ORIENTED_EDGE ( 'NONE', *, *, #11197, .T. ) ;
#12137=AXIS2_PLACEMENT_3D ( 'NONE', #18990, #29018, #16535 ) ;
#12138=AXIS2_PLACEMENT_3D ( 'NONE', #3699, #1553, #24041 ) ;
#12139=ORIENTED_EDGE ( 'NONE', *, *, #7820, .T. ) ;
#12142=VECTOR ( 'NONE', #17670, 1000.000000000000000 ) ;
#12146=CARTESIAN_POINT ( 'NONE',  ( 21.09992658989238734, 32.55121380581068991, 47.04930799450051637 ) ) ;
#12147=ORIENTED_EDGE ( 'NONE', *, *, #16340, .F. ) ;
#12149=FACE_OUTER_BOUND ( 'NONE', #21859, .T. ) ;
#12150=ORIENTED_EDGE ( 'NONE', *, *, #28461, .F. ) ;
#12151=DIRECTION ( 'NONE',  ( -1.101824276508909887E-16, 1.000000000000000000, -0.000000000000000000 ) ) ;
#12160=CARTESIAN_POINT ( 'NONE',  ( 21.09992658989238734, 31.59164230456639544, 47.04930799450051637 ) ) ;
#12165=DIRECTION ( 'NONE',  ( -1.101824276508909887E-16, 1.000000000000000000, -0.000000000000000000 ) ) ;
#12166=ORIENTED_EDGE ( 'NONE', *, *, #15718, .T. ) ;
#12173=ADVANCED_FACE ( 'NONE', ( #9887 ), #4633, .F. ) ;
#12179=DIRECTION ( 'NONE',  ( -1.000000000000000000, 0.000000000000000000, 0.000000000000000000 ) ) ;
#12187=DIRECTION ( 'NONE',  ( -1.101824276508909887E-16, 1.000000000000000000, -0.000000000000000000 ) ) ;
#12188=DIRECTION ( 'NONE',  ( -1.000000000000000000, 0.000000000000000000, 0.000000000000000000 ) ) ;
#12200=TOROIDAL_SURFACE ( 'NONE', #15881, 12.40141737965281621, 0.1249999999999985428 ) ;
#12202=CYLINDRICAL_SURFACE ( 'NONE', #27730, 12.36707279061065101 ) ;
#12204=CIRCLE ( 'NONE', #9594, 0.1249999999999966416 ) ;
#12214=CARTESIAN_POINT ( 'NONE',  ( 21.09992658989238734, 31.09164230456639544, 47.04930799450051637 ) ) ;
#12215=ORIENTED_EDGE ( 'NONE', *, *, #4903, .T. ) ;
#12218=CIRCLE ( 'NONE', #19531, 12.36707279061065101 ) ;
#12221=EDGE_LOOP ( 'NONE', ( #10317, #5682, #28362, #24549 ) ) ;
#12222=CIRCLE ( 'NONE', #26882, 0.1249999999999983763 ) ;
#12225=DIRECTION ( 'NONE',  ( -1.000000000000000000, 0.000000000000000000, 0.000000000000000000 ) ) ;
#12226=CARTESIAN_POINT ( 'NONE',  ( 33.46699938050304013, 24.97145308207319303, 47.04930799450050927 ) ) ;
#12229=DIRECTION ( 'NONE',  ( -1.000000000000000000, 0.000000000000000000, 0.000000000000000000 ) ) ;
#12231=DIRECTION ( 'NONE',  ( -1.101824276508909887E-16, 1.000000000000000000, -0.000000000000000000 ) ) ;
#12238=CARTESIAN_POINT ( 'NONE',  ( 8.698509210239539158, 27.34164230456639544, 47.04930799450051637 ) ) ;
#12240=DIRECTION ( 'NONE',  ( -1.101824276508909887E-16, 1.000000000000000000, -0.000000000000000000 ) ) ;
#12242=CIRCLE ( 'NONE', #29001, 12.62506659569710266 ) ;
#12245=DIRECTION ( 'NONE',  ( -1.000000000000000000, 0.000000000000000000, 0.000000000000000000 ) ) ;
#12249=DIRECTION ( 'NONE',  ( -1.101824276508909887E-16, 1.000000000000000000, -0.000000000000000000 ) ) ;
#12251=AXIS2_PLACEMENT_3D ( 'NONE', #30455, #25199, #10110 ) ;
#12253=CIRCLE ( 'NONE', #22711, 12.27641737965280555 ) ;
#12256=ORIENTED_EDGE ( 'NONE', *, *, #24446, .F. ) ;
#12263=ORIENTED_EDGE ( 'NONE', *, *, #27843, .F. ) ;
#12267=DIRECTION ( 'NONE',  ( -1.101824276508909887E-16, 1.000000000000000000, -0.000000000000000000 ) ) ;
#12269=CARTESIAN_POINT ( 'NONE',  ( 21.09992658989239089, 25.59184655352419213, 47.04930799450051637 ) ) ;
#12270=EDGE_LOOP ( 'NONE', ( #23823, #1502, #14657, #8541 ) ) ;
#12275=EDGE_CURVE ( 'NONE', #27738, #22606, #26773, .T. ) ;
#12277=DIRECTION ( 'NONE',  ( -1.000000000000000000, 0.000000000000000000, 0.000000000000000000 ) ) ;
#12281=DIRECTION ( 'NONE',  ( -1.000000000000000000, 0.000000000000000000, 0.000000000000000000 ) ) ;
#12287=CARTESIAN_POINT ( 'NONE',  ( 33.46699938050304013, 38.56284415653841791, 47.04930799450051637 ) ) ;
#12288=ORIENTED_EDGE ( 'NONE', *, *, #19979, .T. ) ;
#12289=CARTESIAN_POINT ( 'NONE',  ( 21.09992658989238734, 30.71664230456641675, 47.04930799450051637 ) ) ;
#12294=CIRCLE ( 'NONE', #30127, 12.36707279061065279 ) ;
#12295=AXIS2_PLACEMENT_3D ( 'NONE', #17414, #2647, #22664 ) ;
#12299=DIRECTION ( 'NONE',  ( -1.101824276508909887E-16, 1.000000000000000000, -0.000000000000000000 ) ) ;
#12300=VERTEX_POINT ( 'NONE', #10218 ) ;
#12301=CIRCLE ( 'NONE', #12856, 0.1250000000000001110 ) ;
#12303=CARTESIAN_POINT ( 'NONE',  ( 21.09992658989238734, 38.56284415653841791, 47.04930799450051637 ) ) ;
#12304=DIRECTION ( 'NONE',  ( -1.101824276508909887E-16, 1.000000000000000000, -0.000000000000000000 ) ) ;
#12309=AXIS2_PLACEMENT_3D ( 'NONE', #28176, #23080, #27684 ) ;
#12317=FACE_OUTER_BOUND ( 'NONE', #24784, .T. ) ;
#12323=EDGE_LOOP ( 'NONE', ( #19870, #26914, #8942, #24541 ) ) ;
#12324=DIRECTION ( 'NONE',  ( -1.000000000000000000, 0.000000000000000000, 0.000000000000000000 ) ) ;
#12325=DIRECTION ( 'NONE',  ( -1.000000000000000000, -1.101824276508909887E-16, 0.000000000000000000 ) ) ;
#12330=DIRECTION ( 'NONE',  ( -1.224646799147353207E-16, -1.349345573449484691E-32, 1.000000000000000000 ) ) ;
#12331=EDGE_LOOP ( 'NONE', ( #13309, #23660, #7072, #9843 ) ) ;
#12332=CYLINDRICAL_SURFACE ( 'NONE', #11485, 12.62506659569710266 ) ;
#12335=AXIS2_PLACEMENT_3D ( 'NONE', #14927, #7385, #21969 ) ;
#12341=VERTEX_POINT ( 'NONE', #13570 ) ;
#12345=VERTEX_POINT ( 'NONE', #924 ) ;
#12349=EDGE_CURVE ( 'NONE', #21924, #30824, #18884, .T. ) ;
#12350=CARTESIAN_POINT ( 'NONE',  ( 21.09992658989238734, 38.56284415653841791, 47.04930799450051637 ) ) ;
#12351=DIRECTION ( 'NONE',  ( -1.224646799147353207E-16, -1.349345573449484691E-32, 1.000000000000000000 ) ) ;
#12352=CARTESIAN_POINT ( 'NONE',  ( 33.37634396954523908, 27.59164230456639544, 47.04930799450051637 ) ) ;
#12353=ADVANCED_FACE ( 'NONE', ( #3228 ), #28023, .T. ) ;
#12358=EDGE_CURVE ( 'NONE', #21770, #31503, #15542, .T. ) ;
#12362=ORIENTED_EDGE ( 'NONE', *, *, #28119, .F. ) ;
#12365=VECTOR ( 'NONE', #18587, 1000.000000000000000 ) ;
#12375=ORIENTED_EDGE ( 'NONE', *, *, #24233, .F. ) ;
#12379=DIRECTION ( 'NONE',  ( -1.000000000000000000, 0.000000000000000000, 0.000000000000000000 ) ) ;
#12384=VERTEX_POINT ( 'NONE', #20945 ) ;
#12390=FACE_OUTER_BOUND ( 'NONE', #5309, .T. ) ;
#12392=TOROIDAL_SURFACE ( 'NONE', #31251, 12.40141737965284463, 0.1250000000000005274 ) ;
#12394=CARTESIAN_POINT ( 'NONE',  ( 21.09992658989238734, 32.34164230456639899, 47.04930799450051637 ) ) ;
#12395=ORIENTED_EDGE ( 'NONE', *, *, #8269, .T. ) ;
#12399=CARTESIAN_POINT ( 'NONE',  ( 21.09992658989238734, 31.84164230456639544, 47.04930799450051637 ) ) ;
#12402=ORIENTED_EDGE ( 'NONE', *, *, #19585, .F. ) ;
#12404=CARTESIAN_POINT ( 'NONE',  ( 33.72499318558949710, 24.84184655352419213, 47.04930799450051637 ) ) ;
#12407=CARTESIAN_POINT ( 'NONE',  ( 8.823509210239539158, 27.34164230456639544, 47.04930799450051637 ) ) ;
#12408=ORIENTED_EDGE ( 'NONE', *, *, #4753, .F. ) ;
#12410=CARTESIAN_POINT ( 'NONE',  ( 33.72499318558949710, 29.59184655352418858, 47.04930799450051637 ) ) ;
#12411=ORIENTED_EDGE ( 'NONE', *, *, #7120, .F. ) ;
#12417=VERTEX_POINT ( 'NONE', #1731 ) ;
#12418=EDGE_CURVE ( 'NONE', #13126, #25102, #7382, .T. ) ;
#12419=CIRCLE ( 'NONE', #29700, 12.27641737965286062 ) ;
#12420=ORIENTED_EDGE ( 'NONE', *, *, #9116, .T. ) ;
#12421=EDGE_CURVE ( 'NONE', #9009, #6807, #25210, .T. ) ;
#12422=ADVANCED_FACE ( 'NONE', ( #1892 ), #3687, .T. ) ;
#12423=DIRECTION ( 'NONE',  ( -1.224646799147353207E-16, -1.349345573449484691E-32, 1.000000000000000000 ) ) ;
#12427=ORIENTED_EDGE ( 'NONE', *, *, #23159, .T. ) ;
#12434=ORIENTED_EDGE ( 'NONE', *, *, #26982, .F. ) ;
#12440=CARTESIAN_POINT ( 'NONE',  ( 8.698509210239574685, 30.59164230456639544, 47.04930799450051637 ) ) ;
#12442=FACE_OUTER_BOUND ( 'NONE', #1861, .T. ) ;
#12443=DIRECTION ( 'NONE',  ( -1.101824276508909887E-16, 1.000000000000000000, -0.000000000000000000 ) ) ;
#12453=DIRECTION ( 'NONE',  ( -1.000000000000000000, 0.000000000000000000, 0.000000000000000000 ) ) ;
#12455=ORIENTED_EDGE ( 'NONE', *, *, #5071, .F. ) ;
#12459=AXIS2_PLACEMENT_3D ( 'NONE', #9899, #32384, #53 ) ;
#12464=ADVANCED_FACE ( 'NONE', ( #28987 ), #26520, .F. ) ;
#12465=EDGE_CURVE ( 'NONE', #1073, #29330, #24143, .T. ) ;
#12466=ORIENTED_EDGE ( 'NONE', *, *, #29988, .F. ) ;
#12472=DIRECTION ( 'NONE',  ( -1.224646799147353207E-16, -1.349345573449484691E-32, 1.000000000000000000 ) ) ;
#12474=ORIENTED_EDGE ( 'NONE', *, *, #6526, .F. ) ;
#12476=VERTEX_POINT ( 'NONE', #9451 ) ;
#12477=DIRECTION ( 'NONE',  ( -1.000000000000000000, 0.000000000000000000, 0.000000000000000000 ) ) ;
#12479=ORIENTED_EDGE ( 'NONE', *, *, #20835, .T. ) ;
#12481=CARTESIAN_POINT ( 'NONE',  ( 21.09992658989239089, 30.59164230456639544, 47.04930799450051637 ) ) ;
#12492=CIRCLE ( 'NONE', #24510, 12.27641737965287305 ) ;
#12493=DIRECTION ( 'NONE',  ( -1.101824276508909887E-16, 1.000000000000000000, -0.000000000000000000 ) ) ;
#12497=VERTEX_POINT ( 'NONE', #25196 ) ;
#12502=AXIS2_PLACEMENT_3D ( 'NONE', #21037, #13510, #8894 ) ;
#12503=TOROIDAL_SURFACE ( 'NONE', #13526, 12.40141737965288904, 0.1249999999999998612 ) ;
#12508=TOROIDAL_SURFACE ( 'NONE', #2019, 12.61792373059896200, 0.1249999999999979183 ) ;
#12509=ORIENTED_EDGE ( 'NONE', *, *, #11167, .F. ) ;
#12513=VECTOR ( 'NONE', #29415, 1000.000000000000000 ) ;
#12517=DIRECTION ( 'NONE',  ( -1.000000000000000000, 0.000000000000000000, 0.000000000000000000 ) ) ;
#12519=DIRECTION ( 'NONE',  ( -1.101824276508909887E-16, 1.000000000000000000, -0.000000000000000000 ) ) ;
#12527=CARTESIAN_POINT ( 'NONE',  ( 21.09992658989238734, 38.56284415653841791, 47.04930799450051637 ) ) ;
#12533=DIRECTION ( 'NONE',  ( -1.000000000000000000, 0.000000000000000000, 0.000000000000000000 ) ) ;
#12536=EDGE_LOOP ( 'NONE', ( #23432, #14190, #5050, #5640 ) ) ;
#12540=CARTESIAN_POINT ( 'NONE',  ( 8.698509210239512512, 24.59164230456639544, 47.04930799450051637 ) ) ;
#12547=CARTESIAN_POINT ( 'NONE',  ( 21.09992658989238734, 38.56284415653841791, 47.04930799450051637 ) ) ;
#12551=DIRECTION ( 'NONE',  ( -1.000000000000000000, 0.000000000000000000, 0.000000000000000000 ) ) ;
#12553=VERTEX_POINT ( 'NONE', #12407 ) ;
#12554=TOROIDAL_SURFACE ( 'NONE', #8859, 12.40141737965286772, 0.1250000000000003331 ) ;
#12557=CARTESIAN_POINT ( 'NONE',  ( 21.09992658989238734, 38.56284415653841791, 47.04930799450051637 ) ) ;
#12558=DIRECTION ( 'NONE',  ( -1.000000000000000000, 0.000000000000000000, 0.000000000000000000 ) ) ;
#12559=TOROIDAL_SURFACE ( 'NONE', #17321, 12.61792373059858541, 0.1250000000000004996 ) ;
#12562=ORIENTED_EDGE ( 'NONE', *, *, #17456, .T. ) ;
#12563=FACE_OUTER_BOUND ( 'NONE', #9180, .T. ) ;
#12569=DIRECTION ( 'NONE',  ( -1.101824276508909887E-16, 1.000000000000000000, -0.000000000000000000 ) ) ;
#12570=CARTESIAN_POINT ( 'NONE',  ( 33.72499318558949710, 31.09143805560860585, 47.04930799450051637 ) ) ;
#12572=DIRECTION ( 'NONE',  ( -1.000000000000000000, 0.000000000000000000, 0.000000000000000000 ) ) ;
#12574=AXIS2_PLACEMENT_3D ( 'NONE', #31121, #9108, #31761 ) ;
#12576=CARTESIAN_POINT ( 'NONE',  ( 21.09992658989239089, 29.97145308207317527, 47.04930799450051637 ) ) ;
#12580=TOROIDAL_SURFACE ( 'NONE', #4694, 12.40141737965281621, 0.1250000000000009159 ) ;
#12581=CIRCLE ( 'NONE', #2066, 0.1249999999999931721 ) ;
#12587=CIRCLE ( 'NONE', #31433, 12.27641737965284463 ) ;
#12589=AXIS2_PLACEMENT_3D ( 'NONE', #5659, #25679, #30774 ) ;
#12594=ORIENTED_EDGE ( 'NONE', *, *, #11091, .T. ) ;
#12596=FACE_OUTER_BOUND ( 'NONE', #20624, .T. ) ;
#12599=ORIENTED_EDGE ( 'NONE', *, *, #25793, .F. ) ;
#12611=DIRECTION ( 'NONE',  ( -1.101824276508909887E-16, 1.000000000000000000, -0.000000000000000000 ) ) ;
#12616=ORIENTED_EDGE ( 'NONE', *, *, #32291, .T. ) ;
#12624=ORIENTED_EDGE ( 'NONE', *, *, #7038, .F. ) ;
#12625=FACE_OUTER_BOUND ( 'NONE', #25208, .T. ) ;
#12626=AXIS2_PLACEMENT_3D ( 'NONE', #24981, #9884, #27278 ) ;
#12627=EDGE_LOOP ( 'NONE', ( #24988, #8130, #20548, #16835 ) ) ;
#12629=TOROIDAL_SURFACE ( 'NONE', #27273, 12.40141737965287660, 0.1250000000000007772 ) ;
#12632=CIRCLE ( 'NONE', #19963, 12.62506659569710266 ) ;
#12634=AXIS2_PLACEMENT_3D ( 'NONE', #10712, #8084, #200 ) ;
#12636=DIRECTION ( 'NONE',  ( -1.000000000000000000, -1.101824276508909887E-16, 0.000000000000000000 ) ) ;
#12642=ORIENTED_EDGE ( 'NONE', *, *, #27867, .F. ) ;
#12643=EDGE_LOOP ( 'NONE', ( #21220, #17814, #25424, #15596 ) ) ;
#12650=CARTESIAN_POINT ( 'NONE',  ( 33.72499318558949710, 32.09184655352418503, 47.04930799450051637 ) ) ;
#12654=ORIENTED_EDGE ( 'NONE', *, *, #29732, .F. ) ;
#12659=ADVANCED_FACE ( 'NONE', ( #13220 ), #15984, .T. ) ;
#12665=ORIENTED_EDGE ( 'NONE', *, *, #25569, .F. ) ;
#12673=ORIENTED_EDGE ( 'NONE', *, *, #4753, .T. ) ;
#12675=DIRECTION ( 'NONE',  ( -1.224646799147353207E-16, -1.349345573449484691E-32, 1.000000000000000000 ) ) ;
#12677=ORIENTED_EDGE ( 'NONE', *, *, #19376, .F. ) ;
#12681=CARTESIAN_POINT ( 'NONE',  ( 21.09992658989238734, 38.56284415653841791, 47.04930799450051637 ) ) ;
#12684=AXIS2_PLACEMENT_3D ( 'NONE', #19225, #6770, #31084 ) ;
#12685=CARTESIAN_POINT ( 'NONE',  ( 8.474859994195286461, 28.09184655352419213, 47.04930799450051637 ) ) ;
#12688=CARTESIAN_POINT ( 'NONE',  ( 8.823509210239533829, 26.84164230456639899, 47.04930799450051637 ) ) ;
#12694=( NAMED_UNIT ( * ) SI_UNIT ( $, .STERADIAN. ) SOLID_ANGLE_UNIT ( ) );
#12695=ORIENTED_EDGE ( 'NONE', *, *, #27867, .T. ) ;
#12698=CIRCLE ( 'NONE', #3235, 12.36707279061065101 ) ;
#12699=DIRECTION ( 'NONE',  ( -1.101824276508909887E-16, 1.000000000000000000, -0.000000000000000000 ) ) ;
#12701=DIRECTION ( 'NONE',  ( -1.101824276508909887E-16, 1.000000000000000000, -0.000000000000000000 ) ) ;
#12702=ADVANCED_FACE ( 'NONE', ( #14011 ), #11378, .T. ) ;
#12707=CYLINDRICAL_SURFACE ( 'NONE', #26711, 12.36707279061065101 ) ;
#12709=VERTEX_POINT ( 'NONE', #6293 ) ;
#12713=CARTESIAN_POINT ( 'NONE',  ( 33.50134396954526750, 24.59164230456639544, 47.04930799450051637 ) ) ;
#12714=AXIS2_PLACEMENT_3D ( 'NONE', #5040, #32122, #24730 ) ;
#12721=CIRCLE ( 'NONE', #16882, 12.36707279061065101 ) ;
#12728=DIRECTION ( 'NONE',  ( -1.000000000000000000, 0.000000000000000000, 0.000000000000000000 ) ) ;
#12735=CARTESIAN_POINT ( 'NONE',  ( 33.50134396954518223, 32.34164230456639899, 47.04930799450051637 ) ) ;
#12736=EDGE_CURVE ( 'NONE', #3138, #19781, #19232, .T. ) ;
#12749=VERTEX_POINT ( 'NONE', #6778 ) ;
#12753=AXIS2_PLACEMENT_3D ( 'NONE', #25902, #10329, #10495 ) ;
#12755=AXIS2_PLACEMENT_3D ( 'NONE', #22081, #26530, #16508 ) ;
#12759=EDGE_LOOP ( 'NONE', ( #9059, #24334, #24000, #26152 ) ) ;
#12772=DIRECTION ( 'NONE',  ( -1.000000000000000000, -1.101824276508909887E-16, 0.000000000000000000 ) ) ;
#12773=DIRECTION ( 'NONE',  ( -1.000000000000000000, 0.000000000000000000, 0.000000000000000000 ) ) ;
#12774=CARTESIAN_POINT ( 'NONE',  ( 8.474859994195281132, 38.56284415653841791, 47.04930799450051637 ) ) ;
#12779=CIRCLE ( 'NONE', #8064, 12.36707279061065101 ) ;
#12784=EDGE_CURVE ( 'NONE', #3119, #18133, #13680, .T. ) ;
#12785=ORIENTED_EDGE ( 'NONE', *, *, #2527, .T. ) ;
#12794=CIRCLE ( 'NONE', #5963, 12.36707279061065101 ) ;
#12798=EDGE_CURVE ( 'NONE', #27774, #27386, #31513, .T. ) ;
#12801=DIRECTION ( 'NONE',  ( -1.101824276508909887E-16, 1.000000000000000000, -0.000000000000000000 ) ) ;
#12805=FACE_OUTER_BOUND ( 'NONE', #19922, .T. ) ;
#12809=CYLINDRICAL_SURFACE ( 'NONE', #14318, 12.62506659569710266 ) ;
#12811=ADVANCED_BREP_SHAPE_REPRESENTATION ( '', ( #11688, #8172 ), #331 ) ;
#12816=VERTEX_POINT ( 'NONE', #24171 ) ;
#12818=DIRECTION ( 'NONE',  ( 0.000000000000000000, -0.000000000000000000, -1.000000000000000000 ) ) ;
#12819=DIRECTION ( 'NONE',  ( -1.101824276508909887E-16, 1.000000000000000000, -0.000000000000000000 ) ) ;
#12823=CARTESIAN_POINT ( 'NONE',  ( 33.61962556781118394, 32.55121380581068991, 47.04930799450051637 ) ) ;
#12849=EDGE_CURVE ( 'NONE', #3369, #5329, #21018, .T. ) ;
#12851=VERTEX_POINT ( 'NONE', #4808 ) ;
#12855=DIRECTION ( 'NONE',  ( -1.101824276508909887E-16, 1.000000000000000000, -0.000000000000000000 ) ) ;
#12856=AXIS2_PLACEMENT_3D ( 'NONE', #13636, #18859, #26423 ) ;
#12857=ORIENTED_EDGE ( 'NONE', *, *, #26716, .T. ) ;
#12858=CARTESIAN_POINT ( 'NONE',  ( 8.474859994195282908, 38.56284415653841791, 47.04930799450051637 ) ) ;
#12862=ORIENTED_EDGE ( 'NONE', *, *, #31212, .T. ) ;
#12866=AXIS2_PLACEMENT_3D ( 'NONE', #3049, #25061, #17993 ) ;
#12867=AXIS2_PLACEMENT_3D ( 'NONE', #12068, #19928, #31763 ) ;
#12871=ADVANCED_FACE ( 'NONE', ( #2184 ), #12202, .F. ) ;
#12880=TOROIDAL_SURFACE ( 'NONE', #19122, 12.40141737965288193, 0.1250000000000005829 ) ;
#12881=DIRECTION ( 'NONE',  ( -1.000000000000000000, 0.000000000000000000, 0.000000000000000000 ) ) ;
#12882=DIRECTION ( 'NONE',  ( -1.101824276508909887E-16, 1.000000000000000000, -0.000000000000000000 ) ) ;
#12884=AXIS2_PLACEMENT_3D ( 'NONE', #13727, #8949, #20779 ) ;
#12887=CARTESIAN_POINT ( 'NONE',  ( 33.50134396954521065, 30.34164230456639544, 47.04930799450051637 ) ) ;
#12888=ORIENTED_EDGE ( 'NONE', *, *, #1385, .T. ) ;
#12897=DIRECTION ( 'NONE',  ( -1.000000000000000000, -1.101824276508910010E-16, 0.000000000000000000 ) ) ;
#12901=ORIENTED_EDGE ( 'NONE', *, *, #335, .F. ) ;
#12904=VERTEX_POINT ( 'NONE', #20064 ) ;
#12905=CARTESIAN_POINT ( 'NONE',  ( 33.46699938050304013, 31.22145308207317171, 47.04930799450050927 ) ) ;
#12913=ORIENTED_EDGE ( 'NONE', *, *, #9538, .T. ) ;
#12915=CIRCLE ( 'NONE', #21273, 12.36707279061065101 ) ;
#12918=ORIENTED_EDGE ( 'NONE', *, *, #5761, .F. ) ;
#12921=DIRECTION ( 'NONE',  ( -1.101824276508909887E-16, 1.000000000000000000, -0.000000000000000000 ) ) ;
#12923=DIRECTION ( 'NONE',  ( -1.101824276508909887E-16, 1.000000000000000000, -0.000000000000000000 ) ) ;
#12924=ORIENTED_EDGE ( 'NONE', *, *, #28499, .F. ) ;
#12926=CARTESIAN_POINT ( 'NONE',  ( 21.09992658989239089, 30.34164230456639544, 47.04930799450051637 ) ) ;
#12938=DIRECTION ( 'NONE',  ( -1.101824276508909887E-16, 1.000000000000000000, -0.000000000000000000 ) ) ;
#12946=FACE_OUTER_BOUND ( 'NONE', #31416, .T. ) ;
#12949=ADVANCED_FACE ( 'NONE', ( #10557 ), #28753, .T. ) ;
#12952=EDGE_CURVE ( 'NONE', #14341, #3694, #27176, .T. ) ;
#12953=EDGE_LOOP ( 'NONE', ( #9261, #16654, #10841, #3901 ) ) ;
#12956=ADVANCED_FACE ( 'NONE', ( #20708 ), #13587, .T. ) ;
#12959=DIRECTION ( 'NONE',  ( -1.101824276508909887E-16, 1.000000000000000000, -0.000000000000000000 ) ) ;
#12960=CARTESIAN_POINT ( 'NONE',  ( 8.732853799281732776, 38.56284415653841791, 47.04930799450051637 ) ) ;
#12964=CARTESIAN_POINT ( 'NONE',  ( 8.474859994195281132, 32.34143805560860585, 47.04930799450051637 ) ) ;
#12967=DIRECTION ( 'NONE',  ( -1.101824276508909887E-16, 1.000000000000000000, -0.000000000000000000 ) ) ;
#12969=DIRECTION ( 'NONE',  ( -1.101824276508909887E-16, 1.000000000000000000, -0.000000000000000000 ) ) ;
#12973=CARTESIAN_POINT ( 'NONE',  ( 33.71785032049136532, 26.21664230456639899, 47.04930799450051637 ) ) ;
#12976=DIRECTION ( 'NONE',  ( -1.000000000000000000, -1.101824276508909887E-16, 0.000000000000000000 ) ) ;
#12977=DIRECTION ( 'NONE',  ( -1.000000000000000000, 0.000000000000000000, 0.000000000000000000 ) ) ;
#12978=ORIENTED_EDGE ( 'NONE', *, *, #30706, .F. ) ;
#12979=CARTESIAN_POINT ( 'NONE',  ( 33.72499318558949710, 25.59143805560860940, 47.04930799450051637 ) ) ;
#12980=DIRECTION ( 'NONE',  ( -1.101824276508909887E-16, 1.000000000000000000, -0.000000000000000000 ) ) ;
#12981=ADVANCED_FACE ( 'NONE', ( #5464 ), #27710, .T. ) ;
#12982=CARTESIAN_POINT ( 'NONE',  ( 8.732853799281734553, 38.56284415653841791, 47.04930799450051637 ) ) ;
#12983=ORIENTED_EDGE ( 'NONE', *, *, #19280, .F. ) ;
#12985=EDGE_CURVE ( 'NONE', #3694, #14341, #9908, .T. ) ;
#12986=ADVANCED_FACE ( 'NONE', ( #18232 ), #26128, .T. ) ;
#12987=ORIENTED_EDGE ( 'NONE', *, *, #2813, .F. ) ;
#12990=AXIS2_PLACEMENT_3D ( 'NONE', #25638, #6260, #3139 ) ;
#12993=CIRCLE ( 'NONE', #17157, 12.36707279061065101 ) ;
#12999=CARTESIAN_POINT ( 'NONE',  ( 33.46699938050304013, 38.56284415653841791, 47.04930799450051637 ) ) ;
#13002=DIRECTION ( 'NONE',  ( -1.101824276508909887E-16, 1.000000000000000000, -0.000000000000000000 ) ) ;
#13008=ORIENTED_EDGE ( 'NONE', *, *, #2811, .F. ) ;
#13010=CARTESIAN_POINT ( 'NONE',  ( 33.50134396954521065, 30.09164230456639544, 47.04930799450051637 ) ) ;
#13011=DIRECTION ( 'NONE',  ( -1.000000000000000000, -1.101824276508909887E-16, 0.000000000000000000 ) ) ;
#13014=CARTESIAN_POINT ( 'NONE',  ( 33.46699938050304013, 30.97145308207317171, 47.04930799450050927 ) ) ;
#13016=ORIENTED_EDGE ( 'NONE', *, *, #17874, .T. ) ;
#13022=ADVANCED_FACE ( 'NONE', ( #14298 ), #21173, .F. ) ;
#13026=AXIS2_PLACEMENT_3D ( 'NONE', #20373, #12699, #17434 ) ;
#13032=CARTESIAN_POINT ( 'NONE',  ( 21.09992658989238734, 32.21664230456639899, 47.04930799450051637 ) ) ;
#13034=EDGE_LOOP ( 'NONE', ( #6181, #11865, #7998, #23001 ) ) ;
#13039=AXIS2_PLACEMENT_3D ( 'NONE', #657, #23141, #15276 ) ;
#13042=CARTESIAN_POINT ( 'NONE',  ( 21.09992658989238734, 38.56284415653841791, 47.04930799450051637 ) ) ;
#13043=DIRECTION ( 'NONE',  ( -1.101824276508909887E-16, 1.000000000000000000, -0.000000000000000000 ) ) ;
#13044=AXIS2_PLACEMENT_3D ( 'NONE', #15392, #10474, #18166 ) ;
#13051=CARTESIAN_POINT ( 'NONE',  ( 8.823509210239585343, 32.34164230456639899, 47.04930799450051637 ) ) ;
#13055=CARTESIAN_POINT ( 'NONE',  ( 21.09992658989238734, 38.56284415653841791, 47.04930799450051637 ) ) ;
#13056=ORIENTED_EDGE ( 'NONE', *, *, #17786, .T. ) ;
#13057=DIRECTION ( 'NONE',  ( -1.000000000000000000, -1.101824276508909887E-16, 0.000000000000000000 ) ) ;
#13060=CARTESIAN_POINT ( 'NONE',  ( 21.09992658989239089, 30.46183152705961561, 47.04930799450051637 ) ) ;
#13063=ADVANCED_FACE ( 'NONE', ( #1323 ), #23530, .T. ) ;
#13066=EDGE_CURVE ( 'NONE', #28361, #9250, #26596, .T. ) ;
#13070=CIRCLE ( 'NONE', #10461, 12.27641737965286772 ) ;
#13071=AXIS2_PLACEMENT_3D ( 'NONE', #14432, #24427, #26732 ) ;
#13072=EDGE_LOOP ( 'NONE', ( #28018, #11734, #26058, #15009 ) ) ;
#13078=ORIENTED_EDGE ( 'NONE', *, *, #178, .F. ) ;
#13083=ADVANCED_FACE ( 'NONE', ( #26282 ), #28246, .T. ) ;
#13087=ORIENTED_EDGE ( 'NONE', *, *, #17857, .T. ) ;
#13094=EDGE_CURVE ( 'NONE', #16672, #63, #14611, .T. ) ;
#13095=DIRECTION ( 'NONE',  ( -1.000000000000000000, 0.000000000000000000, 0.000000000000000000 ) ) ;
#13096=DIRECTION ( 'NONE',  ( 0.000000000000000000, -0.000000000000000000, -1.000000000000000000 ) ) ;
#13099=DIRECTION ( 'NONE',  ( -1.000000000000000000, 0.000000000000000000, 0.000000000000000000 ) ) ;
#13100=CARTESIAN_POINT ( 'NONE',  ( 21.09992658989238734, 30.84143805560860585, 47.04930799450051637 ) ) ;
#13104=VECTOR ( 'NONE', #27296, 1000.000000000000000 ) ;
#13105=CIRCLE ( 'NONE', #32486, 0.1250000000000001110 ) ;
#13111=AXIS2_PLACEMENT_3D ( 'NONE', #13060, #23220, #17965 ) ;
#13119=AXIS2_PLACEMENT_3D ( 'NONE', #18329, #18494, #5709 ) ;
#13126=VERTEX_POINT ( 'NONE', #9859 ) ;
#13129=CARTESIAN_POINT ( 'NONE',  ( 33.50134396954526039, 25.34164230456639899, 47.04930799450051637 ) ) ;
#13131=DIRECTION ( 'NONE',  ( -1.101824276508909887E-16, 1.000000000000000000, -0.000000000000000000 ) ) ;
#13133=CARTESIAN_POINT ( 'NONE',  ( 8.474859994195286461, 26.59184655352419568, 47.04930799450051637 ) ) ;
#13134=ORIENTED_EDGE ( 'NONE', *, *, #4371, .T. ) ;
#13136=CIRCLE ( 'NONE', #25193, 0.1250000000000001110 ) ;
#13138=ADVANCED_FACE ( 'NONE', ( #4443 ), #17219, .T. ) ;
#13141=ORIENTED_EDGE ( 'NONE', *, *, #24671, .T. ) ;
#13143=DIRECTION ( 'NONE',  ( -1.000000000000000000, 0.000000000000000000, 0.000000000000000000 ) ) ;
#13144=CIRCLE ( 'NONE', #32, 12.36707279061065101 ) ;
#13151=ORIENTED_EDGE ( 'NONE', *, *, #1114, .T. ) ;
#13154=DIRECTION ( 'NONE',  ( -1.000000000000000000, 0.000000000000000000, 0.000000000000000000 ) ) ;
#13156=AXIS2_PLACEMENT_3D ( 'NONE', #23165, #25469, #13333 ) ;
#13159=CARTESIAN_POINT ( 'NONE',  ( 33.46699938050303302, 38.56284415653841791, 47.04930799450051637 ) ) ;
#13167=FACE_OUTER_BOUND ( 'NONE', #11318, .T. ) ;
#13172=CIRCLE ( 'NONE', #9479, 0.1250000000000001110 ) ;
#13178=DIRECTION ( 'NONE',  ( -1.101824276508909887E-16, 1.000000000000000000, -0.000000000000000000 ) ) ;
#13182=EDGE_CURVE ( 'NONE', #7606, #25631, #2559, .T. ) ;
#13186=ADVANCED_FACE ( 'NONE', ( #27580 ), #7404, .F. ) ;
#13189=DIRECTION ( 'NONE',  ( 1.000000000000000000, 0.000000000000000000, 0.000000000000000000 ) ) ;
#13196=TOROIDAL_SURFACE ( 'NONE', #9528, 12.40141737965288371, 0.1249999999999996253 ) ;
#13198=LINE ( 'NONE', #11048, #3572 ) ;
#13199=DIRECTION ( 'NONE',  ( 0.000000000000000000, -0.000000000000000000, -1.000000000000000000 ) ) ;
#13216=DIRECTION ( 'NONE',  ( -1.101824276508909887E-16, 1.000000000000000000, -0.000000000000000000 ) ) ;
#13220=FACE_OUTER_BOUND ( 'NONE', #19987, .T. ) ;
#13221=VECTOR ( 'NONE', #14399, 1000.000000000000000 ) ;
#13231=CARTESIAN_POINT ( 'NONE',  ( 8.698509210239537381, 27.09164230456639899, 47.04930799450051637 ) ) ;
#13232=CARTESIAN_POINT ( 'NONE',  ( 8.474859994195286461, 29.84143805560861296, 47.04930799450051637 ) ) ;
#13237=ORIENTED_EDGE ( 'NONE', *, *, #13854, .F. ) ;
#13238=VECTOR ( 'NONE', #10454, 1000.000000000000000 ) ;
#13240=AXIS2_PLACEMENT_3D ( 'NONE', #27566, #25104, #12477 ) ;
#13241=EDGE_CURVE ( 'NONE', #6908, #19822, #9368, .T. ) ;
#13242=AXIS2_PLACEMENT_3D ( 'NONE', #12289, #26889, #4733 ) ;
#13245=DIRECTION ( 'NONE',  ( -1.101824276508909887E-16, 1.000000000000000000, -0.000000000000000000 ) ) ;
#13247=EDGE_CURVE ( 'NONE', #5204, #12078, #19530, .T. ) ;
#13251=CARTESIAN_POINT ( 'NONE',  ( 21.09992658989239089, 26.97145308207318948, 47.04930799450051637 ) ) ;
#13252=DIRECTION ( 'NONE',  ( -1.101824276508909887E-16, 1.000000000000000000, -0.000000000000000000 ) ) ;
#13257=DIRECTION ( 'NONE',  ( -1.224646799147353207E-16, -1.349345573449484691E-32, 1.000000000000000000 ) ) ;
#13258=CARTESIAN_POINT ( 'NONE',  ( 8.732853799281734553, 38.56284415653841791, 47.04930799450051637 ) ) ;
#13261=DIRECTION ( 'NONE',  ( -1.000000000000000000, 0.000000000000000000, 0.000000000000000000 ) ) ;
#13263=CARTESIAN_POINT ( 'NONE',  ( 21.09992658989238734, 32.47145308207317527, 47.04930799450051637 ) ) ;
#13264=AXIS2_PLACEMENT_3D ( 'NONE', #7555, #4764, #15098 ) ;
#13277=ORIENTED_EDGE ( 'NONE', *, *, #4584, .T. ) ;
#13279=EDGE_CURVE ( 'NONE', #23862, #17110, #5731, .T. ) ;
#13285=ORIENTED_EDGE ( 'NONE', *, *, #31620, .F. ) ;
#13288=CIRCLE ( 'NONE', #26382, 12.62506659569710266 ) ;
#13289=AXIS2_PLACEMENT_3D ( 'NONE', #31010, #23614, #13774 ) ;
#13290=CARTESIAN_POINT ( 'NONE',  ( 33.72499318558949710, 32.34143805560860585, 47.04930799450051637 ) ) ;
#13291=CARTESIAN_POINT ( 'NONE',  ( 8.474859994195281132, 31.84184655352418503, 47.04930799450051637 ) ) ;
#13296=ORIENTED_EDGE ( 'NONE', *, *, #30630, .F. ) ;
#13302=ORIENTED_EDGE ( 'NONE', *, *, #19378, .T. ) ;
#13306=AXIS2_PLACEMENT_3D ( 'NONE', #19113, #21259, #13735 ) ;
#13309=ORIENTED_EDGE ( 'NONE', *, *, #19599, .F. ) ;
#13311=CARTESIAN_POINT ( 'NONE',  ( 21.09992658989239089, 27.09164230456639899, 47.04930799450051637 ) ) ;
#13313=CIRCLE ( 'NONE', #28512, 12.36707279061065101 ) ;
#13316=ORIENTED_EDGE ( 'NONE', *, *, #2110, .T. ) ;
#13319=CARTESIAN_POINT ( 'NONE',  ( 21.09992658989239089, 25.46664230456640254, 47.04930799450051637 ) ) ;
#13322=AXIS2_PLACEMENT_3D ( 'NONE', #18890, #26612, #1989 ) ;
#13323=ORIENTED_EDGE ( 'NONE', *, *, #7613, .F. ) ;
#13328=FACE_OUTER_BOUND ( 'NONE', #2980, .T. ) ;
#13330=CARTESIAN_POINT ( 'NONE',  ( 21.09992658989238734, 31.21664230456641675, 47.04930799450051637 ) ) ;
#13333=DIRECTION ( 'NONE',  ( -1.000000000000000000, 0.000000000000000000, 0.000000000000000000 ) ) ;
#13336=VERTEX_POINT ( 'NONE', #23301 ) ;
#13337=ORIENTED_EDGE ( 'NONE', *, *, #6435, .T. ) ;
#13340=EDGE_LOOP ( 'NONE', ( #15127, #11169, #19897, #25747 ) ) ;
#13349=AXIS2_PLACEMENT_3D ( 'NONE', #5042, #19960, #24237 ) ;
#13350=AXIS2_PLACEMENT_3D ( 'NONE', #2000, #26464, #26788 ) ;
#13351=ORIENTED_EDGE ( 'NONE', *, *, #27505, .F. ) ;
#13356=ADVANCED_FACE ( 'NONE', ( #7888 ), #9405, .T. ) ;
#13358=ADVANCED_FACE ( 'NONE', ( #2632 ), #13603, .T. ) ;
#13366=CARTESIAN_POINT ( 'NONE',  ( 21.09992658989239089, 26.09184655352419213, 47.04930799450051637 ) ) ;
#13370=ORIENTED_EDGE ( 'NONE', *, *, #29043, .T. ) ;
#13376=DIRECTION ( 'NONE',  ( -1.101824276508909887E-16, 1.000000000000000000, -0.000000000000000000 ) ) ;
#13381=CARTESIAN_POINT ( 'NONE',  ( 8.698509210239558698, 29.09164230456639899, 47.04930799450051637 ) ) ;
#13383=ORIENTED_EDGE ( 'NONE', *, *, #31430, .T. ) ;
#13386=CARTESIAN_POINT ( 'NONE',  ( 21.09992658989239089, 27.21183152705960495, 47.04930799450051637 ) ) ;
#13388=ORIENTED_EDGE ( 'NONE', *, *, #4750, .T. ) ;
#13394=TOROIDAL_SURFACE ( 'NONE', #21232, 12.40141737965282154, 0.1250000000000006939 ) ;
#13395=CIRCLE ( 'NONE', #14441, 12.36707279061065101 ) ;
#13402=VERTEX_POINT ( 'NONE', #23937 ) ;
#13412=CARTESIAN_POINT ( 'NONE',  ( 33.72499318558949710, 32.34184655352418503, 47.04930799450051637 ) ) ;
#13418=DIRECTION ( 'NONE',  ( -1.101824276508909887E-16, 1.000000000000000000, -0.000000000000000000 ) ) ;
#13420=ORIENTED_EDGE ( 'NONE', *, *, #11886, .F. ) ;
#13427=ADVANCED_FACE ( 'NONE', ( #29032 ), #12554, .T. ) ;
#13428=DIRECTION ( 'NONE',  ( -1.000000000000000000, -1.101824276508909887E-16, 0.000000000000000000 ) ) ;
#13431=CYLINDRICAL_SURFACE ( 'NONE', #13119, 12.36707279061065101 ) ;
#13432=ADVANCED_FACE ( 'NONE', ( #11156 ), #17783, .T. ) ;
#13435=CIRCLE ( 'NONE', #21794, 12.36707279061065279 ) ;
#13438=DIRECTION ( 'NONE',  ( -1.000000000000000000, 0.000000000000000000, 0.000000000000000000 ) ) ;
#13439=EDGE_CURVE ( 'NONE', #8460, #9948, #19165, .T. ) ;
#13441=VERTEX_POINT ( 'NONE', #31180 ) ;
#13446=ORIENTED_EDGE ( 'NONE', *, *, #7689, .T. ) ;
#13449=EDGE_LOOP ( 'NONE', ( #17858, #12408, #31130, #18809 ) ) ;
#13456=ADVANCED_FACE ( 'NONE', ( #5909 ), #3594, .T. ) ;
#13460=FACE_OUTER_BOUND ( 'NONE', #14188, .T. ) ;
#13463=CARTESIAN_POINT ( 'NONE',  ( 21.09992658989238734, 38.56284415653841791, 47.04930799450051637 ) ) ;
#13464=EDGE_LOOP ( 'NONE', ( #4369, #24723, #4881, #19868 ) ) ;
#13467=ADVANCED_FACE ( 'NONE', ( #11466 ), #25917, .T. ) ;
#13468=AXIS2_PLACEMENT_3D ( 'NONE', #12973, #18515, #22960 ) ;
#13469=EDGE_CURVE ( 'NONE', #17250, #20645, #17241, .T. ) ;
#13470=EDGE_CURVE ( 'NONE', #7990, #2384, #31919, .T. ) ;
#13471=ORIENTED_EDGE ( 'NONE', *, *, #29543, .T. ) ;
#13472=CIRCLE ( 'NONE', #15547, 12.36707279061065279 ) ;
#13475=CARTESIAN_POINT ( 'NONE',  ( 8.732853799281732776, 31.96183152705962272, 47.04930799450051637 ) ) ;
#13481=ORIENTED_EDGE ( 'NONE', *, *, #178, .T. ) ;
#13483=ORIENTED_EDGE ( 'NONE', *, *, #6806, .T. ) ;
#13487=DIRECTION ( 'NONE',  ( -1.101824276508909887E-16, 1.000000000000000000, -0.000000000000000000 ) ) ;
#13488=DIRECTION ( 'NONE',  ( 1.000000000000000000, 0.000000000000000000, 0.000000000000000000 ) ) ;
#13491=ORIENTED_EDGE ( 'NONE', *, *, #32480, .F. ) ;
#13493=DIRECTION ( 'NONE',  ( -1.101824276508909887E-16, 1.000000000000000000, -0.000000000000000000 ) ) ;
#13495=DIRECTION ( 'NONE',  ( -1.101824276508909887E-16, 1.000000000000000000, -0.000000000000000000 ) ) ;
#13499=DIRECTION ( 'NONE',  ( -1.101824276508909887E-16, 1.000000000000000000, -0.000000000000000000 ) ) ;
#13500=ORIENTED_EDGE ( 'NONE', *, *, #5988, .F. ) ;
#13510=DIRECTION ( 'NONE',  ( -1.101824276508909887E-16, 1.000000000000000000, -0.000000000000000000 ) ) ;
#13512=AXIS2_PLACEMENT_3D ( 'NONE', #13714, #25853, #11097 ) ;
#13520=FACE_OUTER_BOUND ( 'NONE', #17395, .T. ) ;
#13522=ORIENTED_EDGE ( 'NONE', *, *, #19977, .F. ) ;
#13524=AXIS2_PLACEMENT_3D ( 'NONE', #6423, #1485, #9045 ) ;
#13526=AXIS2_PLACEMENT_3D ( 'NONE', #24727, #4869, #25050 ) ;
#13527=LINE ( 'NONE', #21534, #8805 ) ;
#13532=DIRECTION ( 'NONE',  ( -1.000000000000000000, -1.101824276508909764E-16, 0.000000000000000000 ) ) ;
#13533=AXIS2_PLACEMENT_3D ( 'NONE', #10150, #17025, #19494 ) ;
#13536=FACE_OUTER_BOUND ( 'NONE', #27917, .T. ) ;
#13538=AXIS2_PLACEMENT_3D ( 'NONE', #191, #27762, #24648 ) ;
#13543=VERTEX_POINT ( 'NONE', #7194 ) ;
#13544=TOROIDAL_SURFACE ( 'NONE', #12502, 12.40141737965283397, 0.1249999999999992922 ) ;
#13546=TOROIDAL_SURFACE ( 'NONE', #11451, 12.40141737965285174, 0.1249999999999993200 ) ;
#13548=AXIS2_PLACEMENT_3D ( 'NONE', #2911, #28359, #23098 ) ;
#13552=AXIS2_PLACEMENT_3D ( 'NONE', #8402, #520, #8245 ) ;
#13554=ORIENTED_EDGE ( 'NONE', *, *, #429, .F. ) ;
#13561=CARTESIAN_POINT ( 'NONE',  ( 21.09992658989239089, 24.84143805560860940, 47.04930799450051637 ) ) ;
#13562=VERTEX_POINT ( 'NONE', #25366 ) ;
#13563=DIRECTION ( 'NONE',  ( -1.224646799147353207E-16, -1.349345573449484691E-32, 1.000000000000000000 ) ) ;
#13564=CARTESIAN_POINT ( 'NONE',  ( 33.72499318558949000, 38.56284415653841791, 47.04930799450051637 ) ) ;
#13565=EDGE_LOOP ( 'NONE', ( #11445, #22323, #11840, #20505 ) ) ;
#13566=CYLINDRICAL_SURFACE ( 'NONE', #2743, 12.62506659569710266 ) ;
#13570=CARTESIAN_POINT ( 'NONE',  ( 33.46699938050304013, 29.71183152705961561, 47.04930799450051637 ) ) ;
#13571=ORIENTED_EDGE ( 'NONE', *, *, #24563, .T. ) ;
#13572=DIRECTION ( 'NONE',  ( -1.101824276508909887E-16, 1.000000000000000000, -0.000000000000000000 ) ) ;
#13579=VECTOR ( 'NONE', #18042, 1000.000000000000000 ) ;
#13586=ADVANCED_FACE ( 'NONE', ( #19497 ), #30359, .T. ) ;
#13587=TOROIDAL_SURFACE ( 'NONE', #3592, 12.61792373059891403, 0.1250000000000023315 ) ;
#13589=VERTEX_POINT ( 'NONE', #9328 ) ;
#13591=AXIS2_PLACEMENT_3D ( 'NONE', #10293, #24731, #5369 ) ;
#13597=EDGE_CURVE ( 'NONE', #3694, #17205, #2042, .T. ) ;
#13598=ORIENTED_EDGE ( 'NONE', *, *, #25292, .T. ) ;
#13603=TOROIDAL_SURFACE ( 'NONE', #18292, 12.61792373059893535, 0.1249999999999994033 ) ;
#13604=CARTESIAN_POINT ( 'NONE',  ( 21.09992658989239089, 24.97145308207319303, 47.04930799450051637 ) ) ;
#13605=CARTESIAN_POINT ( 'NONE',  ( 8.732853799281732776, 38.56284415653841791, 47.04930799450051637 ) ) ;
#13607=AXIS2_PLACEMENT_3D ( 'NONE', #32317, #27552, #7369 ) ;
#13614=DIRECTION ( 'NONE',  ( -1.101824276508909887E-16, 1.000000000000000000, -0.000000000000000000 ) ) ;
#13615=DIRECTION ( 'NONE',  ( -1.000000000000000000, -1.101824276508910010E-16, 0.000000000000000000 ) ) ;
#13616=CARTESIAN_POINT ( 'NONE',  ( 21.09992658989239089, 28.22145308207318237, 47.04930799450051637 ) ) ;
#13618=EDGE_LOOP ( 'NONE', ( #18704, #19680, #28649, #21761 ) ) ;
#13620=LINE ( 'NONE', #1136, #5158 ) ;
#13623=AXIS2_PLACEMENT_3D ( 'NONE', #7285, #22206, #17112 ) ;
#13624=EDGE_LOOP ( 'NONE', ( #28344, #5501, #28453, #16509 ) ) ;
#13626=AXIS2_PLACEMENT_3D ( 'NONE', #5128, #30402, #27770 ) ;
#13630=CIRCLE ( 'NONE', #2100, 12.36707279061065279 ) ;
#13631=DIRECTION ( 'NONE',  ( -1.101824276508909887E-16, 1.000000000000000000, -0.000000000000000000 ) ) ;
#13632=DIRECTION ( 'NONE',  ( -1.101824276508909887E-16, 1.000000000000000000, -0.000000000000000000 ) ) ;
#13633=EDGE_CURVE ( 'NONE', #13336, #30065, #27223, .T. ) ;
#13636=CARTESIAN_POINT ( 'NONE',  ( 33.50134396954518223, 32.34164230456639899, 47.04930799450051637 ) ) ;
#13637=CARTESIAN_POINT ( 'NONE',  ( 8.482002859293778840, 29.96664230456641675, 47.04930799450051637 ) ) ;
#13649=PRESENTATION_STYLE_ASSIGNMENT (( #5938 ) ) ;
#13650=EDGE_LOOP ( 'NONE', ( #5557, #23552, #23561, #24044 ) ) ;
#13651=VERTEX_POINT ( 'NONE', #18601 ) ;
#13657=CARTESIAN_POINT ( 'NONE',  ( 21.09992658989238734, 31.96664230456639544, 47.04930799450051637 ) ) ;
#13658=AXIS2_PLACEMENT_3D ( 'NONE', #24126, #9529, #4436 ) ;
#13659=CARTESIAN_POINT ( 'NONE',  ( 33.46699938050303302, 38.56284415653841791, 47.04930799450051637 ) ) ;
#13660=ORIENTED_EDGE ( 'NONE', *, *, #3846, .T. ) ;
#13662=CIRCLE ( 'NONE', #16772, 0.1250000000000001110 ) ;
#13665=AXIS2_PLACEMENT_3D ( 'NONE', #28117, #2987, #3144 ) ;
#13668=ORIENTED_EDGE ( 'NONE', *, *, #14034, .F. ) ;
#13670=DIRECTION ( 'NONE',  ( -1.000000000000000000, 0.000000000000000000, 0.000000000000000000 ) ) ;
#13673=AXIS2_PLACEMENT_3D ( 'NONE', #22231, #29301, #17477 ) ;
#13678=AXIS2_PLACEMENT_3D ( 'NONE', #15860, #5526, #5686 ) ;
#13680=CIRCLE ( 'NONE', #32025, 12.62506659569710266 ) ;
#13681=ADVANCED_FACE ( 'NONE', ( #13536 ), #25523, .F. ) ;
#13682=ORIENTED_EDGE ( 'NONE', *, *, #17938, .T. ) ;
#13685=FACE_OUTER_BOUND ( 'NONE', #29558, .T. ) ;
#13689=DIRECTION ( 'NONE',  ( -1.101824276508909887E-16, 1.000000000000000000, -0.000000000000000000 ) ) ;
#13698=DIRECTION ( 'NONE',  ( -1.000000000000000000, 0.000000000000000000, 0.000000000000000000 ) ) ;
#13700=FACE_OUTER_BOUND ( 'NONE', #3143, .T. ) ;
#13701=DIRECTION ( 'NONE',  ( -1.224646799147353207E-16, -1.349345573449484691E-32, 1.000000000000000000 ) ) ;
#13704=ORIENTED_EDGE ( 'NONE', *, *, #31181, .T. ) ;
#13707=EDGE_LOOP ( 'NONE', ( #19287, #5308, #8872, #18027 ) ) ;
#13709=CIRCLE ( 'NONE', #17895, 12.27641737965284641 ) ;
#13710=ORIENTED_EDGE ( 'NONE', *, *, #24694, .F. ) ;
#13714=CARTESIAN_POINT ( 'NONE',  ( 21.09992658989238734, 32.34164230456639899, 47.04930799450051637 ) ) ;
#13721=CARTESIAN_POINT ( 'NONE',  ( 8.698509210239581790, 31.84164230456639544, 47.04930799450051637 ) ) ;
#13726=ORIENTED_EDGE ( 'NONE', *, *, #9867, .F. ) ;
#13727=CARTESIAN_POINT ( 'NONE',  ( 21.09992658989239089, 28.84184655352418858, 47.04930799450051637 ) ) ;
#13729=DIRECTION ( 'NONE',  ( -1.101824276508909887E-16, 1.000000000000000000, -0.000000000000000000 ) ) ;
#13735=DIRECTION ( 'NONE',  ( -1.000000000000000000, -1.101824276508909764E-16, 0.000000000000000000 ) ) ;
#13742=AXIS2_PLACEMENT_3D ( 'NONE', #17348, #14408, #12277 ) ;
#13745=ORIENTED_EDGE ( 'NONE', *, *, #17068, .T. ) ;
#13747=ORIENTED_EDGE ( 'NONE', *, *, #2763, .F. ) ;
#13749=ORIENTED_EDGE ( 'NONE', *, *, #11565, .F. ) ;
#13750=CARTESIAN_POINT ( 'NONE',  ( 33.46699938050304013, 26.46183152705960140, 47.04930799450051637 ) ) ;
#13756=DIRECTION ( 'NONE',  ( -1.101824276508909887E-16, 1.000000000000000000, -0.000000000000000000 ) ) ;
#13757=EDGE_CURVE ( 'NONE', #29229, #26728, #11004, .T. ) ;
#13760=EDGE_CURVE ( 'NONE', #28587, #21198, #21995, .T. ) ;
#13766=EDGE_LOOP ( 'NONE', ( #25171, #20963, #32447, #4837 ) ) ;
#13768=VECTOR ( 'NONE', #4056, 1000.000000000000000 ) ;
#13774=DIRECTION ( 'NONE',  ( -1.000000000000000000, 0.000000000000000000, 0.000000000000000000 ) ) ;
#13778=CARTESIAN_POINT ( 'NONE',  ( 21.09992658989239089, 27.72145308207318237, 47.04930799450051637 ) ) ;
#13781=DIRECTION ( 'NONE',  ( -1.000000000000000000, 0.000000000000000000, 0.000000000000000000 ) ) ;
#13783=CARTESIAN_POINT ( 'NONE',  ( 8.474859994195282908, 38.56284415653841791, 47.04930799450051637 ) ) ;
#13788=EDGE_CURVE ( 'NONE', #9936, #21917, #12581, .T. ) ;
#13789=CIRCLE ( 'NONE', #16377, 0.1250000000000001110 ) ;
#13790=VERTEX_POINT ( 'NONE', #29273 ) ;
#13804=AXIS2_PLACEMENT_3D ( 'NONE', #24576, #17519, #22109 ) ;
#13805=DIRECTION ( 'NONE',  ( -1.101824276508909887E-16, 1.000000000000000000, -0.000000000000000000 ) ) ;
#13806=TOROIDAL_SURFACE ( 'NONE', #31109, 12.61792373059896377, 0.1249999999999977518 ) ;
#13808=ORIENTED_EDGE ( 'NONE', *, *, #18116, .T. ) ;
#13809=ORIENTED_EDGE ( 'NONE', *, *, #31820, .F. ) ;
#13810=CARTESIAN_POINT ( 'NONE',  ( 33.46699938050304013, 27.72145308207318237, 47.04930799450050927 ) ) ;
#13811=DIRECTION ( 'NONE',  ( -1.101824276508909887E-16, 1.000000000000000000, -0.000000000000000000 ) ) ;
#13815=AXIS2_PLACEMENT_3D ( 'NONE', #16624, #19246, #16309 ) ;
#13816=CARTESIAN_POINT ( 'NONE',  ( 21.09992658989238734, 31.34164230456639544, 47.04930799450051637 ) ) ;
#13825=EDGE_CURVE ( 'NONE', #19067, #28626, #4695, .T. ) ;
#13826=EDGE_CURVE ( 'NONE', #20581, #10115, #23582, .T. ) ;
#13828=AXIS2_PLACEMENT_3D ( 'NONE', #31071, #31233, #16116 ) ;
#13829=CARTESIAN_POINT ( 'NONE',  ( 21.09992658989238734, 38.56284415653841791, 47.04930799450051637 ) ) ;
#13833=ORIENTED_EDGE ( 'NONE', *, *, #16184, .F. ) ;
#13837=EDGE_CURVE ( 'NONE', #10473, #11669, #13105, .T. ) ;
#13840=DIRECTION ( 'NONE',  ( 0.000000000000000000, -0.000000000000000000, -1.000000000000000000 ) ) ;
#13842=DIRECTION ( 'NONE',  ( -1.101824276508909887E-16, 1.000000000000000000, -0.000000000000000000 ) ) ;
#13843=FACE_OUTER_BOUND ( 'NONE', #7511, .T. ) ;
#13846=DIRECTION ( 'NONE',  ( -1.000000000000000000, 0.000000000000000000, 0.000000000000000000 ) ) ;
#13847=DIRECTION ( 'NONE',  ( -1.101824276508909887E-16, 1.000000000000000000, -0.000000000000000000 ) ) ;
#13850=ORIENTED_EDGE ( 'NONE', *, *, #30810, .F. ) ;
#13854=EDGE_CURVE ( 'NONE', #30180, #15469, #30378, .T. ) ;
#13858=TOROIDAL_SURFACE ( 'NONE', #13350, 12.40141737965279667, 0.1249999999999991951 ) ;
#13859=CARTESIAN_POINT ( 'NONE',  ( 33.50134396954521065, 30.34164230456639544, 47.04930799450051637 ) ) ;
#13866=VERTEX_POINT ( 'NONE', #16623 ) ;
#13871=CARTESIAN_POINT ( 'NONE',  ( 21.09992658989239089, 25.21664230456640254, 47.04930799450051637 ) ) ;
#13875=AXIS2_PLACEMENT_3D ( 'NONE', #23485, #997, #11021 ) ;
#13876=CIRCLE ( 'NONE', #32237, 0.1250000000000001110 ) ;
#13879=ORIENTED_EDGE ( 'NONE', *, *, #9183, .F. ) ;
#13881=FACE_OUTER_BOUND ( 'NONE', #18529, .T. ) ;
#13883=CARTESIAN_POINT ( 'NONE',  ( 21.09992658989238734, 32.09164230456639899, 47.04930799450051637 ) ) ;
#13887=DIRECTION ( 'NONE',  ( -1.000000000000000000, 0.000000000000000000, 0.000000000000000000 ) ) ;
#13891=FACE_OUTER_BOUND ( 'NONE', #25148, .T. ) ;
#13903=EDGE_LOOP ( 'NONE', ( #14403, #326, #1003, #18131 ) ) ;
#13907=CIRCLE ( 'NONE', #24922, 12.36707279061065279 ) ;
#13913=ORIENTED_EDGE ( 'NONE', *, *, #14633, .F. ) ;
#13917=FACE_OUTER_BOUND ( 'NONE', #25015, .T. ) ;
#13918=DIRECTION ( 'NONE',  ( -1.101824276508909887E-16, 1.000000000000000000, -0.000000000000000000 ) ) ;
#13920=AXIS2_PLACEMENT_3D ( 'NONE', #11987, #4924, #157 ) ;
#13937=DIRECTION ( 'NONE',  ( -1.000000000000000000, 0.000000000000000000, 0.000000000000000000 ) ) ;
#13938=CARTESIAN_POINT ( 'NONE',  ( 8.732853799281732776, 31.46183152705961561, 47.04930799450051637 ) ) ;
#13940=AXIS2_PLACEMENT_3D ( 'NONE', #23948, #24113, #32326 ) ;
#13947=DIRECTION ( 'NONE',  ( -1.000000000000000000, -1.101824276508909764E-16, 0.000000000000000000 ) ) ;
#13951=EDGE_CURVE ( 'NONE', #14214, #30931, #30918, .T. ) ;
#13960=EDGE_LOOP ( 'NONE', ( #14061, #24807, #6341, #18938 ) ) ;
#13965=VERTEX_POINT ( 'NONE', #27301 ) ;
#13966=DIRECTION ( 'NONE',  ( -1.000000000000000000, 0.000000000000000000, 0.000000000000000000 ) ) ;
#13972=ORIENTED_EDGE ( 'NONE', *, *, #30298, .F. ) ;
#13977=DIRECTION ( 'NONE',  ( -1.000000000000000000, -1.101824276508909887E-16, 0.000000000000000000 ) ) ;
#13978=VERTEX_POINT ( 'NONE', #30258 ) ;
#13980=DIRECTION ( 'NONE',  ( -1.224646799147353207E-16, -1.349345573449484691E-32, 1.000000000000000000 ) ) ;
#13984=AXIS2_PLACEMENT_3D ( 'NONE', #24473, #4786, #12179 ) ;
#13985=DIRECTION ( 'NONE',  ( -1.000000000000000000, 0.000000000000000000, 0.000000000000000000 ) ) ;
#13987=EDGE_CURVE ( 'NONE', #30065, #13965, #7324, .T. ) ;
#13988=EDGE_CURVE ( 'NONE', #29931, #25766, #2362, .T. ) ;
#13989=EDGE_CURVE ( 'NONE', #5841, #3723, #24601, .T. ) ;
#13993=AXIS2_PLACEMENT_3D ( 'NONE', #28623, #22199, #27126 ) ;
#13994=DIRECTION ( 'NONE',  ( -1.224646799147353207E-16, -1.349345573449484691E-32, 1.000000000000000000 ) ) ;
#13997=CARTESIAN_POINT ( 'NONE',  ( 21.09992658989239089, 30.34164230456639544, 47.04930799450051637 ) ) ;
#14000=FACE_OUTER_BOUND ( 'NONE', #26837, .T. ) ;
#14002=CARTESIAN_POINT ( 'NONE',  ( 21.09992658989239089, 29.59164230456639899, 47.04930799450051637 ) ) ;
#14006=FACE_OUTER_BOUND ( 'NONE', #12643, .T. ) ;
#14009=CARTESIAN_POINT ( 'NONE',  ( 21.09992658989238734, 38.56284415653841791, 47.04930799450051637 ) ) ;
#14010=DIRECTION ( 'NONE',  ( -1.101824276508909887E-16, 1.000000000000000000, -0.000000000000000000 ) ) ;
#14011=FACE_OUTER_BOUND ( 'NONE', #7268, .T. ) ;
#14017=CARTESIAN_POINT ( 'NONE',  ( 21.09992658989239089, 28.09164230456639544, 47.04930799450051637 ) ) ;
#14018=FACE_OUTER_BOUND ( 'NONE', #16607, .T. ) ;
#14025=ORIENTED_EDGE ( 'NONE', *, *, #19599, .T. ) ;
#14027=ORIENTED_EDGE ( 'NONE', *, *, #25645, .T. ) ;
#14031=DIRECTION ( 'NONE',  ( -1.000000000000000000, 0.000000000000000000, 0.000000000000000000 ) ) ;
#14034=EDGE_CURVE ( 'NONE', #5457, #8522, #8401, .T. ) ;
#14038=DIRECTION ( 'NONE',  ( -1.101824276508909887E-16, 1.000000000000000000, -0.000000000000000000 ) ) ;
#14039=CIRCLE ( 'NONE', #11959, 12.36707279061065101 ) ;
#14040=EDGE_LOOP ( 'NONE', ( #5058, #30549, #3527, #28291 ) ) ;
#14042=DIRECTION ( 'NONE',  ( -1.101824276508909887E-16, 1.000000000000000000, -0.000000000000000000 ) ) ;
#14043=DIRECTION ( 'NONE',  ( -1.000000000000000000, 0.000000000000000000, 0.000000000000000000 ) ) ;
#14051=CARTESIAN_POINT ( 'NONE',  ( 33.50134396954526750, 25.09164230456639899, 47.04930799450051637 ) ) ;
#14052=DIRECTION ( 'NONE',  ( -1.101824276508909887E-16, 1.000000000000000000, -0.000000000000000000 ) ) ;
#14061=ORIENTED_EDGE ( 'NONE', *, *, #21884, .F. ) ;
#14062=ORIENTED_EDGE ( 'NONE', *, *, #3589, .T. ) ;
#14069=AXIS2_PLACEMENT_3D ( 'NONE', #5023, #15033, #9939 ) ;
#14074=EDGE_LOOP ( 'NONE', ( #17514, #21164, #31110, #15095 ) ) ;
#14076=DIRECTION ( 'NONE',  ( -1.000000000000000000, 0.000000000000000000, 0.000000000000000000 ) ) ;
#14083=ADVANCED_FACE ( 'NONE', ( #32364 ), #15725, .T. ) ;
#14084=ORIENTED_EDGE ( 'NONE', *, *, #4528, .T. ) ;
#14087=CIRCLE ( 'NONE', #24026, 12.62506659569710266 ) ;
#14091=ADVANCED_FACE ( 'NONE', ( #19711 ), #11032, .T. ) ;
#14109=AXIS2_PLACEMENT_3D ( 'NONE', #2287, #15086, #20164 ) ;
#14111=ORIENTED_EDGE ( 'NONE', *, *, #8574, .T. ) ;
#14113=DIRECTION ( 'NONE',  ( -1.000000000000000000, -1.101824276508909887E-16, 0.000000000000000000 ) ) ;
#14115=ORIENTED_EDGE ( 'NONE', *, *, #7949, .F. ) ;
#14116=CARTESIAN_POINT ( 'NONE',  ( 21.09992658989238734, 38.56284415653841791, 47.04930799450051637 ) ) ;
#14120=ORIENTED_EDGE ( 'NONE', *, *, #4018, .F. ) ;
#14121=CARTESIAN_POINT ( 'NONE',  ( 8.732853799281732776, 38.56284415653841791, 47.04930799450051637 ) ) ;
#14137=ORIENTED_EDGE ( 'NONE', *, *, #23578, .F. ) ;
#14139=CARTESIAN_POINT ( 'NONE',  ( 21.09992658989239089, 30.59164230456639544, 47.04930799450051637 ) ) ;
#14141=DIRECTION ( 'NONE',  ( -1.000000000000000000, 0.000000000000000000, 0.000000000000000000 ) ) ;
#14142=CARTESIAN_POINT ( 'NONE',  ( 21.09992658989239089, 26.34164230456639899, 47.04930799450051637 ) ) ;
#14143=TOROIDAL_SURFACE ( 'NONE', #4169, 12.40141737965281266, 0.1249999999999994865 ) ;
#14146=AXIS2_PLACEMENT_3D ( 'NONE', #9826, #457, #14917 ) ;
#14153=AXIS2_PLACEMENT_3D ( 'NONE', #27643, #22059, #17130 ) ;
#14154=TOROIDAL_SURFACE ( 'NONE', #3125, 12.40141737965284463, 0.1250000000000005274 ) ;
#14160=AXIS2_PLACEMENT_3D ( 'NONE', #8069, #340, #16080 ) ;
#14164=CARTESIAN_POINT ( 'NONE',  ( 21.09992658989239089, 28.21664230456639899, 47.04930799450051637 ) ) ;
#14168=EDGE_CURVE ( 'NONE', #3389, #22214, #20962, .T. ) ;
#14170=EDGE_CURVE ( 'NONE', #11810, #231, #20433, .T. ) ;
#14179=DIRECTION ( 'NONE',  ( -1.101824276508909887E-16, 1.000000000000000000, -0.000000000000000000 ) ) ;
#14182=ORIENTED_EDGE ( 'NONE', *, *, #25212, .F. ) ;
#14187=DIRECTION ( 'NONE',  ( -1.101824276508909887E-16, 1.000000000000000000, -0.000000000000000000 ) ) ;
#14188=EDGE_LOOP ( 'NONE', ( #14768, #1062, #22405, #8321 ) ) ;
#14190=ORIENTED_EDGE ( 'NONE', *, *, #32080, .F. ) ;
#14191=AXIS2_PLACEMENT_3D ( 'NONE', #7557, #648, #7713 ) ;
#14195=CIRCLE ( 'NONE', #27837, 12.36707279061065101 ) ;
#14198=EDGE_CURVE ( 'NONE', #27550, #15557, #29896, .T. ) ;
#14202=DIRECTION ( 'NONE',  ( 0.000000000000000000, -0.000000000000000000, -1.000000000000000000 ) ) ;
#14203=AXIS2_PLACEMENT_3D ( 'NONE', #31964, #31485, #31803 ) ;
#14207=FACE_OUTER_BOUND ( 'NONE', #18680, .T. ) ;
#14209=ADVANCED_FACE ( 'NONE', ( #17905 ), #19916, .T. ) ;
#14214=VERTEX_POINT ( 'NONE', #23151 ) ;
#14217=DIRECTION ( 'NONE',  ( -1.000000000000000000, 0.000000000000000000, 0.000000000000000000 ) ) ;
#14223=ORIENTED_EDGE ( 'NONE', *, *, #18640, .T. ) ;
#14227=ORIENTED_EDGE ( 'NONE', *, *, #22787, .F. ) ;
#14233=EDGE_CURVE ( 'NONE', #1027, #30099, #518, .T. ) ;
#14236=AXIS2_PLACEMENT_3D ( 'NONE', #23576, #5543, #3715 ) ;
#14239=LINE ( 'NONE', #11439, #1665 ) ;
#14241=DIRECTION ( 'NONE',  ( -1.101824276508909887E-16, 1.000000000000000000, -0.000000000000000000 ) ) ;
#14252=DIRECTION ( 'NONE',  ( -1.224646799147353207E-16, -1.349345573449484691E-32, 1.000000000000000000 ) ) ;
#14260=DIRECTION ( 'NONE',  ( -1.000000000000000000, 0.000000000000000000, 0.000000000000000000 ) ) ;
#14261=DIRECTION ( 'NONE',  ( -1.101824276508909887E-16, 1.000000000000000000, -0.000000000000000000 ) ) ;
#14262=CARTESIAN_POINT ( 'NONE',  ( 8.732853799281729223, 26.97145308207318948, 47.04930799450051637 ) ) ;
#14267=VERTEX_POINT ( 'NONE', #3286 ) ;
#14269=CIRCLE ( 'NONE', #5363, 12.52641737965288904 ) ;
#14271=ORIENTED_EDGE ( 'NONE', *, *, #31685, .F. ) ;
#14276=EDGE_CURVE ( 'NONE', #30857, #6807, #16234, .T. ) ;
#14277=EDGE_CURVE ( 'NONE', #21198, #2570, #30947, .T. ) ;
#14278=ORIENTED_EDGE ( 'NONE', *, *, #23857, .F. ) ;
#14280=DIRECTION ( 'NONE',  ( -1.101824276508909887E-16, 1.000000000000000000, -0.000000000000000000 ) ) ;
#14283=VERTEX_POINT ( 'NONE', #16886 ) ;
#14285=TOROIDAL_SURFACE ( 'NONE', #13242, 12.61792373059859607, 0.1249999999999979738 ) ;
#14289=CARTESIAN_POINT ( 'NONE',  ( 21.09992658989238734, 38.56284415653841791, 47.04930799450051637 ) ) ;
#14291=CARTESIAN_POINT ( 'NONE',  ( 21.09992658989239089, 29.84164230456639899, 47.04930799450051637 ) ) ;
#14293=DIRECTION ( 'NONE',  ( -1.000000000000000000, 0.000000000000000000, 0.000000000000000000 ) ) ;
#14297=CARTESIAN_POINT ( 'NONE',  ( 33.37634396954520355, 30.59164230456639544, 47.04930799450051637 ) ) ;
#14298=FACE_OUTER_BOUND ( 'NONE', #24447, .T. ) ;
#14299=TOROIDAL_SURFACE ( 'NONE', #9043, 12.61792373059895844, 0.1249999999999980571 ) ;
#14304=ADVANCED_FACE ( 'NONE', ( #21648 ), #2090, .T. ) ;
#14310=ADVANCED_FACE ( 'NONE', ( #19178 ), #3939, .T. ) ;
#14315=CARTESIAN_POINT ( 'NONE',  ( 33.50134396954520355, 30.59164230456639544, 47.04930799450051637 ) ) ;
#14318=AXIS2_PLACEMENT_3D ( 'NONE', #22315, #32339, #19848 ) ;
#14326=DIRECTION ( 'NONE',  ( 1.000000000000000000, 0.000000000000000000, 0.000000000000000000 ) ) ;
#14335=FACE_OUTER_BOUND ( 'NONE', #139, .T. ) ;
#14337=VERTEX_POINT ( 'NONE', #31827 ) ;
#14340=FACE_OUTER_BOUND ( 'NONE', #20133, .T. ) ;
#14341=VERTEX_POINT ( 'NONE', #29207 ) ;
#14346=FACE_OUTER_BOUND ( 'NONE', #27298, .T. ) ;
#14350=ORIENTED_EDGE ( 'NONE', *, *, #3799, .F. ) ;
#14356=ADVANCED_FACE ( 'NONE', ( #9346 ), #21156, .F. ) ;
#14358=AXIS2_PLACEMENT_3D ( 'NONE', #17678, #27866, #5217 ) ;
#14361=DIRECTION ( 'NONE',  ( -1.101824276508909887E-16, 1.000000000000000000, -0.000000000000000000 ) ) ;
#14363=DIRECTION ( 'NONE',  ( -1.101824276508909887E-16, 1.000000000000000000, -0.000000000000000000 ) ) ;
#14367=DIRECTION ( 'NONE',  ( -1.000000000000000000, -1.101824276508909887E-16, 0.000000000000000000 ) ) ;
#14372=CARTESIAN_POINT ( 'NONE',  ( 21.09992658989238734, 30.71664230456641675, 47.04930799450051637 ) ) ;
#14376=DIRECTION ( 'NONE',  ( -1.224646799147353207E-16, -1.349345573449484691E-32, 1.000000000000000000 ) ) ;
#14379=DIRECTION ( 'NONE',  ( 1.000000000000000000, 0.000000000000000000, 0.000000000000000000 ) ) ;
#14381=DIRECTION ( 'NONE',  ( -1.101824276508909887E-16, 1.000000000000000000, -0.000000000000000000 ) ) ;
#14383=FACE_OUTER_BOUND ( 'NONE', #5558, .T. ) ;
#14388=EDGE_CURVE ( 'NONE', #18298, #30931, #4720, .T. ) ;
#14394=CIRCLE ( 'NONE', #21729, 12.62506659569710266 ) ;
#14395=DIRECTION ( 'NONE',  ( -1.101824276508909887E-16, 1.000000000000000000, -0.000000000000000000 ) ) ;
#14399=DIRECTION ( 'NONE',  ( -1.101824276508909887E-16, 1.000000000000000000, -0.000000000000000000 ) ) ;
#14403=ORIENTED_EDGE ( 'NONE', *, *, #21357, .F. ) ;
#14405=ORIENTED_EDGE ( 'NONE', *, *, #31431, .F. ) ;
#14408=DIRECTION ( 'NONE',  ( -1.101824276508909887E-16, 1.000000000000000000, -0.000000000000000000 ) ) ;
#14414=AXIS2_PLACEMENT_3D ( 'NONE', #19674, #9838, #5076 ) ;
#14419=DIRECTION ( 'NONE',  ( -1.101824276508909887E-16, 1.000000000000000000, -0.000000000000000000 ) ) ;
#14424=EDGE_CURVE ( 'NONE', #7900, #10115, #542, .T. ) ;
#14425=VECTOR ( 'NONE', #23144, 1000.000000000000000 ) ;
#14429=ORIENTED_EDGE ( 'NONE', *, *, #2486, .T. ) ;
#14431=DIRECTION ( 'NONE',  ( -1.101824276508909887E-16, 1.000000000000000000, -0.000000000000000000 ) ) ;
#14432=CARTESIAN_POINT ( 'NONE',  ( 21.09992658989239089, 27.71664230456639899, 47.04930799450051637 ) ) ;
#14434=EDGE_LOOP ( 'NONE', ( #14931, #24394, #16954, #22380 ) ) ;
#14437=EDGE_LOOP ( 'NONE', ( #1952, #27079, #26574, #15664 ) ) ;
#14438=AXIS2_PLACEMENT_3D ( 'NONE', #4588, #1964, #22144 ) ;
#14441=AXIS2_PLACEMENT_3D ( 'NONE', #26020, #15862, #25710 ) ;
#14443=AXIS2_PLACEMENT_3D ( 'NONE', #14819, #13729, #2338 ) ;
#14446=DIRECTION ( 'NONE',  ( -1.000000000000000000, 0.000000000000000000, 0.000000000000000000 ) ) ;
#14449=EDGE_CURVE ( 'NONE', #22635, #22128, #20607, .T. ) ;
#14471=FACE_OUTER_BOUND ( 'NONE', #28737, .T. ) ;
#14474=CARTESIAN_POINT ( 'NONE',  ( 21.09992658989238734, 38.56284415653841791, 47.04930799450051637 ) ) ;
#14475=EDGE_CURVE ( 'NONE', #15078, #13441, #24651, .T. ) ;
#14476=CIRCLE ( 'NONE', #22826, 12.62506659569710266 ) ;
#14478=FACE_OUTER_BOUND ( 'NONE', #10355, .T. ) ;
#14502=ORIENTED_EDGE ( 'NONE', *, *, #19556, .T. ) ;
#14503=DIRECTION ( 'NONE',  ( -1.101824276508909887E-16, 1.000000000000000000, -0.000000000000000000 ) ) ;
#14506=ORIENTED_EDGE ( 'NONE', *, *, #9794, .F. ) ;
#14509=DIRECTION ( 'NONE',  ( -1.224646799147353207E-16, -1.349345573449484691E-32, 1.000000000000000000 ) ) ;
#14512=ORIENTED_EDGE ( 'NONE', *, *, #29495, .T. ) ;
#14515=AXIS2_PLACEMENT_3D ( 'NONE', #7560, #12818, #29559 ) ;
#14517=FACE_OUTER_BOUND ( 'NONE', #7810, .T. ) ;
#14518=CIRCLE ( 'NONE', #20795, 12.36707279061065279 ) ;
#14519=ORIENTED_EDGE ( 'NONE', *, *, #15526, .F. ) ;
#14520=CARTESIAN_POINT ( 'NONE',  ( 33.72499318558949000, 38.56284415653841791, 47.04930799450051637 ) ) ;
#14523=VERTEX_POINT ( 'NONE', #264 ) ;
#14526=DIRECTION ( 'NONE',  ( -1.101824276508909887E-16, 1.000000000000000000, -0.000000000000000000 ) ) ;
#14527=FACE_OUTER_BOUND ( 'NONE', #29861, .T. ) ;
#14534=DIRECTION ( 'NONE',  ( 0.000000000000000000, -0.000000000000000000, -1.000000000000000000 ) ) ;
#14536=FACE_OUTER_BOUND ( 'NONE', #131, .T. ) ;
#14541=CARTESIAN_POINT ( 'NONE',  ( 8.698509210239514289, 24.84164230456639544, 47.04930799450051637 ) ) ;
#14543=DIRECTION ( 'NONE',  ( -1.101824276508909887E-16, 1.000000000000000000, -0.000000000000000000 ) ) ;
#14545=ORIENTED_EDGE ( 'NONE', *, *, #23861, .T. ) ;
#14549=AXIS2_PLACEMENT_3D ( 'NONE', #15451, #20361, #10368 ) ;
#14550=ORIENTED_EDGE ( 'NONE', *, *, #15279, .F. ) ;
#14569=CARTESIAN_POINT ( 'NONE',  ( 21.09992658989239089, 26.97145308207318948, 47.04930799450051637 ) ) ;
#14572=EDGE_CURVE ( 'NONE', #12078, #15900, #2518, .T. ) ;
#14573=ADVANCED_FACE ( 'NONE', ( #3524 ), #5999, .T. ) ;
#14589=CARTESIAN_POINT ( 'NONE',  ( 8.474859994195286461, 25.34184655352419213, 47.04930799450051637 ) ) ;
#14590=CIRCLE ( 'NONE', #13538, 0.1250000000000001110 ) ;
#14592=ORIENTED_EDGE ( 'NONE', *, *, #18687, .T. ) ;
#14593=DIRECTION ( 'NONE',  ( -1.000000000000000000, 0.000000000000000000, 0.000000000000000000 ) ) ;
#14594=ADVANCED_FACE ( 'NONE', ( #31435 ), #19252, .T. ) ;
#14599=AXIS2_PLACEMENT_3D ( 'NONE', #31355, #18215, #8861 ) ;
#14601=ORIENTED_EDGE ( 'NONE', *, *, #25394, .T. ) ;
#14603=DIRECTION ( 'NONE',  ( -1.000000000000000000, 0.000000000000000000, 0.000000000000000000 ) ) ;
#14604=AXIS2_PLACEMENT_3D ( 'NONE', #17145, #12249, #6989 ) ;
#14606=DIRECTION ( 'NONE',  ( -1.101824276508909887E-16, 1.000000000000000000, -0.000000000000000000 ) ) ;
#14608=VERTEX_POINT ( 'NONE', #749 ) ;
#14611=CIRCLE ( 'NONE', #18272, 12.36707279061065101 ) ;
#14612=DIRECTION ( 'NONE',  ( -1.224646799147353207E-16, -1.349345573449484691E-32, 1.000000000000000000 ) ) ;
#14614=DIRECTION ( 'NONE',  ( -1.224646799147353207E-16, -1.349345573449484691E-32, 1.000000000000000000 ) ) ;
#14624=CARTESIAN_POINT ( 'NONE',  ( 8.474859994195282908, 38.56284415653841791, 47.04930799450051637 ) ) ;
#14627=DIRECTION ( 'NONE',  ( -1.101824276508909887E-16, 1.000000000000000000, -0.000000000000000000 ) ) ;
#14628=AXIS2_PLACEMENT_3D ( 'NONE', #30675, #13756, #23281 ) ;
#14630=DIRECTION ( 'NONE',  ( -1.101824276508909887E-16, 1.000000000000000000, -0.000000000000000000 ) ) ;
#14631=AXIS2_PLACEMENT_3D ( 'NONE', #30050, #7561, #25116 ) ;
#14633=EDGE_CURVE ( 'NONE', #12345, #29925, #12492, .T. ) ;
#14636=ORIENTED_EDGE ( 'NONE', *, *, #2006, .F. ) ;
#14647=AXIS2_PLACEMENT_3D ( 'NONE', #2244, #12267, #20280 ) ;
#14650=CARTESIAN_POINT ( 'NONE',  ( 33.72499318558949710, 23.84184655352419213, 47.04930799450051637 ) ) ;
#14653=CARTESIAN_POINT ( 'NONE',  ( 8.823509210239544487, 27.84164230456639544, 47.04930799450051637 ) ) ;
#14656=ADVANCED_FACE ( 'NONE', ( #4666 ), #4344, .T. ) ;
#14657=ORIENTED_EDGE ( 'NONE', *, *, #17036, .T. ) ;
#14661=VECTOR ( 'NONE', #13499, 1000.000000000000000 ) ;
#14664=VERTEX_POINT ( 'NONE', #12226 ) ;
#14667=DIRECTION ( 'NONE',  ( -1.101824276508909887E-16, 1.000000000000000000, -0.000000000000000000 ) ) ;
#14668=CARTESIAN_POINT ( 'NONE',  ( 21.09992658989239089, 27.09164230456639899, 47.04930799450051637 ) ) ;
#14669=ORIENTED_EDGE ( 'NONE', *, *, #20480, .F. ) ;
#14670=ORIENTED_EDGE ( 'NONE', *, *, #2110, .F. ) ;
#14674=CARTESIAN_POINT ( 'NONE',  ( 21.09992658989239089, 23.72145308207319658, 47.04930799450051637 ) ) ;
#14676=VERTEX_POINT ( 'NONE', #29619 ) ;
#14677=ADVANCED_FACE ( 'NONE', ( #18934 ), #22216, .F. ) ;
#14682=EDGE_CURVE ( 'NONE', #27386, #27774, #10370, .T. ) ;
#14683=AXIS2_PLACEMENT_3D ( 'NONE', #16860, #14739, #9488 ) ;
#14684=AXIS2_PLACEMENT_3D ( 'NONE', #24280, #11327, #16241 ) ;
#14690=AXIS2_PLACEMENT_3D ( 'NONE', #27370, #9976, #5535 ) ;
#14695=DIRECTION ( 'NONE',  ( -1.101824276508909887E-16, 1.000000000000000000, -0.000000000000000000 ) ) ;
#14701=FACE_OUTER_BOUND ( 'NONE', #5928, .T. ) ;
#14704=ORIENTED_EDGE ( 'NONE', *, *, #11365, .T. ) ;
#14707=DIRECTION ( 'NONE',  ( -1.101824276508909887E-16, 1.000000000000000000, -0.000000000000000000 ) ) ;
#14708=AXIS2_PLACEMENT_3D ( 'NONE', #10946, #11585, #8955 ) ;
#14712=AXIS2_PLACEMENT_3D ( 'NONE', #8713, #23651, #11493 ) ;
#14714=TOROIDAL_SURFACE ( 'NONE', #24660, 12.40141737965280555, 0.1250000000000006939 ) ;
#14721=CIRCLE ( 'NONE', #19943, 0.1250000000000001110 ) ;
#14723=EDGE_LOOP ( 'NONE', ( #17657, #20517, #4815, #19791 ) ) ;
#14728=CARTESIAN_POINT ( 'NONE',  ( 8.474859994195286461, 25.34143805560860940, 47.04930799450051637 ) ) ;
#14730=DIRECTION ( 'NONE',  ( -1.000000000000000000, 0.000000000000000000, 0.000000000000000000 ) ) ;
#14734=ORIENTED_EDGE ( 'NONE', *, *, #12985, .T. ) ;
#14736=ORIENTED_EDGE ( 'NONE', *, *, #26081, .F. ) ;
#14739=DIRECTION ( 'NONE',  ( -1.101824276508909887E-16, 1.000000000000000000, -0.000000000000000000 ) ) ;
#14743=SHAPE_REPRESENTATION ( 'Coil', ( #8172 ), #331 ) ;
#14744=CARTESIAN_POINT ( 'NONE',  ( 33.72499318558949000, 38.56284415653841791, 47.04930799450051637 ) ) ;
#14746=EDGE_LOOP ( 'NONE', ( #23171, #29752, #31997, #14278 ) ) ;
#14749=DIRECTION ( 'NONE',  ( -1.101824276508909887E-16, 1.000000000000000000, -0.000000000000000000 ) ) ;
#14750=ORIENTED_EDGE ( 'NONE', *, *, #1207, .T. ) ;
#14755=CARTESIAN_POINT ( 'NONE',  ( 8.732853799281718565, 31.22145308207317171, 47.04930799450051637 ) ) ;
#14757=TOROIDAL_SURFACE ( 'NONE', #22076, 12.40141737965286239, 0.1250000000000005551 ) ;
#14759=EDGE_CURVE ( 'NONE', #22795, #20651, #15106, .T. ) ;
#14760=ADVANCED_FACE ( 'NONE', ( #10406 ), #4834, .T. ) ;
#14764=EDGE_CURVE ( 'NONE', #15368, #16515, #22938, .T. ) ;
#14768=ORIENTED_EDGE ( 'NONE', *, *, #13066, .F. ) ;
#14771=CARTESIAN_POINT ( 'NONE',  ( 33.71785032049100295, 29.96664230456641675, 47.04930799450051637 ) ) ;
#14774=ORIENTED_EDGE ( 'NONE', *, *, #23515, .T. ) ;
#14779=DIRECTION ( 'NONE',  ( -1.101824276508909887E-16, 1.000000000000000000, -0.000000000000000000 ) ) ;
#14785=ORIENTED_EDGE ( 'NONE', *, *, #894, .F. ) ;
#14789=DIRECTION ( 'NONE',  ( -1.000000000000000000, 0.000000000000000000, 0.000000000000000000 ) ) ;
#14790=VERTEX_POINT ( 'NONE', #7296 ) ;
#14792=DIRECTION ( 'NONE',  ( 1.000000000000000000, 0.000000000000000000, 0.000000000000000000 ) ) ;
#14796=EDGE_CURVE ( 'NONE', #14341, #22032, #17464, .T. ) ;
#14799=VECTOR ( 'NONE', #12021, 1000.000000000000000 ) ;
#14800=VECTOR ( 'NONE', #6574, 1000.000000000000000 ) ;
#14808=DIRECTION ( 'NONE',  ( -1.000000000000000000, -1.101824276508909887E-16, 0.000000000000000000 ) ) ;
#14810=DIRECTION ( 'NONE',  ( 0.000000000000000000, -0.000000000000000000, -1.000000000000000000 ) ) ;
#14811=CARTESIAN_POINT ( 'NONE',  ( 21.09992658989239089, 27.84164230456639544, 47.04930799450051637 ) ) ;
#14817=CIRCLE ( 'NONE', #4859, 12.62506659569710266 ) ;
#14819=CARTESIAN_POINT ( 'NONE',  ( 21.09992658989238734, 38.56284415653841791, 47.04930799450051637 ) ) ;
#14821=DIRECTION ( 'NONE',  ( -1.000000000000000000, 0.000000000000000000, 0.000000000000000000 ) ) ;
#14824=LINE ( 'NONE', #204, #28601 ) ;
#14826=TOROIDAL_SURFACE ( 'NONE', #9570, 12.61792373059891403, 0.1250000000000023315 ) ;
#14827=EDGE_CURVE ( 'NONE', #12384, #29330, #3543, .T. ) ;
#14831=CIRCLE ( 'NONE', #12755, 12.27641737965282154 ) ;
#14834=DIRECTION ( 'NONE',  ( -1.000000000000000000, 0.000000000000000000, 0.000000000000000000 ) ) ;
#14842=DIRECTION ( 'NONE',  ( -1.101824276508909887E-16, 1.000000000000000000, -0.000000000000000000 ) ) ;
#14845=VERTEX_POINT ( 'NONE', #25502 ) ;
#14851=DIRECTION ( 'NONE',  ( -1.000000000000000000, 0.000000000000000000, 0.000000000000000000 ) ) ;
#14854=ORIENTED_EDGE ( 'NONE', *, *, #17331, .F. ) ;
#14856=EDGE_CURVE ( 'NONE', #17323, #104, #381, .T. ) ;
#14857=CARTESIAN_POINT ( 'NONE',  ( 33.46699938050302592, 31.72145308207317882, 47.04930799450050927 ) ) ;
#14861=CARTESIAN_POINT ( 'NONE',  ( 21.09992658989239089, 24.84164230456639544, 47.04930799450051637 ) ) ;
#14868=DIRECTION ( 'NONE',  ( -1.101824276508909887E-16, 1.000000000000000000, -0.000000000000000000 ) ) ;
#14871=ORIENTED_EDGE ( 'NONE', *, *, #3221, .T. ) ;
#14872=FACE_OUTER_BOUND ( 'NONE', #23304, .T. ) ;
#14873=ADVANCED_FACE ( 'NONE', ( #17946 ), #19790, .T. ) ;
#14874=DIRECTION ( 'NONE',  ( 1.000000000000000000, 0.000000000000000000, 0.000000000000000000 ) ) ;
#14879=CIRCLE ( 'NONE', #14358, 12.52247886585643677 ) ;
#14880=ORIENTED_EDGE ( 'NONE', *, *, #7310, .F. ) ;
#14889=DIRECTION ( 'NONE',  ( -1.000000000000000000, 0.000000000000000000, 0.000000000000000000 ) ) ;
#14892=DIRECTION ( 'NONE',  ( -1.101824276508909887E-16, 1.000000000000000000, -0.000000000000000000 ) ) ;
#14898=ORIENTED_EDGE ( 'NONE', *, *, #6214, .F. ) ;
#14900=CARTESIAN_POINT ( 'NONE',  ( 21.09992658989239089, 29.34164230456639899, 47.04930799450051637 ) ) ;
#14907=CYLINDRICAL_SURFACE ( 'NONE', #6477, 12.36707279061065101 ) ;
#14910=DIRECTION ( 'NONE',  ( -1.101824276508909887E-16, 1.000000000000000000, -0.000000000000000000 ) ) ;
#14911=ORIENTED_EDGE ( 'NONE', *, *, #16556, .F. ) ;
#14914=EDGE_LOOP ( 'NONE', ( #3776, #5033, #575, #1325 ) ) ;
#14917=DIRECTION ( 'NONE',  ( -1.000000000000000000, -1.101824276508909887E-16, 0.000000000000000000 ) ) ;
#14918=TOROIDAL_SURFACE ( 'NONE', #6513, 12.40141737965281621, 0.1249999999999985428 ) ;
#14920=TOROIDAL_SURFACE ( 'NONE', #11254, 12.40141737965284996, 0.1250000000000002776 ) ;
#14922=ORIENTED_EDGE ( 'NONE', *, *, #7352, .T. ) ;
#14923=DIRECTION ( 'NONE',  ( -1.000000000000000000, -1.101824276508909887E-16, 0.000000000000000000 ) ) ;
#14924=EDGE_LOOP ( 'NONE', ( #32012, #5784, #19688, #29061 ) ) ;
#14927=CARTESIAN_POINT ( 'NONE',  ( 21.09992658989239089, 28.21183152705961206, 47.04930799450051637 ) ) ;
#14930=VERTEX_POINT ( 'NONE', #16283 ) ;
#14931=ORIENTED_EDGE ( 'NONE', *, *, #27468, .F. ) ;
#14932=CIRCLE ( 'NONE', #8657, 0.1250000000000001110 ) ;
#14935=ORIENTED_EDGE ( 'NONE', *, *, #17037, .F. ) ;
#14938=DIRECTION ( 'NONE',  ( -1.000000000000000000, -1.101824276508910010E-16, 0.000000000000000000 ) ) ;
#14940=DIRECTION ( 'NONE',  ( -1.101824276508909887E-16, 1.000000000000000000, -0.000000000000000000 ) ) ;
#14946=FACE_OUTER_BOUND ( 'NONE', #25065, .T. ) ;
#14949=DIRECTION ( 'NONE',  ( -1.101824276508909887E-16, 1.000000000000000000, -0.000000000000000000 ) ) ;
#14954=ORIENTED_EDGE ( 'NONE', *, *, #4854, .F. ) ;
#14960=AXIS2_PLACEMENT_3D ( 'NONE', #2049, #20253, #25025 ) ;
#14963=VERTEX_POINT ( 'NONE', #10577 ) ;
#14964=ORIENTED_EDGE ( 'NONE', *, *, #18733, .F. ) ;
#14966=DIRECTION ( 'NONE',  ( -1.101824276508909887E-16, 1.000000000000000000, -0.000000000000000000 ) ) ;
#14968=ORIENTED_EDGE ( 'NONE', *, *, #20030, .F. ) ;
#14974=DIRECTION ( 'NONE',  ( -1.101824276508909887E-16, 1.000000000000000000, -0.000000000000000000 ) ) ;
#14978=AXIS2_PLACEMENT_3D ( 'NONE', #4709, #7505, #27521 ) ;
#14982=VERTEX_POINT ( 'NONE', #28600 ) ;
#14983=CARTESIAN_POINT ( 'NONE',  ( 21.09992658989238734, 30.84184655352422411, 47.04930799450051637 ) ) ;
#14984=VECTOR ( 'NONE', #18908, 1000.000000000000000 ) ;
#14985=CARTESIAN_POINT ( 'NONE',  ( 21.09992658989239089, 30.09164230456639544, 47.04930799450051637 ) ) ;
#14988=DIRECTION ( 'NONE',  ( -1.101824276508909887E-16, 1.000000000000000000, -0.000000000000000000 ) ) ;
#14990=ADVANCED_FACE ( 'NONE', ( #867 ), #10891, .T. ) ;
#14992=DIRECTION ( 'NONE',  ( -1.101824276508909887E-16, 1.000000000000000000, -0.000000000000000000 ) ) ;
#15002=CARTESIAN_POINT ( 'NONE',  ( 21.09992658989239089, 28.34164230456639544, 47.04930799450051637 ) ) ;
#15005=ORIENTED_EDGE ( 'NONE', *, *, #13987, .F. ) ;
#15006=DIRECTION ( 'NONE',  ( -1.000000000000000000, -1.101824276508909887E-16, 0.000000000000000000 ) ) ;
#15007=AXIS2_PLACEMENT_3D ( 'NONE', #27242, #7065, #27080 ) ;
#15008=PRODUCT_DEFINITION_FORMATION_WITH_SPECIFIED_SOURCE ( 'ANY', '', #9564, .NOT_KNOWN. ) ;
#15009=ORIENTED_EDGE ( 'NONE', *, *, #9341, .T. ) ;
#15010=CYLINDRICAL_SURFACE ( 'NONE', #17622, 12.62506659569710266 ) ;
#15011=DIRECTION ( 'NONE',  ( -1.000000000000000000, 0.000000000000000000, 0.000000000000000000 ) ) ;
#15013=ADVANCED_FACE ( 'NONE', ( #11210 ), #28761, .F. ) ;
#15016=CARTESIAN_POINT ( 'NONE',  ( 21.09992658989238734, 32.59164230456639899, 47.04930799450051637 ) ) ;
#15018=FACE_OUTER_BOUND ( 'NONE', #19515, .T. ) ;
#15020=DIRECTION ( 'NONE',  ( -1.000000000000000000, -1.101824276508909887E-16, 0.000000000000000000 ) ) ;
#15022=VERTEX_POINT ( 'NONE', #3976 ) ;
#15026=CARTESIAN_POINT ( 'NONE',  ( 8.732853799281729223, 27.97145308207318237, 47.04930799450051637 ) ) ;
#15031=ORIENTED_EDGE ( 'NONE', *, *, #5362, .F. ) ;
#15032=EDGE_CURVE ( 'NONE', #14523, #4901, #16928, .T. ) ;
#15033=DIRECTION ( 'NONE',  ( -1.101824276508909887E-16, 1.000000000000000000, -0.000000000000000000 ) ) ;
#15034=CIRCLE ( 'NONE', #29719, 0.1250000000000001110 ) ;
#15036=ORIENTED_EDGE ( 'NONE', *, *, #17149, .T. ) ;
#15042=EDGE_CURVE ( 'NONE', #18493, #21006, #30854, .T. ) ;
#15050=DIRECTION ( 'NONE',  ( -1.000000000000000000, -1.101824276508909887E-16, 0.000000000000000000 ) ) ;
#15053=ORIENTED_EDGE ( 'NONE', *, *, #6487, .T. ) ;
#15063=DIRECTION ( 'NONE',  ( -1.101824276508909887E-16, 1.000000000000000000, -0.000000000000000000 ) ) ;
#15067=DIRECTION ( 'NONE',  ( 0.000000000000000000, -0.000000000000000000, -1.000000000000000000 ) ) ;
#15074=ORIENTED_EDGE ( 'NONE', *, *, #22662, .T. ) ;
#15076=ORIENTED_EDGE ( 'NONE', *, *, #16960, .T. ) ;
#15078=VERTEX_POINT ( 'NONE', #31558 ) ;
#15079=AXIS2_PLACEMENT_3D ( 'NONE', #25195, #7966, #3015 ) ;
#15086=DIRECTION ( 'NONE',  ( -1.101824276508909887E-16, 1.000000000000000000, -0.000000000000000000 ) ) ;
#15090=ORIENTED_EDGE ( 'NONE', *, *, #262, .F. ) ;
#15095=ORIENTED_EDGE ( 'NONE', *, *, #28088, .F. ) ;
#15098=DIRECTION ( 'NONE',  ( -1.000000000000000000, 0.000000000000000000, 0.000000000000000000 ) ) ;
#15103=ORIENTED_EDGE ( 'NONE', *, *, #5121, .T. ) ;
#15104=CARTESIAN_POINT ( 'NONE',  ( 21.09992658989239089, 26.59184655352419568, 47.04930799450051637 ) ) ;
#15106=CIRCLE ( 'NONE', #26616, 12.62506659569710266 ) ;
#15108=ORIENTED_EDGE ( 'NONE', *, *, #18204, .F. ) ;
#15110=ORIENTED_EDGE ( 'NONE', *, *, #19378, .F. ) ;
#15114=CIRCLE ( 'NONE', #32409, 12.27641737965283397 ) ;
#15118=CIRCLE ( 'NONE', #26092, 0.1250000000000001110 ) ;
#15120=AXIS2_PLACEMENT_3D ( 'NONE', #92, #16829, #32429 ) ;
#15123=DIRECTION ( 'NONE',  ( -1.101824276508909887E-16, 1.000000000000000000, -0.000000000000000000 ) ) ;
#15125=ADVANCED_FACE ( 'NONE', ( #31394 ), #30309, .T. ) ;
#15127=ORIENTED_EDGE ( 'NONE', *, *, #26931, .F. ) ;
#15128=EDGE_CURVE ( 'NONE', #18493, #22536, #16670, .T. ) ;
#15130=DIRECTION ( 'NONE',  ( 1.000000000000000000, 0.000000000000000000, 0.000000000000000000 ) ) ;
#15134=DIRECTION ( 'NONE',  ( -1.101824276508909887E-16, 1.000000000000000000, -0.000000000000000000 ) ) ;
#15143=CIRCLE ( 'NONE', #28762, 0.1250000000000001110 ) ;
#15145=DIRECTION ( 'NONE',  ( -1.000000000000000000, -1.101824276508909887E-16, 0.000000000000000000 ) ) ;
#15146=AXIS2_PLACEMENT_3D ( 'NONE', #18202, #8695, #11471 ) ;
#15158=DIRECTION ( 'NONE',  ( -1.000000000000000000, 0.000000000000000000, 0.000000000000000000 ) ) ;
#15175=CIRCLE ( 'NONE', #30922, 12.62506659569710266 ) ;
#15180=DIRECTION ( 'NONE',  ( 0.000000000000000000, -0.000000000000000000, -1.000000000000000000 ) ) ;
#15185=CARTESIAN_POINT ( 'NONE',  ( 33.46699938050304723, 25.97145308207318593, 47.04930799450050927 ) ) ;
#15187=VERTEX_POINT ( 'NONE', #22008 ) ;
#15190=CIRCLE ( 'NONE', #23022, 12.62506659569710266 ) ;
#15193=ORIENTED_EDGE ( 'NONE', *, *, #32403, .F. ) ;
#15194=FACE_OUTER_BOUND ( 'NONE', #16908, .T. ) ;
#15196=EDGE_CURVE ( 'NONE', #15022, #19672, #29274, .T. ) ;
#15197=AXIS2_PLACEMENT_3D ( 'NONE', #20551, #28588, #30580 ) ;
#15199=VERTEX_POINT ( 'NONE', #6444 ) ;
#15200=AXIS2_PLACEMENT_3D ( 'NONE', #31667, #26731, #22290 ) ;
#15202=DIRECTION ( 'NONE',  ( -1.101824276508909887E-16, 1.000000000000000000, -0.000000000000000000 ) ) ;
#15203=CARTESIAN_POINT ( 'NONE',  ( 21.09992658989238734, 31.96183152705962272, 47.04930799450051637 ) ) ;
#15206=EDGE_LOOP ( 'NONE', ( #29707, #18926, #26484, #25951 ) ) ;
#15211=DIRECTION ( 'NONE',  ( -1.000000000000000000, 0.000000000000000000, 0.000000000000000000 ) ) ;
#15217=VERTEX_POINT ( 'NONE', #7911 ) ;
#15221=DIRECTION ( 'NONE',  ( 0.000000000000000000, -0.000000000000000000, -1.000000000000000000 ) ) ;
#15230=AXIS2_PLACEMENT_3D ( 'NONE', #28473, #21065, #4489 ) ;
#15238=CARTESIAN_POINT ( 'NONE',  ( 8.474859994195281132, 31.09184655352422411, 47.04930799450051637 ) ) ;
#15239=EDGE_CURVE ( 'NONE', #16515, #4901, #27160, .T. ) ;
#15240=EDGE_CURVE ( 'NONE', #24311, #9505, #23508, .T. ) ;
#15243=CIRCLE ( 'NONE', #23598, 12.62506659569710266 ) ;
#15253=ORIENTED_EDGE ( 'NONE', *, *, #22624, .T. ) ;
#15256=TOROIDAL_SURFACE ( 'NONE', #5313, 12.40141737965288904, 0.1249999999999998612 ) ;
#15257=ORIENTED_EDGE ( 'NONE', *, *, #12349, .T. ) ;
#15259=FACE_OUTER_BOUND ( 'NONE', #3277, .T. ) ;
#15260=CARTESIAN_POINT ( 'NONE',  ( 21.09992658989238734, 30.84143805560860585, 47.04930799450051637 ) ) ;
#15265=ORIENTED_EDGE ( 'NONE', *, *, #4625, .F. ) ;
#15267=CYLINDRICAL_SURFACE ( 'NONE', #16636, 12.36707279061065101 ) ;
#15270=ORIENTED_EDGE ( 'NONE', *, *, #17488, .F. ) ;
#15276=DIRECTION ( 'NONE',  ( -1.000000000000000000, 0.000000000000000000, 0.000000000000000000 ) ) ;
#15279=EDGE_CURVE ( 'NONE', #10069, #22139, #14590, .T. ) ;
#15287=VECTOR ( 'NONE', #6167, 1000.000000000000000 ) ;
#15305=CYLINDRICAL_SURFACE ( 'NONE', #26497, 12.36707279061065279 ) ;
#15307=CARTESIAN_POINT ( 'NONE',  ( 33.71785032049132980, 29.21664230456640254, 47.04930799450051637 ) ) ;
#15312=DIRECTION ( 'NONE',  ( -1.000000000000000000, -1.101824276508910010E-16, 0.000000000000000000 ) ) ;
#15313=CARTESIAN_POINT ( 'NONE',  ( 21.09992658989238734, 38.56284415653841791, 47.04930799450051637 ) ) ;
#15319=DIRECTION ( 'NONE',  ( -1.000000000000000000, 0.000000000000000000, 0.000000000000000000 ) ) ;
#15321=CARTESIAN_POINT ( 'NONE',  ( 21.09992658989238734, 31.97145308207317171, 47.04930799450051637 ) ) ;
#15322=AXIS2_PLACEMENT_3D ( 'NONE', #3503, #5984, #3350 ) ;
#15326=CIRCLE ( 'NONE', #18974, 12.62506659569710266 ) ;
#15331=CIRCLE ( 'NONE', #25293, 0.1250000000000001110 ) ;
#15334=DIRECTION ( 'NONE',  ( -1.000000000000000000, 0.000000000000000000, 0.000000000000000000 ) ) ;
#15337=CARTESIAN_POINT ( 'NONE',  ( 33.72499318558949000, 38.56284415653841791, 47.04930799450051637 ) ) ;
#15346=CARTESIAN_POINT ( 'NONE',  ( 21.09992658989239089, 24.46183152705960140, 47.04930799450051637 ) ) ;
#15349=DIRECTION ( 'NONE',  ( 0.000000000000000000, -0.000000000000000000, -1.000000000000000000 ) ) ;
#15352=DIRECTION ( 'NONE',  ( 0.000000000000000000, -0.000000000000000000, -1.000000000000000000 ) ) ;
#15364=AXIS2_PLACEMENT_3D ( 'NONE', #2717, #15352, #30461 ) ;
#15366=FACE_OUTER_BOUND ( 'NONE', #1702, .T. ) ;
#15368=VERTEX_POINT ( 'NONE', #21161 ) ;
#15372=CARTESIAN_POINT ( 'NONE',  ( 21.09992658989238734, 31.59164230456639544, 47.04930799450051637 ) ) ;
#15373=AXIS2_PLACEMENT_3D ( 'NONE', #16523, #21768, #16362 ) ;
#15375=EDGE_CURVE ( 'NONE', #14267, #4827, #5916, .T. ) ;
#15376=ORIENTED_EDGE ( 'NONE', *, *, #31944, .F. ) ;
#15385=DIRECTION ( 'NONE',  ( 0.000000000000000000, -0.000000000000000000, -1.000000000000000000 ) ) ;
#15388=AXIS2_PLACEMENT_3D ( 'NONE', #2266, #7185, #2096 ) ;
#15392=CARTESIAN_POINT ( 'NONE',  ( 21.09992658989239089, 29.47145308207317882, 47.04930799450051637 ) ) ;
#15395=ADVANCED_FACE ( 'NONE', ( #20849 ), #5444, .T. ) ;
#15402=AXIS2_PLACEMENT_3D ( 'NONE', #18789, #21098, #3708 ) ;
#15404=AXIS2_PLACEMENT_3D ( 'NONE', #28749, #21679, #19207 ) ;
#15405=ORIENTED_EDGE ( 'NONE', *, *, #11937, .F. ) ;
#15412=EDGE_LOOP ( 'NONE', ( #7716, #28635, #6098, #17558 ) ) ;
#15413=EDGE_LOOP ( 'NONE', ( #1033, #21416, #5825, #8587 ) ) ;
#15415=EDGE_CURVE ( 'NONE', #1311, #13866, #18696, .T. ) ;
#15418=DIRECTION ( 'NONE',  ( -1.000000000000000000, 0.000000000000000000, 0.000000000000000000 ) ) ;
#15421=CARTESIAN_POINT ( 'NONE',  ( 8.474859994195281132, 38.56284415653841791, 47.04930799450051637 ) ) ;
#15425=DIRECTION ( 'NONE',  ( -1.000000000000000000, 0.000000000000000000, 0.000000000000000000 ) ) ;
#15429=CYLINDRICAL_SURFACE ( 'NONE', #9926, 12.62506659569710266 ) ;
#15433=VERTEX_POINT ( 'NONE', #8548 ) ;
#15435=CIRCLE ( 'NONE', #21184, 12.36707279061065101 ) ;
#15444=EDGE_CURVE ( 'NONE', #14982, #21567, #21104, .T. ) ;
#15449=DIRECTION ( 'NONE',  ( 0.000000000000000000, -0.000000000000000000, -1.000000000000000000 ) ) ;
#15451=CARTESIAN_POINT ( 'NONE',  ( 21.09992658989238734, 38.56284415653841791, 47.04930799450051637 ) ) ;
#15461=ORIENTED_EDGE ( 'NONE', *, *, #13826, .F. ) ;
#15463=FACE_OUTER_BOUND ( 'NONE', #27676, .T. ) ;
#15464=DIRECTION ( 'NONE',  ( -1.101824276508909887E-16, 1.000000000000000000, -0.000000000000000000 ) ) ;
#15465=CIRCLE ( 'NONE', #19618, 0.1250000000000001110 ) ;
#15469=VERTEX_POINT ( 'NONE', #8074 ) ;
#15470=ORIENTED_EDGE ( 'NONE', *, *, #15444, .T. ) ;
#15474=EDGE_CURVE ( 'NONE', #15199, #20144, #18978, .T. ) ;
#15482=CARTESIAN_POINT ( 'NONE',  ( 21.09992658989239089, 26.34164230456639899, 47.04930799450051637 ) ) ;
#15485=AXIS2_PLACEMENT_3D ( 'NONE', #635, #20492, #20318 ) ;
#15488=VECTOR ( 'NONE', #24949, 1000.000000000000000 ) ;
#15489=AXIS2_PLACEMENT_3D ( 'NONE', #21698, #24325, #4475 ) ;
#15491=ADVANCED_FACE ( 'NONE', ( #9354 ), #11979, .T. ) ;
#15494=CIRCLE ( 'NONE', #23871, 12.27641737965280200 ) ;
#15502=CARTESIAN_POINT ( 'NONE',  ( 33.50134396954528171, 23.59164230456639544, 47.04930799450051637 ) ) ;
#15503=DIRECTION ( 'NONE',  ( -1.101824276508909887E-16, 1.000000000000000000, -0.000000000000000000 ) ) ;
#15504=DIRECTION ( 'NONE',  ( -1.000000000000000000, 0.000000000000000000, 0.000000000000000000 ) ) ;
#15505=VECTOR ( 'NONE', #23636, 1000.000000000000000 ) ;
#15508=DIRECTION ( 'NONE',  ( -1.000000000000000000, 0.000000000000000000, 0.000000000000000000 ) ) ;
#15515=ORIENTED_EDGE ( 'NONE', *, *, #16960, .F. ) ;
#15525=EDGE_LOOP ( 'NONE', ( #15031, #4703, #30731, #13522 ) ) ;
#15526=EDGE_CURVE ( 'NONE', #8522, #5457, #21608, .T. ) ;
#15528=CARTESIAN_POINT ( 'NONE',  ( 33.50134396954527460, 24.34164230456639544, 47.04930799450051637 ) ) ;
#15529=DIRECTION ( 'NONE',  ( -1.101824276508909887E-16, 1.000000000000000000, -0.000000000000000000 ) ) ;
#15531=ORIENTED_EDGE ( 'NONE', *, *, #29086, .T. ) ;
#15535=AXIS2_PLACEMENT_3D ( 'NONE', #1775, #11794, #17184 ) ;
#15538=LINE ( 'NONE', #28181, #12142 ) ;
#15539=CARTESIAN_POINT ( 'NONE',  ( 8.732853799281738105, 26.46183152705960140, 47.04930799450051637 ) ) ;
#15542=LINE ( 'NONE', #25553, #18370 ) ;
#15547=AXIS2_PLACEMENT_3D ( 'NONE', #15321, #10397, #20394 ) ;
#15551=CYLINDRICAL_SURFACE ( 'NONE', #25158, 12.36707279061065101 ) ;
#15552=EDGE_LOOP ( 'NONE', ( #11108, #18799, #20869, #22986 ) ) ;
#15554=ORIENTED_EDGE ( 'NONE', *, *, #24678, .T. ) ;
#15555=CARTESIAN_POINT ( 'NONE',  ( 21.09992658989238734, 32.09164230456639899, 47.04930799450051637 ) ) ;
#15557=VERTEX_POINT ( 'NONE', #29375 ) ;
#15558=EDGE_CURVE ( 'NONE', #17658, #1940, #6893, .T. ) ;
#15559=EDGE_CURVE ( 'NONE', #11505, #17692, #25312, .T. ) ;
#15560=DIRECTION ( 'NONE',  ( -1.000000000000000000, 0.000000000000000000, 0.000000000000000000 ) ) ;
#15564=EDGE_CURVE ( 'NONE', #17073, #5065, #11164, .T. ) ;
#15572=DIRECTION ( 'NONE',  ( -1.101824276508909887E-16, 1.000000000000000000, -0.000000000000000000 ) ) ;
#15578=CARTESIAN_POINT ( 'NONE',  ( 21.09992658989239089, 23.96664230456639899, 47.04930799450051637 ) ) ;
#15582=CARTESIAN_POINT ( 'NONE',  ( 21.09992658989238734, 31.72145308207317171, 47.04930799450051637 ) ) ;
#15596=ORIENTED_EDGE ( 'NONE', *, *, #15558, .F. ) ;
#15598=CIRCLE ( 'NONE', #27671, 0.1250000000000001110 ) ;
#15608=CARTESIAN_POINT ( 'NONE',  ( 21.09992658989238734, 32.54735957529758394, 47.04930799450051637 ) ) ;
#15615=DIRECTION ( 'NONE',  ( -1.101824276508909887E-16, 1.000000000000000000, -0.000000000000000000 ) ) ;
#15617=ORIENTED_EDGE ( 'NONE', *, *, #2994, .T. ) ;
#15618=DIRECTION ( 'NONE',  ( -1.101824276508909887E-16, 1.000000000000000000, -0.000000000000000000 ) ) ;
#15621=ORIENTED_EDGE ( 'NONE', *, *, #24805, .T. ) ;
#15623=DIRECTION ( 'NONE',  ( -1.000000000000000000, -1.101824276508909887E-16, 0.000000000000000000 ) ) ;
#15625=AXIS2_PLACEMENT_3D ( 'NONE', #6006, #18621, #28332 ) ;
#15635=EDGE_CURVE ( 'NONE', #27727, #24189, #7493, .T. ) ;
#15638=ORIENTED_EDGE ( 'NONE', *, *, #2716, .T. ) ;
#15644=CIRCLE ( 'NONE', #29283, 0.1249999999999983763 ) ;
#15645=ORIENTED_EDGE ( 'NONE', *, *, #10847, .F. ) ;
#15654=DIRECTION ( 'NONE',  ( -1.000000000000000000, 0.000000000000000000, 0.000000000000000000 ) ) ;
#15656=DIRECTION ( 'NONE',  ( -1.101824276508909887E-16, 1.000000000000000000, -0.000000000000000000 ) ) ;
#15662=CARTESIAN_POINT ( 'NONE',  ( 8.474859994195286461, 28.84143805560861296, 47.04930799450051637 ) ) ;
#15663=EDGE_CURVE ( 'NONE', #17323, #31343, #30024, .T. ) ;
#15664=ORIENTED_EDGE ( 'NONE', *, *, #15718, .F. ) ;
#15671=DIRECTION ( 'NONE',  ( -1.000000000000000000, 0.000000000000000000, 0.000000000000000000 ) ) ;
#15672=ORIENTED_EDGE ( 'NONE', *, *, #16033, .T. ) ;
#15674=ADVANCED_FACE ( 'NONE', ( #8510 ), #20055, .T. ) ;
#15675=ORIENTED_EDGE ( 'NONE', *, *, #6595, .F. ) ;
#15679=AXIS2_PLACEMENT_3D ( 'NONE', #5584, #30702, #10192 ) ;
#15682=LINE ( 'NONE', #3203, #18744 ) ;
#15683=ORIENTED_EDGE ( 'NONE', *, *, #22671, .T. ) ;
#15685=VERTEX_POINT ( 'NONE', #7870 ) ;
#15687=DIRECTION ( 'NONE',  ( -1.000000000000000000, 0.000000000000000000, 0.000000000000000000 ) ) ;
#15688=CARTESIAN_POINT ( 'NONE',  ( 21.09992658989239089, 27.34164230456639544, 47.04930799450051637 ) ) ;
#15689=DIRECTION ( 'NONE',  ( 0.000000000000000000, -0.000000000000000000, -1.000000000000000000 ) ) ;
#15691=LINE ( 'NONE', #31445, #18060 ) ;
#15695=CIRCLE ( 'NONE', #31938, 12.62506659569710266 ) ;
#15696=VERTEX_POINT ( 'NONE', #13291 ) ;
#15699=CARTESIAN_POINT ( 'NONE',  ( 21.09992658989239089, 29.22145308207318237, 47.04930799450051637 ) ) ;
#15700=FACE_OUTER_BOUND ( 'NONE', #26891, .T. ) ;
#15704=FACE_OUTER_BOUND ( 'NONE', #8835, .T. ) ;
#15705=ADVANCED_FACE ( 'NONE', ( #25745 ), #5564, .T. ) ;
#15710=AXIS2_PLACEMENT_3D ( 'NONE', #25840, #25685, #20754 ) ;
#15718=EDGE_CURVE ( 'NONE', #1319, #1121, #20319, .T. ) ;
#15719=EDGE_CURVE ( 'NONE', #14982, #11505, #27422, .T. ) ;
#15720=CIRCLE ( 'NONE', #1556, 12.62506659569710266 ) ;
#15725=TOROIDAL_SURFACE ( 'NONE', #6281, 12.40141737965284641, 0.1249999999999995698 ) ;
#15732=TOROIDAL_SURFACE ( 'NONE', #9509, 12.61792373059894778, 0.1249999999999986539 ) ;
#15735=ORIENTED_EDGE ( 'NONE', *, *, #13182, .T. ) ;
#15736=ORIENTED_EDGE ( 'NONE', *, *, #21228, .F. ) ;
#15741=CARTESIAN_POINT ( 'NONE',  ( 21.09992658989239089, 23.97145308207319658, 47.04930799450051637 ) ) ;
#15746=AXIS2_PLACEMENT_3D ( 'NONE', #8903, #18905, #2495 ) ;
#15750=ORIENTED_EDGE ( 'NONE', *, *, #3746, .F. ) ;
#15754=ORIENTED_EDGE ( 'NONE', *, *, #24694, .T. ) ;
#15758=TOROIDAL_SURFACE ( 'NONE', #13658, 12.61792373059897798, 0.1249999999999968636 ) ;
#15759=EDGE_CURVE ( 'NONE', #7622, #27343, #2928, .T. ) ;
#15767=CARTESIAN_POINT ( 'NONE',  ( 21.09992658989239089, 29.21664230456640254, 47.04930799450051637 ) ) ;
#15768=DIRECTION ( 'NONE',  ( -1.000000000000000000, 0.000000000000000000, 0.000000000000000000 ) ) ;
#15770=ORIENTED_EDGE ( 'NONE', *, *, #1538, .F. ) ;
#15771=DIRECTION ( 'NONE',  ( -1.101824276508909887E-16, 1.000000000000000000, -0.000000000000000000 ) ) ;
#15774=DIRECTION ( 'NONE',  ( -1.101824276508909887E-16, 1.000000000000000000, -0.000000000000000000 ) ) ;
#15777=CARTESIAN_POINT ( 'NONE',  ( 8.823509210239569356, 30.84164230456639544, 47.04930799450051637 ) ) ;
#15783=FILL_AREA_STYLE_COLOUR ( '', #27588 ) ;
#15785=ORIENTED_EDGE ( 'NONE', *, *, #11243, .F. ) ;
#15786=ADVANCED_FACE ( 'NONE', ( #23118 ), #13806, .T. ) ;
#15791=ORIENTED_EDGE ( 'NONE', *, *, #21961, .T. ) ;
#15793=DIRECTION ( 'NONE',  ( -1.000000000000000000, 0.000000000000000000, 0.000000000000000000 ) ) ;
#15798=AXIS2_PLACEMENT_3D ( 'NONE', #2174, #4308, #12188 ) ;
#15803=ORIENTED_EDGE ( 'NONE', *, *, #30, .F. ) ;
#15813=DIRECTION ( 'NONE',  ( -1.000000000000000000, -1.101824276508909764E-16, 0.000000000000000000 ) ) ;
#15821=EDGE_CURVE ( 'NONE', #25773, #30925, #31616, .T. ) ;
#15824=EDGE_CURVE ( 'NONE', #12417, #12816, #21116, .T. ) ;
#15835=EDGE_LOOP ( 'NONE', ( #21951, #10135, #14429, #31068 ) ) ;
#15837=CARTESIAN_POINT ( 'NONE',  ( 21.09992658989239089, 27.59143805560860940, 47.04930799450051637 ) ) ;
#15844=AXIS2_PLACEMENT_3D ( 'NONE', #29796, #14534, #11744 ) ;
#15847=CIRCLE ( 'NONE', #31063, 0.1250000000000018319 ) ;
#15854=VERTEX_POINT ( 'NONE', #6851 ) ;
#15855=DIRECTION ( 'NONE',  ( -1.101824276508909887E-16, 1.000000000000000000, -0.000000000000000000 ) ) ;
#15857=DIRECTION ( 'NONE',  ( -1.101824276508909887E-16, 1.000000000000000000, -0.000000000000000000 ) ) ;
#15860=CARTESIAN_POINT ( 'NONE',  ( 21.09992658989239089, 30.47145308207317882, 47.04930799450051637 ) ) ;
#15862=DIRECTION ( 'NONE',  ( -1.101824276508909887E-16, 1.000000000000000000, -0.000000000000000000 ) ) ;
#15863=ORIENTED_EDGE ( 'NONE', *, *, #26937, .T. ) ;
#15879=ORIENTED_EDGE ( 'NONE', *, *, #16149, .T. ) ;
#15881=AXIS2_PLACEMENT_3D ( 'NONE', #25064, #22917, #32297 ) ;
#15883=ORIENTED_EDGE ( 'NONE', *, *, #25967, .T. ) ;
#15884=AXIS2_PLACEMENT_3D ( 'NONE', #17645, #17808, #24881 ) ;
#15888=ORIENTED_EDGE ( 'NONE', *, *, #16753, .T. ) ;
#15891=DIRECTION ( 'NONE',  ( -1.000000000000000000, -1.101824276508910010E-16, 0.000000000000000000 ) ) ;
#15892=EDGE_CURVE ( 'NONE', #13866, #27623, #11184, .T. ) ;
#15896=AXIS2_PLACEMENT_3D ( 'NONE', #16216, #26236, #1274 ) ;
#15900=VERTEX_POINT ( 'NONE', #31794 ) ;
#15902=DIRECTION ( 'NONE',  ( -1.101824276508909887E-16, 1.000000000000000000, -0.000000000000000000 ) ) ;
#15907=DIRECTION ( 'NONE',  ( -1.101824276508909887E-16, 1.000000000000000000, -0.000000000000000000 ) ) ;
#15911=VECTOR ( 'NONE', #23570, 1000.000000000000000 ) ;
#15913=AXIS2_PLACEMENT_3D ( 'NONE', #21854, #1076, #6011 ) ;
#15917=AXIS2_PLACEMENT_3D ( 'NONE', #24877, #22395, #401 ) ;
#15918=ORIENTED_EDGE ( 'NONE', *, *, #31944, .T. ) ;
#15919=AXIS2_PLACEMENT_3D ( 'NONE', #14474, #26774, #26602 ) ;
#15922=ORIENTED_EDGE ( 'NONE', *, *, #19025, .T. ) ;
#15928=DIRECTION ( 'NONE',  ( -1.224646799147353207E-16, -1.349345573449484691E-32, 1.000000000000000000 ) ) ;
#15929=ORIENTED_EDGE ( 'NONE', *, *, #17029, .F. ) ;
#15930=CARTESIAN_POINT ( 'NONE',  ( 21.09992658989239089, 30.34143805560860585, 47.04930799450051637 ) ) ;
#15934=CARTESIAN_POINT ( 'NONE',  ( 8.823509210239574685, 31.09164230456639544, 47.04930799450051637 ) ) ;
#15936=AXIS2_PLACEMENT_3D ( 'NONE', #9126, #29306, #6826 ) ;
#15937=CARTESIAN_POINT ( 'NONE',  ( 21.09992658989238734, 31.59164230456639544, 47.04930799450051637 ) ) ;
#15943=DIRECTION ( 'NONE',  ( -1.101824276508909887E-16, 1.000000000000000000, -0.000000000000000000 ) ) ;
#15947=CARTESIAN_POINT ( 'NONE',  ( 8.474859994195286461, 29.34143805560861296, 47.04930799450051637 ) ) ;
#15949=EDGE_LOOP ( 'NONE', ( #3793, #14601, #31692, #24613 ) ) ;
#15954=AXIS2_PLACEMENT_3D ( 'NONE', #28418, #20535, #5931 ) ;
#15962=CARTESIAN_POINT ( 'NONE',  ( 21.09992658989238734, 38.56284415653841791, 47.04930799450051637 ) ) ;
#15982=FACE_OUTER_BOUND ( 'NONE', #5465, .T. ) ;
#15984=CYLINDRICAL_SURFACE ( 'NONE', #2156, 12.62506659569710443 ) ;
#15988=EDGE_LOOP ( 'NONE', ( #28631, #18443, #29447, #11615 ) ) ;
#15992=DIRECTION ( 'NONE',  ( -1.000000000000000000, 0.000000000000000000, 0.000000000000000000 ) ) ;
#15994=LINE ( 'NONE', #3358, #979 ) ;
#15995=ORIENTED_EDGE ( 'NONE', *, *, #29460, .T. ) ;
#15997=CIRCLE ( 'NONE', #28586, 0.1250000000000001110 ) ;
#15998=TOROIDAL_SURFACE ( 'NONE', #27540, 12.40141737965286062, 0.1249999999999998196 ) ;
#16002=AXIS2_PLACEMENT_3D ( 'NONE', #3867, #21576, #32217 ) ;
#16006=CARTESIAN_POINT ( 'NONE',  ( 21.09992658989239089, 25.84184655352419213, 47.04930799450051637 ) ) ;
#16010=CARTESIAN_POINT ( 'NONE',  ( 21.09992658989238734, 38.56284415653841791, 47.04930799450051637 ) ) ;
#16018=CARTESIAN_POINT ( 'NONE',  ( 33.50134396954521776, 29.34164230456639899, 47.04930799450051637 ) ) ;
#16022=DIRECTION ( 'NONE',  ( -1.101824276508909887E-16, 1.000000000000000000, -0.000000000000000000 ) ) ;
#16023=CARTESIAN_POINT ( 'NONE',  ( 33.46699938050304013, 25.72145308207319303, 47.04930799450050927 ) ) ;
#16025=VERTEX_POINT ( 'NONE', #14728 ) ;
#16033=EDGE_CURVE ( 'NONE', #28369, #20933, #21929, .T. ) ;
#16048=FACE_OUTER_BOUND ( 'NONE', #22140, .T. ) ;
#16050=ADVANCED_FACE ( 'NONE', ( #24562 ), #124, .T. ) ;
#16055=AXIS2_PLACEMENT_3D ( 'NONE', #28002, #30784, #25533 ) ;
#16056=DIRECTION ( 'NONE',  ( 1.000000000000000000, 0.000000000000000000, 0.000000000000000000 ) ) ;
#16060=EDGE_LOOP ( 'NONE', ( #19816, #25946, #13500, #21225 ) ) ;
#16067=EDGE_CURVE ( 'NONE', #25102, #13126, #11724, .T. ) ;
#16074=EDGE_CURVE ( 'NONE', #12012, #31925, #270, .T. ) ;
#16076=EDGE_CURVE ( 'NONE', #321, #18497, #6393, .T. ) ;
#16077=ORIENTED_EDGE ( 'NONE', *, *, #13854, .T. ) ;
#16078=CARTESIAN_POINT ( 'NONE',  ( 33.50134396954527460, 24.09164230456639544, 47.04930799450051637 ) ) ;
#16079=CARTESIAN_POINT ( 'NONE',  ( 33.72499318558949710, 27.09184655352419568, 47.04930799450051637 ) ) ;
#16080=DIRECTION ( 'NONE',  ( -1.000000000000000000, -1.101824276508909887E-16, 0.000000000000000000 ) ) ;
#16081=ORIENTED_EDGE ( 'NONE', *, *, #11629, .F. ) ;
#16083=DIRECTION ( 'NONE',  ( -1.101824276508909887E-16, 1.000000000000000000, -0.000000000000000000 ) ) ;
#16087=DIRECTION ( 'NONE',  ( -1.101824276508909887E-16, 1.000000000000000000, -0.000000000000000000 ) ) ;
#16091=CARTESIAN_POINT ( 'NONE',  ( 21.09992658989239089, 28.84184655352418858, 47.04930799450051637 ) ) ;
#16092=CYLINDRICAL_SURFACE ( 'NONE', #14712, 12.36707279061065101 ) ;
#16093=ORIENTED_EDGE ( 'NONE', *, *, #17618, .F. ) ;
#16095=CARTESIAN_POINT ( 'NONE',  ( 8.732853799281725671, 26.22145308207318593, 47.04930799450051637 ) ) ;
#16099=CARTESIAN_POINT ( 'NONE',  ( 33.71785032049133690, 28.46664230456639899, 47.04930799450051637 ) ) ;
#16102=VERTEX_POINT ( 'NONE', #10936 ) ;
#16106=AXIS2_PLACEMENT_3D ( 'NONE', #5767, #15774, #23645 ) ;
#16107=TOROIDAL_SURFACE ( 'NONE', #20305, 12.40141737965285174, 0.1249999999999993200 ) ;
#16116=DIRECTION ( 'NONE',  ( -1.000000000000000000, 0.000000000000000000, 0.000000000000000000 ) ) ;
#16119=CARTESIAN_POINT ( 'NONE',  ( 21.09992658989238734, 38.56284415653841791, 47.04930799450051637 ) ) ;
#16120=DIRECTION ( 'NONE',  ( -1.101824276508909887E-16, 1.000000000000000000, -0.000000000000000000 ) ) ;
#16127=ORIENTED_EDGE ( 'NONE', *, *, #22990, .T. ) ;
#16128=DIRECTION ( 'NONE',  ( -1.101824276508909887E-16, 1.000000000000000000, -0.000000000000000000 ) ) ;
#16129=DIRECTION ( 'NONE',  ( -1.000000000000000000, 0.000000000000000000, 0.000000000000000000 ) ) ;
#16131=CARTESIAN_POINT ( 'NONE',  ( 21.09992658989238734, 31.09164230456639544, 47.04930799450051637 ) ) ;
#16132=CARTESIAN_POINT ( 'NONE',  ( 8.474859994195282908, 38.56284415653841791, 47.04930799450051637 ) ) ;
#16139=AXIS2_PLACEMENT_3D ( 'NONE', #17759, #27777, #5302 ) ;
#16141=DIRECTION ( 'NONE',  ( 1.000000000000000000, 0.000000000000000000, 0.000000000000000000 ) ) ;
#16144=EDGE_LOOP ( 'NONE', ( #13913, #4082, #20845, #7456 ) ) ;
#16148=ADVANCED_FACE ( 'NONE', ( #17826 ), #3320, .T. ) ;
#16149=EDGE_CURVE ( 'NONE', #28443, #5065, #27849, .T. ) ;
#16154=AXIS2_PLACEMENT_3D ( 'NONE', #20026, #7411, #12 ) ;
#16157=AXIS2_PLACEMENT_3D ( 'NONE', #445, #18487, #30500 ) ;
#16159=CARTESIAN_POINT ( 'NONE',  ( 33.46699938050303302, 38.56284415653841791, 47.04930799450051637 ) ) ;
#16162=ORIENTED_EDGE ( 'NONE', *, *, #19059, .F. ) ;
#16165=CARTESIAN_POINT ( 'NONE',  ( 33.46699938050304013, 29.47145308207317882, 47.04930799450050927 ) ) ;
#16166=CARTESIAN_POINT ( 'NONE',  ( 8.474859994195286461, 30.59143805560860585, 47.04930799450051637 ) ) ;
#16173=LINE ( 'NONE', #13258, #18987 ) ;
#16176=CARTESIAN_POINT ( 'NONE',  ( 21.09992658989238734, 38.56284415653841791, 47.04930799450051637 ) ) ;
#16180=CARTESIAN_POINT ( 'NONE',  ( 21.09992658989238734, 32.09184655352418503, 47.04930799450051637 ) ) ;
#16181=CARTESIAN_POINT ( 'NONE',  ( 21.09992658989238734, 38.56284415653841791, 47.04930799450051637 ) ) ;
#16182=ORIENTED_EDGE ( 'NONE', *, *, #2403, .F. ) ;
#16183=DIRECTION ( 'NONE',  ( -1.101824276508909887E-16, 1.000000000000000000, -0.000000000000000000 ) ) ;
#16184=EDGE_CURVE ( 'NONE', #21016, #2064, #11700, .T. ) ;
#16185=TOROIDAL_SURFACE ( 'NONE', #26136, 12.40141737965284108, 0.1249999999999997918 ) ;
#16186=CIRCLE ( 'NONE', #24573, 0.1249999999999966416 ) ;
#16188=AXIS2_PLACEMENT_3D ( 'NONE', #8243, #13811, #18550 ) ;
#16191=AXIS2_PLACEMENT_3D ( 'NONE', #19820, #29851, #4405 ) ;
#16196=AXIS2_PLACEMENT_3D ( 'NONE', #26342, #16323, #16492 ) ;
#16197=AXIS2_PLACEMENT_3D ( 'NONE', #7806, #18445, #11080 ) ;
#16198=ORIENTED_EDGE ( 'NONE', *, *, #24557, .T. ) ;
#16199=DIRECTION ( 'NONE',  ( -1.101824276508909887E-16, 1.000000000000000000, -0.000000000000000000 ) ) ;
#16205=ORIENTED_EDGE ( 'NONE', *, *, #13837, .F. ) ;
#16209=EDGE_CURVE ( 'NONE', #2007, #7282, #31631, .T. ) ;
#16214=VECTOR ( 'NONE', #24266, 1000.000000000000000 ) ;
#16216=CARTESIAN_POINT ( 'NONE',  ( 21.09992658989239089, 29.72145308207318237, 47.04930799450051637 ) ) ;
#16217=EDGE_LOOP ( 'NONE', ( #9929, #12427, #11964, #7564 ) ) ;
#16218=CARTESIAN_POINT ( 'NONE',  ( 33.46699938050303302, 38.56284415653841791, 47.04930799450051637 ) ) ;
#16221=DIRECTION ( 'NONE',  ( -1.101824276508909887E-16, 1.000000000000000000, -0.000000000000000000 ) ) ;
#16229=AXIS2_PLACEMENT_3D ( 'NONE', #10099, #17470, #29787 ) ;
#16231=EDGE_LOOP ( 'NONE', ( #16637, #2275, #9918, #4739 ) ) ;
#16234=CIRCLE ( 'NONE', #5782, 12.27641737965288193 ) ;
#16241=DIRECTION ( 'NONE',  ( -1.000000000000000000, 0.000000000000000000, 0.000000000000000000 ) ) ;
#16245=EDGE_CURVE ( 'NONE', #32203, #11810, #24162, .T. ) ;
#16247=CIRCLE ( 'NONE', #7886, 12.62506659569710443 ) ;
#16251=DIRECTION ( 'NONE',  ( -1.000000000000000000, 0.000000000000000000, 0.000000000000000000 ) ) ;
#16254=EDGE_LOOP ( 'NONE', ( #23147, #10561, #23590, #2778 ) ) ;
#16257=EDGE_CURVE ( 'NONE', #8095, #30111, #17406, .T. ) ;
#16263=DIRECTION ( 'NONE',  ( -1.000000000000000000, -1.101824276508909887E-16, 0.000000000000000000 ) ) ;
#16265=CARTESIAN_POINT ( 'NONE',  ( 33.46699938050303302, 38.56284415653841791, 47.04930799450051637 ) ) ;
#16273=AXIS2_PLACEMENT_3D ( 'NONE', #21618, #14252, #31651 ) ;
#16274=ORIENTED_EDGE ( 'NONE', *, *, #6351, .F. ) ;
#16275=DIRECTION ( 'NONE',  ( -1.000000000000000000, -1.101824276508909887E-16, 0.000000000000000000 ) ) ;
#16278=AXIS2_PLACEMENT_3D ( 'NONE', #19111, #23730, #18633 ) ;
#16279=ORIENTED_EDGE ( 'NONE', *, *, #15042, .T. ) ;
#16283=CARTESIAN_POINT ( 'NONE',  ( 33.37634396954521065, 29.84164230456639899, 47.04930799450051637 ) ) ;
#16285=AXIS2_PLACEMENT_3D ( 'NONE', #21088, #3534, #10626 ) ;
#16286=DIRECTION ( 'NONE',  ( -1.000000000000000000, -1.101824276508909764E-16, 0.000000000000000000 ) ) ;
#16289=CARTESIAN_POINT ( 'NONE',  ( 8.698509210239533829, 26.84164230456639899, 47.04930799450051637 ) ) ;
#16290=DIRECTION ( 'NONE',  ( 0.000000000000000000, -0.000000000000000000, -1.000000000000000000 ) ) ;
#16297=CARTESIAN_POINT ( 'NONE',  ( 21.09992658989239089, 29.96183152705961206, 47.04930799450051637 ) ) ;
#16304=CYLINDRICAL_SURFACE ( 'NONE', #30409, 12.36707279061065101 ) ;
#16309=DIRECTION ( 'NONE',  ( -1.000000000000000000, -1.101824276508909887E-16, 0.000000000000000000 ) ) ;
#16312=AXIS2_PLACEMENT_3D ( 'NONE', #22731, #19608, #2392 ) ;
#16316=AXIS2_PLACEMENT_3D ( 'NONE', #18312, #27689, #8002 ) ;
#16320=EDGE_LOOP ( 'NONE', ( #2801, #6894, #32037, #24661 ) ) ;
#16323=DIRECTION ( 'NONE',  ( -1.224646799147353207E-16, -1.349345573449484691E-32, 1.000000000000000000 ) ) ;
#16334=EDGE_CURVE ( 'NONE', #24129, #25156, #31054, .T. ) ;
#16336=CARTESIAN_POINT ( 'NONE',  ( 8.474859994195286461, 27.09184655352419568, 47.04930799450051637 ) ) ;
#16337=DIRECTION ( 'NONE',  ( -1.000000000000000000, 0.000000000000000000, 0.000000000000000000 ) ) ;
#16340=EDGE_CURVE ( 'NONE', #31649, #8369, #21592, .T. ) ;
#16345=DIRECTION ( 'NONE',  ( -1.000000000000000000, -1.101824276508909764E-16, 0.000000000000000000 ) ) ;
#16348=CARTESIAN_POINT ( 'NONE',  ( 21.09992658989239089, 30.34164230456639544, 47.04930799450051637 ) ) ;
#16349=ORIENTED_EDGE ( 'NONE', *, *, #20637, .T. ) ;
#16355=CARTESIAN_POINT ( 'NONE',  ( 33.46699938050304013, 29.96183152705961206, 47.04930799450051637 ) ) ;
#16358=CARTESIAN_POINT ( 'NONE',  ( 33.46699938050304013, 31.96183152705962272, 47.04930799450051637 ) ) ;
#16362=DIRECTION ( 'NONE',  ( -1.000000000000000000, 0.000000000000000000, 0.000000000000000000 ) ) ;
#16363=AXIS2_PLACEMENT_3D ( 'NONE', #23479, #3122, #30876 ) ;
#16365=ORIENTED_EDGE ( 'NONE', *, *, #20835, .F. ) ;
#16366=EDGE_LOOP ( 'NONE', ( #25581, #23628, #23133, #28116 ) ) ;
#16372=DIRECTION ( 'NONE',  ( -1.000000000000000000, 0.000000000000000000, 0.000000000000000000 ) ) ;
#16373=EDGE_CURVE ( 'NONE', #18749, #19345, #12721, .T. ) ;
#16377=AXIS2_PLACEMENT_3D ( 'NONE', #29483, #4366, #16984 ) ;
#16383=CARTESIAN_POINT ( 'NONE',  ( 8.482002859293455543, 29.71664230456640254, 47.04930799450051637 ) ) ;
#16384=DIRECTION ( 'NONE',  ( -1.000000000000000000, -1.101824276508909887E-16, 0.000000000000000000 ) ) ;
#16400=LINE ( 'NONE', #26259, #9218 ) ;
#16403=EDGE_LOOP ( 'NONE', ( #8811, #31444, #14704, #21671 ) ) ;
#16406=DIRECTION ( 'NONE',  ( -1.101824276508909887E-16, 1.000000000000000000, -0.000000000000000000 ) ) ;
#16407=ORIENTED_EDGE ( 'NONE', *, *, #17408, .F. ) ;
#16413=AXIS2_PLACEMENT_3D ( 'NONE', #4629, #12187, #22182 ) ;
#16423=VERTEX_POINT ( 'NONE', #12352 ) ;
#16424=AXIS2_PLACEMENT_3D ( 'NONE', #574, #8610, #25524 ) ;
#16428=ORIENTED_EDGE ( 'NONE', *, *, #18157, .F. ) ;
#16434=ORIENTED_EDGE ( 'NONE', *, *, #146, .F. ) ;
#16435=CIRCLE ( 'NONE', #27981, 12.36707279061065101 ) ;
#16436=DIRECTION ( 'NONE',  ( -1.101824276508909887E-16, 1.000000000000000000, -0.000000000000000000 ) ) ;
#16444=AXIS2_PLACEMENT_3D ( 'NONE', #14541, #11752, #2058 ) ;
#16445=DIRECTION ( 'NONE',  ( -1.000000000000000000, 0.000000000000000000, 0.000000000000000000 ) ) ;
#16450=CYLINDRICAL_SURFACE ( 'NONE', #11552, 12.36707279061065279 ) ;
#16452=ADVANCED_FACE ( 'NONE', ( #8078 ), #11137, .T. ) ;
#16453=ORIENTED_EDGE ( 'NONE', *, *, #25569, .T. ) ;
#16454=DIRECTION ( 'NONE',  ( -1.000000000000000000, 0.000000000000000000, 0.000000000000000000 ) ) ;
#16456=DIRECTION ( 'NONE',  ( -1.101824276508909887E-16, 1.000000000000000000, -0.000000000000000000 ) ) ;
#16458=DIRECTION ( 'NONE',  ( -1.000000000000000000, 0.000000000000000000, 0.000000000000000000 ) ) ;
#16464=ORIENTED_EDGE ( 'NONE', *, *, #23861, .F. ) ;
#16466=CIRCLE ( 'NONE', #29051, 0.1249999999999983763 ) ;
#16469=DIRECTION ( 'NONE',  ( 0.000000000000000000, -0.000000000000000000, -1.000000000000000000 ) ) ;
#16471=AXIS2_PLACEMENT_3D ( 'NONE', #16078, #26086, #31191 ) ;
#16474=ORIENTED_EDGE ( 'NONE', *, *, #26572, .F. ) ;
#16478=EDGE_CURVE ( 'NONE', #28743, #12476, #3278, .T. ) ;
#16479=ADVANCED_FACE ( 'NONE', ( #31046 ), #1162, .T. ) ;
#16486=AXIS2_PLACEMENT_3D ( 'NONE', #30722, #18220, #28253 ) ;
#16492=DIRECTION ( 'NONE',  ( 1.000000000000000000, 0.000000000000000000, 0.000000000000000000 ) ) ;
#16494=CARTESIAN_POINT ( 'NONE',  ( 21.09992658989238734, 31.21664230456641675, 47.04930799450051637 ) ) ;
#16505=DIRECTION ( 'NONE',  ( -1.101824276508909887E-16, 1.000000000000000000, -0.000000000000000000 ) ) ;
#16508=DIRECTION ( 'NONE',  ( -1.000000000000000000, 0.000000000000000000, 0.000000000000000000 ) ) ;
#16509=ORIENTED_EDGE ( 'NONE', *, *, #28578, .F. ) ;
#16512=CIRCLE ( 'NONE', #28049, 12.36707279061065101 ) ;
#16513=CIRCLE ( 'NONE', #24388, 12.27641737965283042 ) ;
#16514=CIRCLE ( 'NONE', #7628, 12.27641737965288193 ) ;
#16515=VERTEX_POINT ( 'NONE', #15777 ) ;
#16516=EDGE_CURVE ( 'NONE', #6910, #28202, #22127, .T. ) ;
#16518=DIRECTION ( 'NONE',  ( -1.101824276508909887E-16, 1.000000000000000000, -0.000000000000000000 ) ) ;
#16519=ORIENTED_EDGE ( 'NONE', *, *, #18212, .F. ) ;
#16520=CARTESIAN_POINT ( 'NONE',  ( 21.09992658989238734, 38.56284415653841791, 47.04930799450051637 ) ) ;
#16521=DIRECTION ( 'NONE',  ( -1.101824276508909887E-16, 1.000000000000000000, -0.000000000000000000 ) ) ;
#16523=CARTESIAN_POINT ( 'NONE',  ( 8.482002859293405805, 24.96664230456639899, 47.04930799450051637 ) ) ;
#16526=ORIENTED_EDGE ( 'NONE', *, *, #7464, .T. ) ;
#16527=AXIS2_PLACEMENT_3D ( 'NONE', #27610, #7269, #5132 ) ;
#16535=DIRECTION ( 'NONE',  ( -1.000000000000000000, 0.000000000000000000, 0.000000000000000000 ) ) ;
#16547=CARTESIAN_POINT ( 'NONE',  ( 21.09992658989239089, 28.59184655352419213, 47.04930799450051637 ) ) ;
#16549=ORIENTED_EDGE ( 'NONE', *, *, #19785, .T. ) ;
#16556=EDGE_CURVE ( 'NONE', #2570, #28996, #18480, .T. ) ;
#16558=DIRECTION ( 'NONE',  ( -1.101824276508909887E-16, 1.000000000000000000, -0.000000000000000000 ) ) ;
#16562=CARTESIAN_POINT ( 'NONE',  ( 33.72499318558949710, 27.09143805560860940, 47.04930799450051637 ) ) ;
#16566=DIRECTION ( 'NONE',  ( -1.224646799147353207E-16, -1.349345573449484691E-32, 1.000000000000000000 ) ) ;
#16567=ORIENTED_EDGE ( 'NONE', *, *, #6594, .T. ) ;
#16573=ORIENTED_EDGE ( 'NONE', *, *, #3433, .T. ) ;
#16575=AXIS2_PLACEMENT_3D ( 'NONE', #23297, #3096, #15425 ) ;
#16585=EDGE_CURVE ( 'NONE', #3968, #22382, #15326, .T. ) ;
#16586=ADVANCED_FACE ( 'NONE', ( #29553 ), #24616, .T. ) ;
#16590=DIRECTION ( 'NONE',  ( -1.000000000000000000, 0.000000000000000000, 0.000000000000000000 ) ) ;
#16593=CIRCLE ( 'NONE', #2469, 12.36707279061065101 ) ;
#16603=CARTESIAN_POINT ( 'NONE',  ( 8.580227611973585411, 32.55121380581068991, 47.04930799450051637 ) ) ;
#16604=EDGE_CURVE ( 'NONE', #3840, #32154, #6934, .T. ) ;
#16605=DIRECTION ( 'NONE',  ( -1.101824276508909887E-16, 1.000000000000000000, -0.000000000000000000 ) ) ;
#16607=EDGE_LOOP ( 'NONE', ( #11185, #31266, #10552, #24076 ) ) ;
#16608=CYLINDRICAL_SURFACE ( 'NONE', #15489, 12.62506659569710266 ) ;
#16614=DIRECTION ( 'NONE',  ( -1.000000000000000000, 0.000000000000000000, 0.000000000000000000 ) ) ;
#16617=VERTEX_POINT ( 'NONE', #26918 ) ;
#16619=CARTESIAN_POINT ( 'NONE',  ( 21.09992658989238734, 30.96664230456641675, 47.04930799450051637 ) ) ;
#16622=EDGE_CURVE ( 'NONE', #31962, #14214, #6421, .T. ) ;
#16623=CARTESIAN_POINT ( 'NONE',  ( 8.474859994195286461, 24.84184655352419213, 47.04930799450051637 ) ) ;
#16624=CARTESIAN_POINT ( 'NONE',  ( 21.09992658989239089, 25.34164230456639899, 47.04930799450051637 ) ) ;
#16633=DIRECTION ( 'NONE',  ( -1.000000000000000000, 0.000000000000000000, 0.000000000000000000 ) ) ;
#16636=AXIS2_PLACEMENT_3D ( 'NONE', #27578, #17398, #10344 ) ;
#16637=ORIENTED_EDGE ( 'NONE', *, *, #8709, .F. ) ;
#16654=ORIENTED_EDGE ( 'NONE', *, *, #22616, .T. ) ;
#16659=EDGE_CURVE ( 'NONE', #13866, #2064, #14817, .T. ) ;
#16660=CARTESIAN_POINT ( 'NONE',  ( 33.72499318558949000, 38.56284415653841791, 47.04930799450051637 ) ) ;
#16661=EDGE_CURVE ( 'NONE', #16423, #29220, #17944, .T. ) ;
#16665=UNCERTAINTY_MEASURE_WITH_UNIT (LENGTH_MEASURE( 1.000000000000000082E-05 ), #26106, 'distance_accuracy_value', 'NONE');
#16667=ORIENTED_EDGE ( 'NONE', *, *, #3851, .T. ) ;
#16668=TOROIDAL_SURFACE ( 'NONE', #2533, 12.40141737965286772, 0.1250000000000003331 ) ;
#16670=CIRCLE ( 'NONE', #19826, 0.1250000000000001110 ) ;
#16672=VERTEX_POINT ( 'NONE', #9198 ) ;
#16673=CARTESIAN_POINT ( 'NONE',  ( 8.474859994195286461, 25.84184655352419213, 47.04930799450051637 ) ) ;
#16674=CYLINDRICAL_SURFACE ( 'NONE', #21435, 12.62506659569710266 ) ;
#16681=ORIENTED_EDGE ( 'NONE', *, *, #23594, .F. ) ;
#16682=DIRECTION ( 'NONE',  ( -1.101824276508909887E-16, 1.000000000000000000, -0.000000000000000000 ) ) ;
#16683=CIRCLE ( 'NONE', #23504, 12.62506659569710443 ) ;
#16684=ORIENTED_EDGE ( 'NONE', *, *, #11523, .F. ) ;
#16686=DIRECTION ( 'NONE',  ( 0.000000000000000000, -0.000000000000000000, -1.000000000000000000 ) ) ;
#16689=CARTESIAN_POINT ( 'NONE',  ( 33.37634396954521065, 30.34164230456639544, 47.04930799450051637 ) ) ;
#16696=DIRECTION ( 'NONE',  ( -1.101824276508909887E-16, 1.000000000000000000, -0.000000000000000000 ) ) ;
#16701=DIRECTION ( 'NONE',  ( -1.101824276508909887E-16, 1.000000000000000000, -0.000000000000000000 ) ) ;
#16703=ORIENTED_EDGE ( 'NONE', *, *, #2031, .F. ) ;
#16705=ORIENTED_EDGE ( 'NONE', *, *, #25967, .F. ) ;
#16708=VERTEX_POINT ( 'NONE', #24780 ) ;
#16709=AXIS2_PLACEMENT_3D ( 'NONE', #14116, #24604, #14603 ) ;
#16714=DIRECTION ( 'NONE',  ( -1.000000000000000000, 0.000000000000000000, 0.000000000000000000 ) ) ;
#16715=ORIENTED_EDGE ( 'NONE', *, *, #4202, .F. ) ;
#16724=CARTESIAN_POINT ( 'NONE',  ( 8.698509210239588896, 32.59164230456639899, 47.04930799450051637 ) ) ;
#16725=CARTESIAN_POINT ( 'NONE',  ( 21.09992658989239089, 27.96664230456639899, 47.04930799450051637 ) ) ;
#16730=AXIS2_PLACEMENT_3D ( 'NONE', #26015, #15857, #8152 ) ;
#16732=CIRCLE ( 'NONE', #23023, 0.1250000000000001110 ) ;
#16741=ADVANCED_FACE ( 'NONE', ( #30362 ), #14299, .T. ) ;
#16744=EDGE_CURVE ( 'NONE', #28434, #7034, #142, .T. ) ;
#16747=AXIS2_PLACEMENT_3D ( 'NONE', #13386, #23382, #889 ) ;
#16752=FACE_OUTER_BOUND ( 'NONE', #11038, .T. ) ;
#16753=EDGE_CURVE ( 'NONE', #16795, #20430, #26866, .T. ) ;
#16765=AXIS2_PLACEMENT_3D ( 'NONE', #1143, #11480, #26577 ) ;
#16772=AXIS2_PLACEMENT_3D ( 'NONE', #9223, #13994, #3805 ) ;
#16776=CARTESIAN_POINT ( 'NONE',  ( 21.09992658989238734, 38.56284415653841791, 47.04930799450051637 ) ) ;
#16780=CARTESIAN_POINT ( 'NONE',  ( 33.72499318558949000, 38.56284415653841791, 47.04930799450051637 ) ) ;
#16781=ADVANCED_FACE ( 'NONE', ( #12317 ), #12809, .T. ) ;
#16785=CARTESIAN_POINT ( 'NONE',  ( 33.46699938050304013, 38.56284415653841791, 47.04930799450051637 ) ) ;
#16793=VERTEX_POINT ( 'NONE', #12650 ) ;
#16795=VERTEX_POINT ( 'NONE', #22638 ) ;
#16798=CIRCLE ( 'NONE', #17318, 12.62506659569710266 ) ;
#16799=AXIS2_PLACEMENT_3D ( 'NONE', #10133, #22588, #14730 ) ;
#16803=DIRECTION ( 'NONE',  ( -1.101824276508909887E-16, 1.000000000000000000, -0.000000000000000000 ) ) ;
#16805=CARTESIAN_POINT ( 'NONE',  ( 8.732853799281738105, 24.21183152705959785, 47.04930799450051637 ) ) ;
#16812=DIRECTION ( 'NONE',  ( -1.101824276508909887E-16, 1.000000000000000000, -0.000000000000000000 ) ) ;
#16821=DIRECTION ( 'NONE',  ( -1.101824276508909887E-16, 1.000000000000000000, -0.000000000000000000 ) ) ;
#16826=ORIENTED_EDGE ( 'NONE', *, *, #7723, .T. ) ;
#16827=AXIS2_PLACEMENT_3D ( 'NONE', #24527, #12067, #22061 ) ;
#16829=DIRECTION ( 'NONE',  ( -1.101824276508909887E-16, 1.000000000000000000, -0.000000000000000000 ) ) ;
#16832=ORIENTED_EDGE ( 'NONE', *, *, #26982, .T. ) ;
#16835=ORIENTED_EDGE ( 'NONE', *, *, #32323, .F. ) ;
#16836=ADVANCED_FACE ( 'NONE', ( #30691 ), #2792, .T. ) ;
#16838=AXIS2_PLACEMENT_3D ( 'NONE', #10902, #10750, #1044 ) ;
#16839=AXIS2_PLACEMENT_3D ( 'NONE', #24051, #9453, #6338 ) ;
#16843=EDGE_CURVE ( 'NONE', #30925, #10687, #7503, .T. ) ;
#16845=ORIENTED_EDGE ( 'NONE', *, *, #20445, .F. ) ;
#16857=ORIENTED_EDGE ( 'NONE', *, *, #26072, .F. ) ;
#16860=CARTESIAN_POINT ( 'NONE',  ( 21.09992658989238734, 38.56284415653841791, 47.04930799450051637 ) ) ;
#16861=CARTESIAN_POINT ( 'NONE',  ( 21.09992658989238734, 38.56284415653841791, 47.04930799450051637 ) ) ;
#16862=CARTESIAN_POINT ( 'NONE',  ( 21.09992658989239089, 25.22145308207319303, 47.04930799450051637 ) ) ;
#16867=LINE ( 'NONE', #16218, #22894 ) ;
#16872=ORIENTED_EDGE ( 'NONE', *, *, #31352, .T. ) ;
#16874=AXIS2_PLACEMENT_3D ( 'NONE', #13381, #23377, #15508 ) ;
#16876=FACE_OUTER_BOUND ( 'NONE', #5812, .T. ) ;
#16880=CIRCLE ( 'NONE', #15844, 0.1250000000000001110 ) ;
#16881=EDGE_CURVE ( 'NONE', #1375, #17361, #8025, .T. ) ;
#16882=AXIS2_PLACEMENT_3D ( 'NONE', #349, #29918, #24978 ) ;
#16885=CARTESIAN_POINT ( 'NONE',  ( 21.09992658989239089, 29.84164230456639899, 47.04930799450051637 ) ) ;
#16886=CARTESIAN_POINT ( 'NONE',  ( 8.474859994195286461, 27.59184655352419568, 47.04930799450051637 ) ) ;
#16893=CYLINDRICAL_SURFACE ( 'NONE', #3930, 12.62506659569710266 ) ;
#16894=CARTESIAN_POINT ( 'NONE',  ( 8.474859994195282908, 38.56284415653841791, 47.04930799450051637 ) ) ;
#16895=ORIENTED_EDGE ( 'NONE', *, *, #19025, .F. ) ;
#16896=ORIENTED_EDGE ( 'NONE', *, *, #20154, .F. ) ;
#16904=ORIENTED_EDGE ( 'NONE', *, *, #19219, .T. ) ;
#16905=DIRECTION ( 'NONE',  ( -1.101824276508909887E-16, 1.000000000000000000, -0.000000000000000000 ) ) ;
#16908=EDGE_LOOP ( 'NONE', ( #21205, #24641, #940, #25182 ) ) ;
#16912=VERTEX_POINT ( 'NONE', #18353 ) ;
#16915=CYLINDRICAL_SURFACE ( 'NONE', #30083, 12.62506659569710266 ) ;
#16924=CIRCLE ( 'NONE', #30052, 0.1249999999999966416 ) ;
#16925=ADVANCED_FACE ( 'NONE', ( #3580 ), #9060, .T. ) ;
#16928=LINE ( 'NONE', #9388, #12513 ) ;
#16934=CIRCLE ( 'NONE', #15896, 12.36707279061065101 ) ;
#16935=LINE ( 'NONE', #4965, #18414 ) ;
#16941=ORIENTED_EDGE ( 'NONE', *, *, #1031, .T. ) ;
#16944=DIRECTION ( 'NONE',  ( -1.101824276508909887E-16, 1.000000000000000000, -0.000000000000000000 ) ) ;
#16950=AXIS2_PLACEMENT_3D ( 'NONE', #5871, #30974, #20463 ) ;
#16951=ORIENTED_EDGE ( 'NONE', *, *, #23234, .F. ) ;
#16953=VERTEX_POINT ( 'NONE', #28383 ) ;
#16954=ORIENTED_EDGE ( 'NONE', *, *, #5229, .T. ) ;
#16955=TOROIDAL_SURFACE ( 'NONE', #15917, 12.40141737965286062, 0.1249999999999998196 ) ;
#16956=AXIS2_PLACEMENT_3D ( 'NONE', #5315, #14842, #15319 ) ;
#16960=EDGE_CURVE ( 'NONE', #22668, #27774, #16924, .T. ) ;
#16962=DIRECTION ( 'NONE',  ( -1.000000000000000000, 0.000000000000000000, 0.000000000000000000 ) ) ;
#16963=DIRECTION ( 'NONE',  ( -1.101824276508909887E-16, 1.000000000000000000, -0.000000000000000000 ) ) ;
#16966=EDGE_LOOP ( 'NONE', ( #21336, #26687, #21645, #25797 ) ) ;
#16968=ORIENTED_EDGE ( 'NONE', *, *, #12421, .T. ) ;
#16969=DIRECTION ( 'NONE',  ( 1.000000000000000000, 0.000000000000000000, 0.000000000000000000 ) ) ;
#16972=ORIENTED_EDGE ( 'NONE', *, *, #22293, .T. ) ;
#16974=LINE ( 'NONE', #29794, #27472 ) ;
#16975=CARTESIAN_POINT ( 'NONE',  ( 21.09992658989239089, 25.96664230456639899, 47.04930799450051637 ) ) ;
#16977=CARTESIAN_POINT ( 'NONE',  ( 21.09992658989238734, 31.84164230456639544, 47.04930799450051637 ) ) ;
#16978=DIRECTION ( 'NONE',  ( -1.101824276508909887E-16, 1.000000000000000000, -0.000000000000000000 ) ) ;
#16980=FACE_OUTER_BOUND ( 'NONE', #10952, .T. ) ;
#16984=DIRECTION ( 'NONE',  ( 1.000000000000000000, 0.000000000000000000, 0.000000000000000000 ) ) ;
#16985=VERTEX_POINT ( 'NONE', #1604 ) ;
#16993=CIRCLE ( 'NONE', #24862, 12.62506659569710266 ) ;
#16995=AXIS2_PLACEMENT_3D ( 'NONE', #20455, #13257, #6016 ) ;
#16997=CYLINDRICAL_SURFACE ( 'NONE', #25048, 12.62506659569710266 ) ;
#17000=ORIENTED_EDGE ( 'NONE', *, *, #21788, .T. ) ;
#17001=CARTESIAN_POINT ( 'NONE',  ( 33.46699938050303302, 38.56284415653841791, 47.04930799450051637 ) ) ;
#17025=DIRECTION ( 'NONE',  ( -1.101824276508909887E-16, 1.000000000000000000, -0.000000000000000000 ) ) ;
#17029=EDGE_CURVE ( 'NONE', #31427, #12749, #25335, .T. ) ;
#17031=DIRECTION ( 'NONE',  ( -1.101824276508909887E-16, 1.000000000000000000, -0.000000000000000000 ) ) ;
#17035=DIRECTION ( 'NONE',  ( -1.101824276508909887E-16, 1.000000000000000000, -0.000000000000000000 ) ) ;
#17036=EDGE_CURVE ( 'NONE', #17110, #23862, #12218, .T. ) ;
#17037=EDGE_CURVE ( 'NONE', #23072, #24621, #22157, .T. ) ;
#17044=DIRECTION ( 'NONE',  ( -1.000000000000000000, 0.000000000000000000, 0.000000000000000000 ) ) ;
#17054=EDGE_LOOP ( 'NONE', ( #24506, #11295, #3617, #4656 ) ) ;
#17060=LINE ( 'NONE', #29552, #15488 ) ;
#17066=CARTESIAN_POINT ( 'NONE',  ( 33.37634396954524618, 26.59164230456639899, 47.04930799450051637 ) ) ;
#17068=EDGE_CURVE ( 'NONE', #16102, #8095, #24789, .T. ) ;
#17069=CARTESIAN_POINT ( 'NONE',  ( 21.09992658989239089, 28.84164230456639544, 47.04930799450051637 ) ) ;
#17073=VERTEX_POINT ( 'NONE', #8996 ) ;
#17076=AXIS2_PLACEMENT_3D ( 'NONE', #28942, #1518, #19068 ) ;
#17078=EDGE_CURVE ( 'NONE', #9758, #21045, #18991, .T. ) ;
#17090=AXIS2_PLACEMENT_3D ( 'NONE', #1813, #4104, #31536 ) ;
#17093=CARTESIAN_POINT ( 'NONE',  ( 21.09992658989238734, 38.56284415653841791, 47.04930799450051637 ) ) ;
#17097=CARTESIAN_POINT ( 'NONE',  ( 21.09992658989239089, 28.59164230456639544, 47.04930799450051637 ) ) ;
#17103=VECTOR ( 'NONE', #17774, 1000.000000000000000 ) ;
#17104=DIRECTION ( 'NONE',  ( -1.101824276508909887E-16, 1.000000000000000000, -0.000000000000000000 ) ) ;
#17108=DIRECTION ( 'NONE',  ( -1.000000000000000000, 0.000000000000000000, 0.000000000000000000 ) ) ;
#17110=VERTEX_POINT ( 'NONE', #2093 ) ;
#17112=DIRECTION ( 'NONE',  ( 1.000000000000000000, 0.000000000000000000, 0.000000000000000000 ) ) ;
#17113=DIRECTION ( 'NONE',  ( 0.000000000000000000, -0.000000000000000000, -1.000000000000000000 ) ) ;
#17114=EDGE_CURVE ( 'NONE', #8095, #15696, #29676, .T. ) ;
#17117=EDGE_CURVE ( 'NONE', #1400, #12749, #682, .T. ) ;
#17121=ORIENTED_EDGE ( 'NONE', *, *, #23309, .T. ) ;
#17123=AXIS2_PLACEMENT_3D ( 'NONE', #15767, #17734, #18378 ) ;
#17130=DIRECTION ( 'NONE',  ( 1.000000000000000000, 0.000000000000000000, 0.000000000000000000 ) ) ;
#17131=CARTESIAN_POINT ( 'NONE',  ( 33.46699938050304013, 24.47145308207319303, 47.04930799450050927 ) ) ;
#17135=CARTESIAN_POINT ( 'NONE',  ( 8.698509210239523171, 25.84164230456639899, 47.04930799450051637 ) ) ;
#17138=FACE_OUTER_BOUND ( 'NONE', #13464, .T. ) ;
#17142=CARTESIAN_POINT ( 'NONE',  ( 8.732853799281738105, 25.21183152705960140, 47.04930799450051637 ) ) ;
#17145=CARTESIAN_POINT ( 'NONE',  ( 21.09992658989239089, 24.59164230456639544, 47.04930799450051637 ) ) ;
#17148=EDGE_CURVE ( 'NONE', #4270, #22296, #18522, .T. ) ;
#17149=EDGE_CURVE ( 'NONE', #15696, #12384, #22175, .T. ) ;
#17156=AXIS2_PLACEMENT_3D ( 'NONE', #8404, #10719, #23809 ) ;
#17157=AXIS2_PLACEMENT_3D ( 'NONE', #13778, #3271, #8688 ) ;
#17165=DIRECTION ( 'NONE',  ( -1.000000000000000000, 0.000000000000000000, 0.000000000000000000 ) ) ;
#17167=DIRECTION ( 'NONE',  ( -1.000000000000000000, -1.101824276508909764E-16, 0.000000000000000000 ) ) ;
#17168=ADVANCED_FACE ( 'NONE', ( #121 ), #1209, .T. ) ;
#17172=CARTESIAN_POINT ( 'NONE',  ( 8.474859994195286461, 28.34143805560861296, 47.04930799450051637 ) ) ;
#17174=ORIENTED_EDGE ( 'NONE', *, *, #19102, .T. ) ;
#17175=DIRECTION ( 'NONE',  ( -1.000000000000000000, 0.000000000000000000, 0.000000000000000000 ) ) ;
#17184=DIRECTION ( 'NONE',  ( 1.000000000000000000, 0.000000000000000000, 0.000000000000000000 ) ) ;
#17186=ORIENTED_EDGE ( 'NONE', *, *, #13988, .F. ) ;
#17187=AXIS2_PLACEMENT_3D ( 'NONE', #11891, #21394, #14031 ) ;
#17192=TOROIDAL_SURFACE ( 'NONE', #13533, 12.40141737965286239, 0.1250000000000005551 ) ;
#17205=VERTEX_POINT ( 'NONE', #20138 ) ;
#17217=EDGE_CURVE ( 'NONE', #1073, #3554, #2261, .T. ) ;
#17218=EDGE_LOOP ( 'NONE', ( #12983, #5728, #15531, #28000 ) ) ;
#17219=TOROIDAL_SURFACE ( 'NONE', #987, 12.61792373059899752, 0.1250000000000005274 ) ;
#17221=FACE_OUTER_BOUND ( 'NONE', #11495, .T. ) ;
#17226=ORIENTED_EDGE ( 'NONE', *, *, #10655, .F. ) ;
#17239=CARTESIAN_POINT ( 'NONE',  ( 8.698509210239553369, 28.59164230456639544, 47.04930799450051637 ) ) ;
#17240=AXIS2_PLACEMENT_3D ( 'NONE', #23620, #16221, #23299 ) ;
#17241=CIRCLE ( 'NONE', #28275, 12.62506659569710266 ) ;
#17243=AXIS2_PLACEMENT_3D ( 'NONE', #10348, #20343, #7891 ) ;
#17248=CARTESIAN_POINT ( 'NONE',  ( 21.09992658989239089, 28.71664230456639899, 47.04930799450051637 ) ) ;
#17249=EDGE_CURVE ( 'NONE', #24454, #20832, #21660, .T. ) ;
#17250=VERTEX_POINT ( 'NONE', #23415 ) ;
#17251=CYLINDRICAL_SURFACE ( 'NONE', #25909, 12.36707279061065101 ) ;
#17253=AXIS2_PLACEMENT_3D ( 'NONE', #1881, #23879, #11255 ) ;
#17265=DIRECTION ( 'NONE',  ( 0.000000000000000000, -0.000000000000000000, -1.000000000000000000 ) ) ;
#17267=CYLINDRICAL_SURFACE ( 'NONE', #31845, 12.62506659569710266 ) ;
#17270=DIRECTION ( 'NONE',  ( -1.000000000000000000, 0.000000000000000000, 0.000000000000000000 ) ) ;
#17274=DIRECTION ( 'NONE',  ( -1.101824276508909887E-16, 1.000000000000000000, -0.000000000000000000 ) ) ;
#17283=AXIS2_PLACEMENT_3D ( 'NONE', #32087, #14526, #22720 ) ;
#17284=AXIS2_PLACEMENT_3D ( 'NONE', #11528, #31560, #1030 ) ;
#17286=EDGE_CURVE ( 'NONE', #12709, #11810, #11201, .T. ) ;
#17288=AXIS2_PLACEMENT_3D ( 'NONE', #18032, #5571, #3089 ) ;
#17294=DIRECTION ( 'NONE',  ( -1.101824276508909887E-16, 1.000000000000000000, -0.000000000000000000 ) ) ;
#17295=AXIS2_PLACEMENT_3D ( 'NONE', #30493, #15221, #12773 ) ;
#17297=EDGE_CURVE ( 'NONE', #22668, #2021, #26919, .T. ) ;
#17300=ORIENTED_EDGE ( 'NONE', *, *, #23632, .T. ) ;
#17301=CARTESIAN_POINT ( 'NONE',  ( 21.09992658989239089, 29.59164230456639899, 47.04930799450051637 ) ) ;
#17305=CYLINDRICAL_SURFACE ( 'NONE', #6563, 12.36707279061065279 ) ;
#17306=DIRECTION ( 'NONE',  ( -1.000000000000000000, 0.000000000000000000, 0.000000000000000000 ) ) ;
#17310=ORIENTED_EDGE ( 'NONE', *, *, #2623, .F. ) ;
#17312=FACE_OUTER_BOUND ( 'NONE', #17537, .T. ) ;
#17314=DIRECTION ( 'NONE',  ( -1.101824276508909887E-16, 1.000000000000000000, -0.000000000000000000 ) ) ;
#17318=AXIS2_PLACEMENT_3D ( 'NONE', #19849, #12969, #7712 ) ;
#17321=AXIS2_PLACEMENT_3D ( 'NONE', #24464, #1979, #6744 ) ;
#17323=VERTEX_POINT ( 'NONE', #25721 ) ;
#17327=EDGE_LOOP ( 'NONE', ( #20496, #27633, #16872, #1407 ) ) ;
#17328=ORIENTED_EDGE ( 'NONE', *, *, #26081, .T. ) ;
#17329=CARTESIAN_POINT ( 'NONE',  ( 21.09992658989239089, 27.59164230456639544, 47.04930799450051637 ) ) ;
#17331=EDGE_CURVE ( 'NONE', #20581, #28135, #28508, .T. ) ;
#17332=CYLINDRICAL_SURFACE ( 'NONE', #14647, 12.62506659569710266 ) ;
#17333=ADVANCED_FACE ( 'NONE', ( #30494 ), #10157, .T. ) ;
#17339=VECTOR ( 'NONE', #28337, 1000.000000000000000 ) ;
#17342=ADVANCED_FACE ( 'NONE', ( #8485 ), #31630, .T. ) ;
#17348=CARTESIAN_POINT ( 'NONE',  ( 21.09992658989238734, 31.59143805560860585, 47.04930799450051637 ) ) ;
#17354=ORIENTED_EDGE ( 'NONE', *, *, #31432, .T. ) ;
#17355=DIRECTION ( 'NONE',  ( -1.000000000000000000, 0.000000000000000000, 0.000000000000000000 ) ) ;
#17359=CARTESIAN_POINT ( 'NONE',  ( 8.482002859293798380, 31.21664230456641675, 47.04930799450051637 ) ) ;
#17361=VERTEX_POINT ( 'NONE', #16023 ) ;
#17367=CIRCLE ( 'NONE', #3659, 0.1249999999999966416 ) ;
#17372=AXIS2_PLACEMENT_3D ( 'NONE', #28689, #6205, #28860 ) ;
#17376=LINE ( 'NONE', #8032, #4660 ) ;
#17384=DIRECTION ( 'NONE',  ( -1.000000000000000000, -1.101824276508909887E-16, 0.000000000000000000 ) ) ;
#17386=DIRECTION ( 'NONE',  ( -1.101824276508909887E-16, 1.000000000000000000, -0.000000000000000000 ) ) ;
#17387=AXIS2_PLACEMENT_3D ( 'NONE', #22229, #22725, #29795 ) ;
#17389=DIRECTION ( 'NONE',  ( -1.101824276508909887E-16, 1.000000000000000000, -0.000000000000000000 ) ) ;
#17390=AXIS2_PLACEMENT_3D ( 'NONE', #19792, #22583, #4704 ) ;
#17395=EDGE_LOOP ( 'NONE', ( #12455, #17452, #15103, #2779 ) ) ;
#17398=DIRECTION ( 'NONE',  ( -1.101824276508909887E-16, 1.000000000000000000, -0.000000000000000000 ) ) ;
#17400=ORIENTED_EDGE ( 'NONE', *, *, #2031, .T. ) ;
#17406=CIRCLE ( 'NONE', #633, 12.62506659569710443 ) ;
#17408=EDGE_CURVE ( 'NONE', #10801, #30753, #24217, .T. ) ;
#17411=AXIS2_PLACEMENT_3D ( 'NONE', #25325, #1284, #13615 ) ;
#17413=ORIENTED_EDGE ( 'NONE', *, *, #9667, .T. ) ;
#17414=CARTESIAN_POINT ( 'NONE',  ( 21.09992658989239089, 25.59164230456639899, 47.04930799450051637 ) ) ;
#17417=ORIENTED_EDGE ( 'NONE', *, *, #10814, .F. ) ;
#17422=FACE_OUTER_BOUND ( 'NONE', #30589, .T. ) ;
#17423=DIRECTION ( 'NONE',  ( -1.000000000000000000, 0.000000000000000000, 0.000000000000000000 ) ) ;
#17425=CARTESIAN_POINT ( 'NONE',  ( 21.09992658989239089, 26.09164230456639899, 47.04930799450051637 ) ) ;
#17434=DIRECTION ( 'NONE',  ( -1.000000000000000000, 0.000000000000000000, 0.000000000000000000 ) ) ;
#17436=DIRECTION ( 'NONE',  ( -1.101824276508909887E-16, 1.000000000000000000, -0.000000000000000000 ) ) ;
#17444=ORIENTED_EDGE ( 'NONE', *, *, #19585, .T. ) ;
#17448=DIRECTION ( 'NONE',  ( -1.101824276508909887E-16, 1.000000000000000000, -0.000000000000000000 ) ) ;
#17449=ADVANCED_FACE ( 'NONE', ( #11269 ), #4373, .T. ) ;
#17450=DIRECTION ( 'NONE',  ( 1.000000000000000000, 0.000000000000000000, 0.000000000000000000 ) ) ;
#17452=ORIENTED_EDGE ( 'NONE', *, *, #5127, .T. ) ;
#17454=EDGE_CURVE ( 'NONE', #22296, #16912, #9610, .T. ) ;
#17456=EDGE_CURVE ( 'NONE', #5065, #17073, #12242, .T. ) ;
#17459=CYLINDRICAL_SURFACE ( 'NONE', #22435, 12.62506659569710443 ) ;
#17460=EDGE_LOOP ( 'NONE', ( #26966, #30418, #2444, #4702 ) ) ;
#17464=LINE ( 'NONE', #5155, #18221 ) ;
#17467=DIRECTION ( 'NONE',  ( -1.000000000000000000, -1.101824276508909887E-16, 0.000000000000000000 ) ) ;
#17469=DIRECTION ( 'NONE',  ( -1.101824276508909887E-16, 1.000000000000000000, -0.000000000000000000 ) ) ;
#17470=DIRECTION ( 'NONE',  ( -1.224646799147353207E-16, -1.349345573449484691E-32, 1.000000000000000000 ) ) ;
#17471=DIRECTION ( 'NONE',  ( -1.101824276508909887E-16, 1.000000000000000000, -0.000000000000000000 ) ) ;
#17472=CARTESIAN_POINT ( 'NONE',  ( 8.732853799281734553, 38.56284415653841791, 47.04930799450051637 ) ) ;
#17473=ORIENTED_EDGE ( 'NONE', *, *, #5822, .T. ) ;
#17474=CARTESIAN_POINT ( 'NONE',  ( 21.09992658989239089, 26.22145308207318593, 47.04930799450051637 ) ) ;
#17475=CARTESIAN_POINT ( 'NONE',  ( 8.474859994195286461, 30.34184655352422411, 47.04930799450051637 ) ) ;
#17477=DIRECTION ( 'NONE',  ( 1.000000000000000000, 0.000000000000000000, 0.000000000000000000 ) ) ;
#17483=AXIS2_PLACEMENT_3D ( 'NONE', #2080, #12105, #22095 ) ;
#17484=ADVANCED_FACE ( 'NONE', ( #1729 ), #702, .T. ) ;
#17486=DIRECTION ( 'NONE',  ( -1.224646799147353207E-16, -1.349345573449484691E-32, 1.000000000000000000 ) ) ;
#17488=EDGE_CURVE ( 'NONE', #8205, #26804, #16435, .T. ) ;
#17491=ORIENTED_EDGE ( 'NONE', *, *, #15279, .T. ) ;
#17494=CIRCLE ( 'NONE', #20632, 12.62506659569710266 ) ;
#17495=ORIENTED_EDGE ( 'NONE', *, *, #6146, .F. ) ;
#17500=CARTESIAN_POINT ( 'NONE',  ( 8.482002859293784169, 30.21664230456641675, 47.04930799450051637 ) ) ;
#17513=CARTESIAN_POINT ( 'NONE',  ( 33.46699938050304013, 38.56284415653841791, 47.04930799450051637 ) ) ;
#17514=ORIENTED_EDGE ( 'NONE', *, *, #1851, .F. ) ;
#17518=DIRECTION ( 'NONE',  ( -1.101824276508909887E-16, 1.000000000000000000, -0.000000000000000000 ) ) ;
#17519=DIRECTION ( 'NONE',  ( -1.101824276508909887E-16, 1.000000000000000000, -0.000000000000000000 ) ) ;
#17524=CARTESIAN_POINT ( 'NONE',  ( 8.698509210239588896, 32.59164230456639899, 47.04930799450051637 ) ) ;
#17525=DIRECTION ( 'NONE',  ( -1.101824276508909887E-16, 1.000000000000000000, -0.000000000000000000 ) ) ;
#17532=TOROIDAL_SURFACE ( 'NONE', #6003, 12.61792373059894246, 0.1249999999999989730 ) ;
#17537=EDGE_LOOP ( 'NONE', ( #19166, #9176, #4361, #18165 ) ) ;
#17539=EDGE_LOOP ( 'NONE', ( #14115, #32438, #1608, #23758 ) ) ;
#17542=DIRECTION ( 'NONE',  ( -1.101824276508909887E-16, 1.000000000000000000, -0.000000000000000000 ) ) ;
#17558=ORIENTED_EDGE ( 'NONE', *, *, #7379, .F. ) ;
#17565=DIRECTION ( 'NONE',  ( -1.000000000000000000, 0.000000000000000000, 0.000000000000000000 ) ) ;
#17571=EDGE_CURVE ( 'NONE', #19822, #9936, #20646, .T. ) ;
#17573=EDGE_CURVE ( 'NONE', #14283, #593, #5441, .T. ) ;
#17575=AXIS2_PLACEMENT_3D ( 'NONE', #20739, #237, #20580 ) ;
#17583=CARTESIAN_POINT ( 'NONE',  ( 8.698509210239571132, 30.84164230456639544, 47.04930799450051637 ) ) ;
#17584=DIRECTION ( 'NONE',  ( -1.000000000000000000, 0.000000000000000000, 0.000000000000000000 ) ) ;
#17592=ORIENTED_EDGE ( 'NONE', *, *, #27757, .T. ) ;
#17596=AXIS2_PLACEMENT_3D ( 'NONE', #21363, #31728, #11707 ) ;
#17597=EDGE_CURVE ( 'NONE', #4270, #27697, #19582, .T. ) ;
#17610=CARTESIAN_POINT ( 'NONE',  ( 21.09992658989238734, 32.59164230456639899, 47.04930799450051637 ) ) ;
#17612=DIRECTION ( 'NONE',  ( -1.101824276508909887E-16, 1.000000000000000000, -0.000000000000000000 ) ) ;
#17613=LINE ( 'NONE', #27629, #17103 ) ;
#17615=ORIENTED_EDGE ( 'NONE', *, *, #13439, .T. ) ;
#17617=EDGE_LOOP ( 'NONE', ( #5700, #2764, #15638, #17823 ) ) ;
#17618=EDGE_CURVE ( 'NONE', #12345, #14664, #2298, .T. ) ;
#17620=CARTESIAN_POINT ( 'NONE',  ( 21.09992658989238734, 38.56284415653841791, 47.04930799450051637 ) ) ;
#17622=AXIS2_PLACEMENT_3D ( 'NONE', #4997, #2525, #12551 ) ;
#17624=DIRECTION ( 'NONE',  ( -1.101824276508909887E-16, 1.000000000000000000, -0.000000000000000000 ) ) ;
#17627=DIRECTION ( 'NONE',  ( -1.101824276508909887E-16, 1.000000000000000000, -0.000000000000000000 ) ) ;
#17629=CARTESIAN_POINT ( 'NONE',  ( 21.09992658989238734, 38.56284415653841791, 47.04930799450051637 ) ) ;
#17632=CARTESIAN_POINT ( 'NONE',  ( 33.37634396954521776, 29.59164230456639899, 47.04930799450051637 ) ) ;
#17645=CARTESIAN_POINT ( 'NONE',  ( 33.50134396954519644, 31.09164230456639544, 47.04930799450051637 ) ) ;
#17646=ORIENTED_EDGE ( 'NONE', *, *, #14856, .F. ) ;
#17657=ORIENTED_EDGE ( 'NONE', *, *, #18558, .F. ) ;
#17658=VERTEX_POINT ( 'NONE', #6110 ) ;
#17661=DIRECTION ( 'NONE',  ( -1.000000000000000000, -1.101824276508909887E-16, 0.000000000000000000 ) ) ;
#17665=VERTEX_POINT ( 'NONE', #540 ) ;
#17669=ORIENTED_EDGE ( 'NONE', *, *, #221, .T. ) ;
#17670=DIRECTION ( 'NONE',  ( -1.101824276508909887E-16, 1.000000000000000000, -0.000000000000000000 ) ) ;
#17674=DIRECTION ( 'NONE',  ( -1.101824276508909887E-16, 1.000000000000000000, -0.000000000000000000 ) ) ;
#17678=CARTESIAN_POINT ( 'NONE',  ( 21.09992658989238734, 32.54735957529758394, 47.04930799450051637 ) ) ;
#17679=VERTEX_POINT ( 'NONE', #30593 ) ;
#17685=AXIS2_PLACEMENT_3D ( 'NONE', #29079, #26293, #29408 ) ;
#17692=VERTEX_POINT ( 'NONE', #6646 ) ;
#17697=CARTESIAN_POINT ( 'NONE',  ( 33.46699938050304013, 24.72145308207319303, 47.04930799450050927 ) ) ;
#17698=DIRECTION ( 'NONE',  ( -1.000000000000000000, 0.000000000000000000, 0.000000000000000000 ) ) ;
#17703=CARTESIAN_POINT ( 'NONE',  ( 8.732853799281738105, 28.71183152705961206, 47.04930799450051637 ) ) ;
#17704=AXIS2_PLACEMENT_3D ( 'NONE', #2239, #12423, #102 ) ;
#17706=ORIENTED_EDGE ( 'NONE', *, *, #15474, .T. ) ;
#17707=CARTESIAN_POINT ( 'NONE',  ( 33.50134396954519644, 31.34164230456639544, 47.04930799450051637 ) ) ;
#17715=EDGE_LOOP ( 'NONE', ( #13809, #1058, #15617, #26428 ) ) ;
#17724=LINE ( 'NONE', #10689, #30335 ) ;
#17726=CIRCLE ( 'NONE', #2528, 0.1250000000000001110 ) ;
#17727=AXIS2_PLACEMENT_3D ( 'NONE', #8704, #5925, #18694 ) ;
#17731=TOROIDAL_SURFACE ( 'NONE', #14604, 12.40141737965287838, 0.1249999999999998335 ) ;
#17732=VERTEX_POINT ( 'NONE', #32085 ) ;
#17734=DIRECTION ( 'NONE',  ( -1.101824276508909887E-16, 1.000000000000000000, -0.000000000000000000 ) ) ;
#17751=EDGE_CURVE ( 'NONE', #25197, #5223, #3967, .T. ) ;
#17755=ORIENTED_EDGE ( 'NONE', *, *, #6594, .F. ) ;
#17756=CARTESIAN_POINT ( 'NONE',  ( 8.482002859293444885, 28.71664230456639899, 47.04930799450051637 ) ) ;
#17759=CARTESIAN_POINT ( 'NONE',  ( 33.71785032049135822, 26.46664230456639899, 47.04930799450051637 ) ) ;
#17763=ORIENTED_EDGE ( 'NONE', *, *, #714, .F. ) ;
#17766=CARTESIAN_POINT ( 'NONE',  ( 8.474859994195281132, 38.56284415653841791, 47.04930799450051637 ) ) ;
#17768=ORIENTED_EDGE ( 'NONE', *, *, #7462, .T. ) ;
#17774=DIRECTION ( 'NONE',  ( -1.101824276508909887E-16, 1.000000000000000000, -0.000000000000000000 ) ) ;
#17777=AXIS2_PLACEMENT_3D ( 'NONE', #19629, #19958, #29825 ) ;
#17778=TOROIDAL_SURFACE ( 'NONE', #25140, 12.61792373059861028, 0.1250000000000006106 ) ;
#17783=TOROIDAL_SURFACE ( 'NONE', #9922, 12.40141737965288726, 0.1250000000000003331 ) ;
#17784=DIRECTION ( 'NONE',  ( -1.000000000000000000, 0.000000000000000000, 0.000000000000000000 ) ) ;
#17786=EDGE_CURVE ( 'NONE', #21045, #16795, #8680, .T. ) ;
#17787=DIRECTION ( 'NONE',  ( -1.101824276508909887E-16, 1.000000000000000000, -0.000000000000000000 ) ) ;
#17795=DIRECTION ( 'NONE',  ( -1.000000000000000000, 0.000000000000000000, 0.000000000000000000 ) ) ;
#17796=DIRECTION ( 'NONE',  ( 1.000000000000000000, 0.000000000000000000, 0.000000000000000000 ) ) ;
#17800=VERTEX_POINT ( 'NONE', #31599 ) ;
#17801=CARTESIAN_POINT ( 'NONE',  ( 33.72499318558949710, 24.34143805560860940, 47.04930799450051637 ) ) ;
#17807=TOROIDAL_SURFACE ( 'NONE', #3646, 12.40141737965286062, 0.1249999999999998196 ) ;
#17808=DIRECTION ( 'NONE',  ( -1.224646799147353207E-16, -1.349345573449484691E-32, 1.000000000000000000 ) ) ;
#17809=ORIENTED_EDGE ( 'NONE', *, *, #27201, .F. ) ;
#17810=CARTESIAN_POINT ( 'NONE',  ( 21.09992658989239089, 29.22145308207318237, 47.04930799450051637 ) ) ;
#17811=ORIENTED_EDGE ( 'NONE', *, *, #16661, .F. ) ;
#17814=ORIENTED_EDGE ( 'NONE', *, *, #2395, .T. ) ;
#17815=AXIS2_PLACEMENT_3D ( 'NONE', #5609, #511, #10549 ) ;
#17823=ORIENTED_EDGE ( 'NONE', *, *, #7218, .F. ) ;
#17826=FACE_OUTER_BOUND ( 'NONE', #6482, .T. ) ;
#17827=FACE_OUTER_BOUND ( 'NONE', #25618, .T. ) ;
#17828=EDGE_CURVE ( 'NONE', #18298, #31962, #20197, .T. ) ;
#17843=DIRECTION ( 'NONE',  ( -1.101824276508909887E-16, 1.000000000000000000, -0.000000000000000000 ) ) ;
#17847=AXIS2_PLACEMENT_3D ( 'NONE', #27624, #5310, #13189 ) ;
#17849=ORIENTED_EDGE ( 'NONE', *, *, #26931, .T. ) ;
#17850=AXIS2_PLACEMENT_3D ( 'NONE', #29303, #11749, #26356 ) ;
#17857=EDGE_CURVE ( 'NONE', #7622, #460, #31228, .T. ) ;
#17858=ORIENTED_EDGE ( 'NONE', *, *, #2524, .F. ) ;
#17860=EDGE_CURVE ( 'NONE', #12816, #10473, #22285, .T. ) ;
#17863=AXIS2_PLACEMENT_3D ( 'NONE', #16180, #20633, #10640 ) ;
#17874=EDGE_CURVE ( 'NONE', #2041, #9758, #11819, .T. ) ;
#17877=DIRECTION ( 'NONE',  ( -1.000000000000000000, -1.101824276508909887E-16, 0.000000000000000000 ) ) ;
#17879=VERTEX_POINT ( 'NONE', #17949 ) ;
#17881=CARTESIAN_POINT ( 'NONE',  ( 21.09992658989239089, 26.21183152705960140, 47.04930799450051637 ) ) ;
#17884=LINE ( 'NONE', #27900, #19011 ) ;
#17886=EDGE_LOOP ( 'NONE', ( #22413, #21797, #23759, #24840 ) ) ;
#17894=FACE_OUTER_BOUND ( 'NONE', #8821, .T. ) ;
#17895=AXIS2_PLACEMENT_3D ( 'NONE', #18155, #25874, #10794 ) ;
#17904=FACE_OUTER_BOUND ( 'NONE', #27420, .T. ) ;
#17905=FACE_OUTER_BOUND ( 'NONE', #4844, .T. ) ;
#17907=AXIS2_PLACEMENT_3D ( 'NONE', #20097, #4678, #7640 ) ;
#17916=CARTESIAN_POINT ( 'NONE',  ( 21.09992658989239089, 27.09164230456639899, 47.04930799450051637 ) ) ;
#17917=DIRECTION ( 'NONE',  ( -1.101824276508909887E-16, 1.000000000000000000, -0.000000000000000000 ) ) ;
#17920=ORIENTED_EDGE ( 'NONE', *, *, #256, .F. ) ;
#17923=DIRECTION ( 'NONE',  ( -1.101824276508909887E-16, 1.000000000000000000, -0.000000000000000000 ) ) ;
#17925=DIRECTION ( 'NONE',  ( -1.000000000000000000, -1.101824276508909887E-16, 0.000000000000000000 ) ) ;
#17930=ORIENTED_EDGE ( 'NONE', *, *, #9993, .T. ) ;
#17938=EDGE_CURVE ( 'NONE', #4682, #25773, #15494, .T. ) ;
#17940=ADVANCED_FACE ( 'NONE', ( #30116 ), #31733, .T. ) ;
#17941=CARTESIAN_POINT ( 'NONE',  ( 21.09992658989239089, 26.59164230456639899, 47.04930799450051637 ) ) ;
#17944=CIRCLE ( 'NONE', #23193, 0.1250000000000001110 ) ;
#17946=FACE_OUTER_BOUND ( 'NONE', #22473, .T. ) ;
#17949=CARTESIAN_POINT ( 'NONE',  ( 8.732853799281732776, 31.72145308207317171, 47.04930799450051637 ) ) ;
#17950=CARTESIAN_POINT ( 'NONE',  ( 33.46699938050304013, 26.96183152705960495, 47.04930799450051637 ) ) ;
#17955=ORIENTED_EDGE ( 'NONE', *, *, #17286, .F. ) ;
#17956=DIRECTION ( 'NONE',  ( -1.101824276508909887E-16, 1.000000000000000000, -0.000000000000000000 ) ) ;
#17960=DIRECTION ( 'NONE',  ( -1.101824276508909887E-16, 1.000000000000000000, -0.000000000000000000 ) ) ;
#17965=DIRECTION ( 'NONE',  ( -1.000000000000000000, 0.000000000000000000, 0.000000000000000000 ) ) ;
#17969=AXIS2_PLACEMENT_3D ( 'NONE', #477, #8045, #18034 ) ;
#17972=ORIENTED_EDGE ( 'NONE', *, *, #22450, .T. ) ;
#17974=ORIENTED_EDGE ( 'NONE', *, *, #7856, .T. ) ;
#17978=VECTOR ( 'NONE', #6507, 1000.000000000000000 ) ;
#17984=ORIENTED_EDGE ( 'NONE', *, *, #23669, .T. ) ;
#17987=DIRECTION ( 'NONE',  ( -1.000000000000000000, 0.000000000000000000, 0.000000000000000000 ) ) ;
#17990=VECTOR ( 'NONE', #8191, 1000.000000000000000 ) ;
#17991=CARTESIAN_POINT ( 'NONE',  ( 21.09992658989239089, 29.09184655352418858, 47.04930799450051637 ) ) ;
#17993=DIRECTION ( 'NONE',  ( -1.000000000000000000, 0.000000000000000000, 0.000000000000000000 ) ) ;
#18004=DIRECTION ( 'NONE',  ( -1.101824276508909887E-16, 1.000000000000000000, -0.000000000000000000 ) ) ;
#18005=VECTOR ( 'NONE', #8999, 1000.000000000000000 ) ;
#18006=DIRECTION ( 'NONE',  ( -1.101824276508909887E-16, 1.000000000000000000, -0.000000000000000000 ) ) ;
#18007=DIRECTION ( 'NONE',  ( -1.101824276508909887E-16, 1.000000000000000000, -0.000000000000000000 ) ) ;
#18010=ADVANCED_FACE ( 'NONE', ( #26139 ), #7632, .T. ) ;
#18013=ORIENTED_EDGE ( 'NONE', *, *, #23351, .T. ) ;
#18014=ORIENTED_EDGE ( 'NONE', *, *, #19552, .T. ) ;
#18015=DIRECTION ( 'NONE',  ( -1.101824276508909887E-16, 1.000000000000000000, -0.000000000000000000 ) ) ;
#18018=EDGE_CURVE ( 'NONE', #21770, #30824, #28594, .T. ) ;
#18022=ORIENTED_EDGE ( 'NONE', *, *, #31628, .F. ) ;
#18025=ADVANCED_FACE ( 'NONE', ( #5972 ), #23520, .F. ) ;
#18027=ORIENTED_EDGE ( 'NONE', *, *, #28504, .F. ) ;
#18032=CARTESIAN_POINT ( 'NONE',  ( 8.482002859293428898, 27.21664230456639899, 47.04930799450051637 ) ) ;
#18034=DIRECTION ( 'NONE',  ( -1.000000000000000000, 0.000000000000000000, 0.000000000000000000 ) ) ;
#18035=VECTOR ( 'NONE', #21850, 1000.000000000000000 ) ;
#18041=CIRCLE ( 'NONE', #31684, 12.62506659569710266 ) ;
#18042=DIRECTION ( 'NONE',  ( -1.101824276508909887E-16, 1.000000000000000000, -0.000000000000000000 ) ) ;
#18047=DIRECTION ( 'NONE',  ( -1.000000000000000000, 0.000000000000000000, 0.000000000000000000 ) ) ;
#18049=CARTESIAN_POINT ( 'NONE',  ( 21.09992658989238734, 30.72145308207317882, 47.04930799450051637 ) ) ;
#18052=ORIENTED_EDGE ( 'NONE', *, *, #22476, .F. ) ;
#18059=CARTESIAN_POINT ( 'NONE',  ( 21.09992658989238734, 32.21183152705962272, 47.04930799450051637 ) ) ;
#18060=VECTOR ( 'NONE', #763, 1000.000000000000000 ) ;
#18062=AXIS2_PLACEMENT_3D ( 'NONE', #17239, #2157, #24468 ) ;
#18065=DIRECTION ( 'NONE',  ( -1.000000000000000000, 0.000000000000000000, 0.000000000000000000 ) ) ;
#18073=CARTESIAN_POINT ( 'NONE',  ( 21.09992658989239089, 27.97145308207318237, 47.04930799450051637 ) ) ;
#18085=CARTESIAN_POINT ( 'NONE',  ( 33.46699938050303302, 38.56284415653841791, 47.04930799450051637 ) ) ;
#18088=ORIENTED_EDGE ( 'NONE', *, *, #20403, .F. ) ;
#18096=EDGE_LOOP ( 'NONE', ( #8110, #19584, #23115, #1597 ) ) ;
#18104=CIRCLE ( 'NONE', #22299, 0.1249999999999983763 ) ;
#18111=CARTESIAN_POINT ( 'NONE',  ( 21.09992658989239089, 26.09164230456639899, 47.04930799450051637 ) ) ;
#18116=EDGE_CURVE ( 'NONE', #9970, #24538, #8173, .T. ) ;
#18117=DIRECTION ( 'NONE',  ( -1.101824276508909887E-16, 1.000000000000000000, -0.000000000000000000 ) ) ;
#18131=ORIENTED_EDGE ( 'NONE', *, *, #20888, .T. ) ;
#18133=VERTEX_POINT ( 'NONE', #29420 ) ;
#18134=CIRCLE ( 'NONE', #7128, 12.36707279061065101 ) ;
#18136=FACE_OUTER_BOUND ( 'NONE', #4696, .T. ) ;
#18155=CARTESIAN_POINT ( 'NONE',  ( 21.09992658989239089, 27.59164230456639544, 47.04930799450051637 ) ) ;
#18157=EDGE_CURVE ( 'NONE', #28443, #31932, #18041, .T. ) ;
#18161=CARTESIAN_POINT ( 'NONE',  ( 21.09992658989238734, 38.56284415653841791, 47.04930799450051637 ) ) ;
#18163=ADVANCED_FACE ( 'NONE', ( #24320 ), #13858, .T. ) ;
#18164=ADVANCED_FACE ( 'NONE', ( #14000 ), #17532, .T. ) ;
#18165=ORIENTED_EDGE ( 'NONE', *, *, #17597, .T. ) ;
#18166=DIRECTION ( 'NONE',  ( -1.000000000000000000, 0.000000000000000000, 0.000000000000000000 ) ) ;
#18168=DIRECTION ( 'NONE',  ( -1.000000000000000000, 0.000000000000000000, 0.000000000000000000 ) ) ;
#18172=ORIENTED_EDGE ( 'NONE', *, *, #19982, .T. ) ;
#18177=ORIENTED_EDGE ( 'NONE', *, *, #10951, .T. ) ;
#18180=DIRECTION ( 'NONE',  ( -1.000000000000000000, -1.101824276508909887E-16, 0.000000000000000000 ) ) ;
#18182=ORIENTED_EDGE ( 'NONE', *, *, #7039, .T. ) ;
#18190=CARTESIAN_POINT ( 'NONE',  ( 33.72499318558949710, 24.59184655352419213, 47.04930799450051637 ) ) ;
#18194=CARTESIAN_POINT ( 'NONE',  ( 21.09992658989239089, 28.71664230456639899, 47.04930799450051637 ) ) ;
#18202=CARTESIAN_POINT ( 'NONE',  ( 21.09992658989238734, 38.56284415653841791, 47.04930799450051637 ) ) ;
#18204=EDGE_CURVE ( 'NONE', #22382, #5329, #18566, .T. ) ;
#18207=DIRECTION ( 'NONE',  ( -1.224646799147353207E-16, -1.349345573449484691E-32, 1.000000000000000000 ) ) ;
#18212=EDGE_CURVE ( 'NONE', #19026, #23509, #9215, .T. ) ;
#18215=DIRECTION ( 'NONE',  ( -1.101824276508909887E-16, 1.000000000000000000, -0.000000000000000000 ) ) ;
#18217=DIRECTION ( 'NONE',  ( -1.101824276508909887E-16, 1.000000000000000000, -0.000000000000000000 ) ) ;
#18218=CARTESIAN_POINT ( 'NONE',  ( 33.50134396954522487, 28.59164230456639544, 47.04930799450051637 ) ) ;
#18220=DIRECTION ( 'NONE',  ( -1.101824276508909887E-16, 1.000000000000000000, -0.000000000000000000 ) ) ;
#18221=VECTOR ( 'NONE', #10252, 1000.000000000000000 ) ;
#18230=CARTESIAN_POINT ( 'NONE',  ( 21.09992658989239089, 26.84164230456639899, 47.04930799450051637 ) ) ;
#18232=FACE_OUTER_BOUND ( 'NONE', #19929, .T. ) ;
#18234=FACE_OUTER_BOUND ( 'NONE', #15552, .T. ) ;
#18248=DIRECTION ( 'NONE',  ( -1.000000000000000000, 0.000000000000000000, 0.000000000000000000 ) ) ;
#18249=CARTESIAN_POINT ( 'NONE',  ( 8.698509210239528500, 26.34164230456639899, 47.04930799450051637 ) ) ;
#18252=ADVANCED_FACE ( 'NONE', ( #17422 ), #2656, .T. ) ;
#18255=CARTESIAN_POINT ( 'NONE',  ( 8.474859994195282908, 38.56284415653841791, 47.04930799450051637 ) ) ;
#18260=AXIS2_PLACEMENT_3D ( 'NONE', #11030, #3628, #30891 ) ;
#18261=CARTESIAN_POINT ( 'NONE',  ( 8.732853799281734553, 38.56284415653841791, 47.04930799450051637 ) ) ;
#18264=AXIS2_PLACEMENT_3D ( 'NONE', #19611, #17314, #31937 ) ;
#18268=CARTESIAN_POINT ( 'NONE',  ( 21.09992658989239089, 25.47145308207319303, 47.04930799450051637 ) ) ;
#18270=DIRECTION ( 'NONE',  ( 0.000000000000000000, -0.000000000000000000, -1.000000000000000000 ) ) ;
#18272=AXIS2_PLACEMENT_3D ( 'NONE', #3788, #31370, #28585 ) ;
#18276=CARTESIAN_POINT ( 'NONE',  ( 21.09992658989239089, 24.59164230456639544, 47.04930799450051637 ) ) ;
#18278=ORIENTED_EDGE ( 'NONE', *, *, #24308, .T. ) ;
#18281=DIRECTION ( 'NONE',  ( 0.000000000000000000, -0.000000000000000000, -1.000000000000000000 ) ) ;
#18289=EDGE_CURVE ( 'NONE', #3113, #10702, #12294, .T. ) ;
#18290=EDGE_LOOP ( 'NONE', ( #5220, #7316, #6495, #11373 ) ) ;
#18292=AXIS2_PLACEMENT_3D ( 'NONE', #22963, #22648, #20185 ) ;
#18298=VERTEX_POINT ( 'NONE', #29915 ) ;
#18304=LINE ( 'NONE', #10785, #17339 ) ;
#18305=ORIENTED_EDGE ( 'NONE', *, *, #13469, .T. ) ;
#18306=DIRECTION ( 'NONE',  ( -1.101824276508909887E-16, 1.000000000000000000, -0.000000000000000000 ) ) ;
#18312=CARTESIAN_POINT ( 'NONE',  ( 8.482002859293448438, 28.96664230456639899, 47.04930799450051637 ) ) ;
#18321=ORIENTED_EDGE ( 'NONE', *, *, #2994, .F. ) ;
#18322=DIRECTION ( 'NONE',  ( -1.224646799147353207E-16, -1.349345573449484691E-32, 1.000000000000000000 ) ) ;
#18324=AXIS2_PLACEMENT_3D ( 'NONE', #9253, #21223, #24018 ) ;
#18327=TOROIDAL_SURFACE ( 'NONE', #11511, 12.61792373059891226, 0.1250000000000024980 ) ;
#18329=CARTESIAN_POINT ( 'NONE',  ( 21.09992658989238734, 38.56284415653841791, 47.04930799450051637 ) ) ;
#18333=AXIS2_PLACEMENT_3D ( 'NONE', #6120, #25818, #11059 ) ;
#18343=CIRCLE ( 'NONE', #3140, 0.1250000000000001110 ) ;
#18347=AXIS2_PLACEMENT_3D ( 'NONE', #27031, #14892, #10296 ) ;
#18348=ORIENTED_EDGE ( 'NONE', *, *, #28913, .T. ) ;
#18353=CARTESIAN_POINT ( 'NONE',  ( 33.37634396954525329, 26.34164230456639899, 47.04930799450051637 ) ) ;
#18357=CARTESIAN_POINT ( 'NONE',  ( 8.482002859293777064, 30.96664230456641675, 47.04930799450051637 ) ) ;
#18362=CARTESIAN_POINT ( 'NONE',  ( 8.823509210239542710, 27.59164230456639544, 47.04930799450051637 ) ) ;
#18364=EDGE_CURVE ( 'NONE', #6807, #22128, #10729, .T. ) ;
#18368=AXIS2_PLACEMENT_3D ( 'NONE', #27850, #20932, #30964 ) ;
#18370=VECTOR ( 'NONE', #8486, 1000.000000000000000 ) ;
#18378=DIRECTION ( 'NONE',  ( -1.000000000000000000, -1.101824276508909887E-16, 0.000000000000000000 ) ) ;
#18385=EDGE_LOOP ( 'NONE', ( #27998, #27064, #24776, #27903 ) ) ;
#18386=FACE_OUTER_BOUND ( 'NONE', #13072, .T. ) ;
#18389=FACE_OUTER_BOUND ( 'NONE', #25105, .T. ) ;
#18391=CARTESIAN_POINT ( 'NONE',  ( 21.09992658989239089, 23.59164230456639544, 47.04930799450051637 ) ) ;
#18392=CIRCLE ( 'NONE', #28368, 12.36707279061065101 ) ;
#18401=DIRECTION ( 'NONE',  ( -1.000000000000000000, 0.000000000000000000, 0.000000000000000000 ) ) ;
#18403=DIRECTION ( 'NONE',  ( -1.000000000000000000, 0.000000000000000000, 0.000000000000000000 ) ) ;
#18410=CARTESIAN_POINT ( 'NONE',  ( 33.46699938050304723, 26.22145308207318593, 47.04930799450050927 ) ) ;
#18411=ORIENTED_EDGE ( 'NONE', *, *, #27802, .T. ) ;
#18414=VECTOR ( 'NONE', #7436, 1000.000000000000000 ) ;
#18418=EDGE_LOOP ( 'NONE', ( #21051, #29314, #30297, #12677 ) ) ;
#18426=CARTESIAN_POINT ( 'NONE',  ( 33.72499318558949710, 25.34143805560860940, 47.04930799450051637 ) ) ;
#18427=EDGE_CURVE ( 'NONE', #21045, #21064, #29074, .T. ) ;
#18432=FACE_OUTER_BOUND ( 'NONE', #16366, .T. ) ;
#18434=CARTESIAN_POINT ( 'NONE',  ( 21.09992658989238734, 38.56284415653841791, 47.04930799450051637 ) ) ;
#18436=DIRECTION ( 'NONE',  ( -1.000000000000000000, 0.000000000000000000, 0.000000000000000000 ) ) ;
#18441=DIRECTION ( 'NONE',  ( -1.101824276508909887E-16, 1.000000000000000000, -0.000000000000000000 ) ) ;
#18443=ORIENTED_EDGE ( 'NONE', *, *, #20720, .T. ) ;
#18444=CYLINDRICAL_SURFACE ( 'NONE', #15230, 12.62506659569710266 ) ;
#18445=DIRECTION ( 'NONE',  ( -1.101824276508909887E-16, 1.000000000000000000, -0.000000000000000000 ) ) ;
#18446=EDGE_CURVE ( 'NONE', #4539, #24404, #19096, .T. ) ;
#18451=EDGE_LOOP ( 'NONE', ( #25416, #31587, #29696, #29385 ) ) ;
#18452=CARTESIAN_POINT ( 'NONE',  ( 8.474859994195259816, 23.84143805560861296, 47.04930799450051637 ) ) ;
#18454=AXIS2_PLACEMENT_3D ( 'NONE', #22726, #15503, #12897 ) ;
#18465=ORIENTED_EDGE ( 'NONE', *, *, #7462, .F. ) ;
#18472=FACE_OUTER_BOUND ( 'NONE', #21614, .T. ) ;
#18475=ORIENTED_EDGE ( 'NONE', *, *, #7124, .F. ) ;
#18480=CIRCLE ( 'NONE', #2750, 0.1250000000000001110 ) ;
#18482=ORIENTED_EDGE ( 'NONE', *, *, #16074, .F. ) ;
#18487=DIRECTION ( 'NONE',  ( -1.101824276508909887E-16, 1.000000000000000000, -0.000000000000000000 ) ) ;
#18489=DIRECTION ( 'NONE',  ( -1.101824276508909887E-16, 1.000000000000000000, -0.000000000000000000 ) ) ;
#18491=ORIENTED_EDGE ( 'NONE', *, *, #28279, .T. ) ;
#18492=AXIS2_PLACEMENT_3D ( 'NONE', #11597, #9290, #19458 ) ;
#18493=VERTEX_POINT ( 'NONE', #9481 ) ;
#18494=DIRECTION ( 'NONE',  ( -1.101824276508909887E-16, 1.000000000000000000, -0.000000000000000000 ) ) ;
#18497=VERTEX_POINT ( 'NONE', #19145 ) ;
#18502=AXIS2_PLACEMENT_3D ( 'NONE', #10279, #24718, #2229 ) ;
#18504=DIRECTION ( 'NONE',  ( 1.000000000000000000, 0.000000000000000000, 0.000000000000000000 ) ) ;
#18505=CARTESIAN_POINT ( 'NONE',  ( 8.474859994195281132, 38.56284415653841791, 47.04930799450051637 ) ) ;
#18508=ORIENTED_EDGE ( 'NONE', *, *, #6896, .T. ) ;
#18509=ORIENTED_EDGE ( 'NONE', *, *, #30868, .F. ) ;
#18515=DIRECTION ( 'NONE',  ( -1.224646799147353207E-16, -1.349345573449484691E-32, 1.000000000000000000 ) ) ;
#18520=EDGE_CURVE ( 'NONE', #3113, #18497, #14932, .T. ) ;
#18522=CIRCLE ( 'NONE', #7533, 12.36707279061065101 ) ;
#18525=ORIENTED_EDGE ( 'NONE', *, *, #30991, .T. ) ;
#18526=CARTESIAN_POINT ( 'NONE',  ( 21.09992658989239089, 27.22145308207318593, 47.04930799450051637 ) ) ;
#18529=EDGE_LOOP ( 'NONE', ( #15929, #95, #3472, #1378 ) ) ;
#18532=ORIENTED_EDGE ( 'NONE', *, *, #31832, .F. ) ;
#18545=DIRECTION ( 'NONE',  ( -1.000000000000000000, 0.000000000000000000, 0.000000000000000000 ) ) ;
#18547=ORIENTED_EDGE ( 'NONE', *, *, #4942, .F. ) ;
#18549=DIRECTION ( 'NONE',  ( -1.224646799147353207E-16, -1.349345573449484691E-32, 1.000000000000000000 ) ) ;
#18550=DIRECTION ( 'NONE',  ( -1.000000000000000000, 0.000000000000000000, 0.000000000000000000 ) ) ;
#18551=EDGE_CURVE ( 'NONE', #32344, #14664, #19621, .T. ) ;
#18552=DIRECTION ( 'NONE',  ( -1.101824276508909887E-16, 1.000000000000000000, -0.000000000000000000 ) ) ;
#18558=EDGE_CURVE ( 'NONE', #18497, #15900, #28566, .T. ) ;
#18561=EDGE_CURVE ( 'NONE', #17732, #2041, #26450, .T. ) ;
#18566=CIRCLE ( 'NONE', #21714, 0.1250000000000001110 ) ;
#18567=AXIS2_PLACEMENT_3D ( 'NONE', #19539, #14630, #7075 ) ;
#18573=ORIENTED_EDGE ( 'NONE', *, *, #1294, .F. ) ;
#18577=DIRECTION ( 'NONE',  ( -1.101824276508909887E-16, 1.000000000000000000, -0.000000000000000000 ) ) ;
#18578=VERTEX_POINT ( 'NONE', #24736 ) ;
#18587=DIRECTION ( 'NONE',  ( -1.101824276508909887E-16, 1.000000000000000000, -0.000000000000000000 ) ) ;
#18588=CARTESIAN_POINT ( 'NONE',  ( 8.474859994195286461, 24.09143805560860940, 47.04930799450051637 ) ) ;
#18590=DIRECTION ( 'NONE',  ( -1.101824276508909887E-16, 1.000000000000000000, -0.000000000000000000 ) ) ;
#18591=DIRECTION ( 'NONE',  ( -1.101824276508909887E-16, 1.000000000000000000, -0.000000000000000000 ) ) ;
#18600=DIRECTION ( 'NONE',  ( -1.101824276508909887E-16, 1.000000000000000000, -0.000000000000000000 ) ) ;
#18601=CARTESIAN_POINT ( 'NONE',  ( 33.46699938050304013, 24.46183152705960140, 47.04930799450051637 ) ) ;
#18607=AXIS2_PLACEMENT_3D ( 'NONE', #21606, #28681, #18504 ) ;
#18611=VECTOR ( 'NONE', #32049, 1000.000000000000000 ) ;
#18612=EDGE_CURVE ( 'NONE', #9970, #15217, #21728, .T. ) ;
#18616=CARTESIAN_POINT ( 'NONE',  ( 21.09992658989239089, 24.71664230456639899, 47.04930799450051637 ) ) ;
#18619=CIRCLE ( 'NONE', #10812, 12.36707279061065279 ) ;
#18621=DIRECTION ( 'NONE',  ( -1.101824276508909887E-16, 1.000000000000000000, -0.000000000000000000 ) ) ;
#18623=CARTESIAN_POINT ( 'NONE',  ( 21.09992658989238734, 38.56284415653841791, 47.04930799450051637 ) ) ;
#18626=ORIENTED_EDGE ( 'NONE', *, *, #26677, .T. ) ;
#18633=DIRECTION ( 'NONE',  ( -1.000000000000000000, -1.101824276508910010E-16, 0.000000000000000000 ) ) ;
#18635=DIRECTION ( 'NONE',  ( -1.101824276508909887E-16, 1.000000000000000000, -0.000000000000000000 ) ) ;
#18638=CARTESIAN_POINT ( 'NONE',  ( 33.72499318558949710, 24.34184655352419213, 47.04930799450051637 ) ) ;
#18640=EDGE_CURVE ( 'NONE', #14790, #11991, #20685, .T. ) ;
#18642=AXIS2_PLACEMENT_3D ( 'NONE', #8595, #13689, #25984 ) ;
#18647=CIRCLE ( 'NONE', #8182, 12.36707279061065101 ) ;
#18653=DIRECTION ( 'NONE',  ( -1.101824276508909887E-16, 1.000000000000000000, -0.000000000000000000 ) ) ;
#18658=ADVANCED_FACE ( 'NONE', ( #5528 ), #31174, .T. ) ;
#18663=ORIENTED_EDGE ( 'NONE', *, *, #13633, .T. ) ;
#18667=DIRECTION ( 'NONE',  ( -1.000000000000000000, 0.000000000000000000, 0.000000000000000000 ) ) ;
#18677=DIRECTION ( 'NONE',  ( -1.000000000000000000, 0.000000000000000000, 0.000000000000000000 ) ) ;
#18678=CARTESIAN_POINT ( 'NONE',  ( 33.50134396954523197, 28.34164230456639544, 47.04930799450051637 ) ) ;
#18679=DIRECTION ( 'NONE',  ( -1.000000000000000000, -1.101824276508909887E-16, 0.000000000000000000 ) ) ;
#18680=EDGE_LOOP ( 'NONE', ( #19100, #181, #21816, #333 ) ) ;
#18687=EDGE_CURVE ( 'NONE', #9226, #1319, #25409, .T. ) ;
#18691=CARTESIAN_POINT ( 'NONE',  ( 21.09992658989238734, 38.56284415653841791, 47.04930799450051637 ) ) ;
#18692=EDGE_CURVE ( 'NONE', #19345, #10922, #1280, .T. ) ;
#18694=DIRECTION ( 'NONE',  ( -1.000000000000000000, 0.000000000000000000, 0.000000000000000000 ) ) ;
#18696=LINE ( 'NONE', #5601, #4337 ) ;
#18697=AXIS2_PLACEMENT_3D ( 'NONE', #17524, #12124, #17355 ) ;
#18699=LINE ( 'NONE', #3777, #10356 ) ;
#18704=ORIENTED_EDGE ( 'NONE', *, *, #13439, .F. ) ;
#18705=ORIENTED_EDGE ( 'NONE', *, *, #28933, .F. ) ;
#18713=DIRECTION ( 'NONE',  ( -1.000000000000000000, -1.101824276508910010E-16, 0.000000000000000000 ) ) ;
#18716=AXIS2_PLACEMENT_3D ( 'NONE', #22991, #7586, #12517 ) ;
#18717=CIRCLE ( 'NONE', #2481, 12.62506659569710443 ) ;
#18720=VECTOR ( 'NONE', #1127, 1000.000000000000000 ) ;
#18721=DIRECTION ( 'NONE',  ( -1.000000000000000000, 0.000000000000000000, 0.000000000000000000 ) ) ;
#18727=EDGE_CURVE ( 'NONE', #5329, #12476, #15691, .T. ) ;
#18733=EDGE_CURVE ( 'NONE', #21016, #1311, #27016, .T. ) ;
#18737=CARTESIAN_POINT ( 'NONE',  ( 8.698509210239526723, 26.09164230456639899, 47.04930799450051637 ) ) ;
#18744=VECTOR ( 'NONE', #13245, 1000.000000000000000 ) ;
#18745=CARTESIAN_POINT ( 'NONE',  ( 21.09992658989239089, 24.96664230456639899, 47.04930799450051637 ) ) ;
#18749=VERTEX_POINT ( 'NONE', #3865 ) ;
#18752=FACE_OUTER_BOUND ( 'NONE', #24294, .T. ) ;
#18755=DIRECTION ( 'NONE',  ( -1.101824276508909887E-16, 1.000000000000000000, -0.000000000000000000 ) ) ;
#18761=ORIENTED_EDGE ( 'NONE', *, *, #25215, .F. ) ;
#18764=AXIS2_PLACEMENT_3D ( 'NONE', #17941, #30592, #22371 ) ;
#18767=EDGE_CURVE ( 'NONE', #12476, #28743, #32250, .T. ) ;
#18773=EDGE_CURVE ( 'NONE', #2250, #16708, #13395, .T. ) ;
#18775=AXIS2_PLACEMENT_3D ( 'NONE', #30893, #13495, #18401 ) ;
#18780=DIRECTION ( 'NONE',  ( 1.000000000000000000, 0.000000000000000000, 0.000000000000000000 ) ) ;
#18784=DIRECTION ( 'NONE',  ( -1.000000000000000000, -1.101824276508910010E-16, 0.000000000000000000 ) ) ;
#18787=CYLINDRICAL_SURFACE ( 'NONE', #24133, 12.36707279061065101 ) ;
#18789=CARTESIAN_POINT ( 'NONE',  ( 21.09992658989239089, 28.09164230456639544, 47.04930799450051637 ) ) ;
#18790=ORIENTED_EDGE ( 'NONE', *, *, #22715, .T. ) ;
#18796=CIRCLE ( 'NONE', #19865, 0.1250000000000018319 ) ;
#18799=ORIENTED_EDGE ( 'NONE', *, *, #992, .T. ) ;
#18801=EDGE_CURVE ( 'NONE', #112, #14283, #9185, .T. ) ;
#18807=CIRCLE ( 'NONE', #31425, 0.1250000000000001110 ) ;
#18808=TOROIDAL_SURFACE ( 'NONE', #19363, 12.40141737965284463, 0.1250000000000005274 ) ;
#18809=ORIENTED_EDGE ( 'NONE', *, *, #16881, .T. ) ;
#18811=DIRECTION ( 'NONE',  ( -1.000000000000000000, 0.000000000000000000, 0.000000000000000000 ) ) ;
#18815=ORIENTED_EDGE ( 'NONE', *, *, #19441, .T. ) ;
#18816=ORIENTED_EDGE ( 'NONE', *, *, #7379, .T. ) ;
#18817=CARTESIAN_POINT ( 'NONE',  ( 21.09992658989239089, 26.47145308207318593, 47.04930799450051637 ) ) ;
#18821=AXIS2_PLACEMENT_3D ( 'NONE', #13231, #18281, #28315 ) ;
#18824=CARTESIAN_POINT ( 'NONE',  ( 8.482002859293471531, 31.71664230456639544, 47.04930799450051637 ) ) ;
#18826=CIRCLE ( 'NONE', #13607, 0.1250000000000001110 ) ;
#18829=EDGE_CURVE ( 'NONE', #31159, #1392, #7078, .T. ) ;
#18830=ORIENTED_EDGE ( 'NONE', *, *, #1746, .F. ) ;
#18831=CYLINDRICAL_SURFACE ( 'NONE', #6635, 12.36707279061065101 ) ;
#18834=DIRECTION ( 'NONE',  ( -1.000000000000000000, 0.000000000000000000, 0.000000000000000000 ) ) ;
#18837=CARTESIAN_POINT ( 'NONE',  ( 21.09992658989239089, 23.84164230456639544, 47.04930799450051637 ) ) ;
#18842=FACE_OUTER_BOUND ( 'NONE', #22546, .T. ) ;
#18848=AXIS2_PLACEMENT_3D ( 'NONE', #1269, #26059, #6207 ) ;
#18854=AXIS2_PLACEMENT_3D ( 'NONE', #11876, #27131, #31741 ) ;
#18859=DIRECTION ( 'NONE',  ( -1.224646799147353207E-16, -1.349345573449484691E-32, 1.000000000000000000 ) ) ;
#18863=CIRCLE ( 'NONE', #29907, 0.1250000000000001110 ) ;
#18867=CARTESIAN_POINT ( 'NONE',  ( 21.09992658989238734, 30.96664230456641675, 47.04930799450051637 ) ) ;
#18869=ORIENTED_EDGE ( 'NONE', *, *, #31391, .T. ) ;
#18871=CARTESIAN_POINT ( 'NONE',  ( 21.09992658989239089, 28.34164230456639544, 47.04930799450051637 ) ) ;
#18874=EDGE_CURVE ( 'NONE', #15187, #3444, #2218, .T. ) ;
#18877=CARTESIAN_POINT ( 'NONE',  ( 33.46699938050302592, 32.47145308207318237, 47.04930799450050927 ) ) ;
#18881=AXIS2_PLACEMENT_3D ( 'NONE', #24900, #25224, #9639 ) ;
#18884=CIRCLE ( 'NONE', #31482, 12.27641737965286239 ) ;
#18885=EDGE_CURVE ( 'NONE', #30931, #14214, #30176, .T. ) ;
#18887=EDGE_CURVE ( 'NONE', #3483, #32275, #16513, .T. ) ;
#18889=ORIENTED_EDGE ( 'NONE', *, *, #17751, .T. ) ;
#18890=CARTESIAN_POINT ( 'NONE',  ( 21.09992658989239089, 29.34164230456639899, 47.04930799450051637 ) ) ;
#18898=DIRECTION ( 'NONE',  ( -1.101824276508909887E-16, 1.000000000000000000, -0.000000000000000000 ) ) ;
#18905=DIRECTION ( 'NONE',  ( -1.101824276508909887E-16, 1.000000000000000000, -0.000000000000000000 ) ) ;
#18907=ORIENTED_EDGE ( 'NONE', *, *, #24446, .T. ) ;
#18908=DIRECTION ( 'NONE',  ( -1.101824276508909887E-16, 1.000000000000000000, -0.000000000000000000 ) ) ;
#18911=CARTESIAN_POINT ( 'NONE',  ( 33.37634396954521065, 30.09164230456639544, 47.04930799450051637 ) ) ;
#18912=FACE_OUTER_BOUND ( 'NONE', #27714, .T. ) ;
#18913=CARTESIAN_POINT ( 'NONE',  ( 21.09992658989239089, 25.84143805560860940, 47.04930799450051637 ) ) ;
#18920=FACE_OUTER_BOUND ( 'NONE', #696, .T. ) ;
#18922=ADVANCED_FACE ( 'NONE', ( #24210 ), #10255, .T. ) ;
#18924=ORIENTED_EDGE ( 'NONE', *, *, #30909, .F. ) ;
#18926=ORIENTED_EDGE ( 'NONE', *, *, #7613, .T. ) ;
#18927=TOROIDAL_SURFACE ( 'NONE', #12684, 12.40141737965281088, 0.1249999999999987788 ) ;
#18934=FACE_OUTER_BOUND ( 'NONE', #24324, .T. ) ;
#18935=CARTESIAN_POINT ( 'NONE',  ( 8.474859994195286461, 25.59184655352419213, 47.04930799450051637 ) ) ;
#18938=ORIENTED_EDGE ( 'NONE', *, *, #14475, .T. ) ;
#18943=ORIENTED_EDGE ( 'NONE', *, *, #21858, .F. ) ;
#18944=DIRECTION ( 'NONE',  ( -1.000000000000000000, 0.000000000000000000, 0.000000000000000000 ) ) ;
#18950=DIRECTION ( 'NONE',  ( -1.101824276508909887E-16, 1.000000000000000000, -0.000000000000000000 ) ) ;
#18951=DIRECTION ( 'NONE',  ( 1.000000000000000000, 0.000000000000000000, 0.000000000000000000 ) ) ;
#18955=CARTESIAN_POINT ( 'NONE',  ( 33.46699938050304013, 24.21183152705959785, 47.04930799450051637 ) ) ;
#18959=CARTESIAN_POINT ( 'NONE',  ( 21.09992658989239089, 29.09164230456639899, 47.04930799450051637 ) ) ;
#18968=ORIENTED_EDGE ( 'NONE', *, *, #11049, .T. ) ;
#18969=AXIS2_PLACEMENT_3D ( 'NONE', #18678, #5306, #21301 ) ;
#18974=AXIS2_PLACEMENT_3D ( 'NONE', #26431, #4273, #31843 ) ;
#18975=FACE_OUTER_BOUND ( 'NONE', #21462, .T. ) ;
#18976=CARTESIAN_POINT ( 'NONE',  ( 8.474859994195286461, 28.09143805560861296, 47.04930799450051637 ) ) ;
#18978=CIRCLE ( 'NONE', #3279, 12.62506659569710266 ) ;
#18985=EDGE_LOOP ( 'NONE', ( #15888, #8040, #29681, #17310 ) ) ;
#18987=VECTOR ( 'NONE', #10790, 1000.000000000000000 ) ;
#18988=LINE ( 'NONE', #1001, #9497 ) ;
#18990=CARTESIAN_POINT ( 'NONE',  ( 21.09992658989238734, 38.56284415653841791, 47.04930799450051637 ) ) ;
#18991=LINE ( 'NONE', #4889, #10657 ) ;
#18993=VECTOR ( 'NONE', #8969, 1000.000000000000000 ) ;
#18994=CARTESIAN_POINT ( 'NONE',  ( 33.72499318558949710, 32.09143805560860585, 47.04930799450051637 ) ) ;
#18995=CARTESIAN_POINT ( 'NONE',  ( 33.37634396954526039, 25.34164230456639899, 47.04930799450051637 ) ) ;
#19001=DIRECTION ( 'NONE',  ( -1.101824276508909887E-16, 1.000000000000000000, -0.000000000000000000 ) ) ;
#19004=EDGE_LOOP ( 'NONE', ( #30426, #3260, #5721, #6790 ) ) ;
#19006=EDGE_CURVE ( 'NONE', #29925, #12345, #3938, .T. ) ;
#19008=AXIS2_PLACEMENT_3D ( 'NONE', #32464, #27371, #24912 ) ;
#19009=VECTOR ( 'NONE', #5892, 1000.000000000000000 ) ;
#19011=VECTOR ( 'NONE', #5416, 1000.000000000000000 ) ;
#19015=LINE ( 'NONE', #29044, #15505 ) ;
#19017=ADVANCED_FACE ( 'NONE', ( #12563 ), #17305, .F. ) ;
#19023=ORIENTED_EDGE ( 'NONE', *, *, #8709, .T. ) ;
#19025=EDGE_CURVE ( 'NONE', #28135, #27014, #13907, .T. ) ;
#19026=VERTEX_POINT ( 'NONE', #17632 ) ;
#19028=DIRECTION ( 'NONE',  ( -1.224646799147353207E-16, -1.349345573449484691E-32, 1.000000000000000000 ) ) ;
#19029=AXIS2_PLACEMENT_3D ( 'NONE', #28022, #7840, #5381 ) ;
#19033=FACE_OUTER_BOUND ( 'NONE', #23607, .T. ) ;
#19037=ORIENTED_EDGE ( 'NONE', *, *, #17857, .F. ) ;
#19045=EDGE_CURVE ( 'NONE', #31503, #19462, #10775, .T. ) ;
#19048=DIRECTION ( 'NONE',  ( -1.101824276508909887E-16, 1.000000000000000000, -0.000000000000000000 ) ) ;
#19054=ORIENTED_EDGE ( 'NONE', *, *, #3172, .T. ) ;
#19055=TOROIDAL_SURFACE ( 'NONE', #15936, 12.40141737965280200, 0.1249999999999999445 ) ;
#19059=EDGE_CURVE ( 'NONE', #15022, #27344, #10266, .T. ) ;
#19065=DIRECTION ( 'NONE',  ( -1.101824276508909887E-16, 1.000000000000000000, -0.000000000000000000 ) ) ;
#19067=VERTEX_POINT ( 'NONE', #11068 ) ;
#19068=DIRECTION ( 'NONE',  ( -1.000000000000000000, -1.101824276508909887E-16, 0.000000000000000000 ) ) ;
#19071=CARTESIAN_POINT ( 'NONE',  ( 21.09992658989238734, 31.46183152705961561, 47.04930799450051637 ) ) ;
#19076=CARTESIAN_POINT ( 'NONE',  ( 8.823509210239560474, 29.34164230456639899, 47.04930799450051637 ) ) ;
#19078=DIRECTION ( 'NONE',  ( -1.101824276508909887E-16, 1.000000000000000000, -0.000000000000000000 ) ) ;
#19086=CARTESIAN_POINT ( 'NONE',  ( 33.72499318558949000, 38.56284415653841791, 47.04930799450051637 ) ) ;
#19090=CARTESIAN_POINT ( 'NONE',  ( 21.09992658989239089, 26.59164230456639899, 47.04930799450051637 ) ) ;
#19091=CIRCLE ( 'NONE', #7076, 0.1250000000000001110 ) ;
#19096=CIRCLE ( 'NONE', #16486, 12.27641737965280555 ) ;
#19097=EDGE_CURVE ( 'NONE', #18749, #26804, #23690, .T. ) ;
#19099=CARTESIAN_POINT ( 'NONE',  ( 8.482002859293789498, 30.71664230456641675, 47.04930799450051637 ) ) ;
#19100=ORIENTED_EDGE ( 'NONE', *, *, #23669, .F. ) ;
#19101=AXIS2_PLACEMENT_3D ( 'NONE', #8504, #5559, #13438 ) ;
#19102=EDGE_CURVE ( 'NONE', #28361, #5841, #21267, .T. ) ;
#19103=CYLINDRICAL_SURFACE ( 'NONE', #4689, 12.62506659569710266 ) ;
#19105=ORIENTED_EDGE ( 'NONE', *, *, #5574, .T. ) ;
#19109=ORIENTED_EDGE ( 'NONE', *, *, #5945, .T. ) ;
#19111=CARTESIAN_POINT ( 'NONE',  ( 21.09992658989239089, 29.34164230456639899, 47.04930799450051637 ) ) ;
#19112=DIRECTION ( 'NONE',  ( -1.224646799147353207E-16, -1.349345573449484691E-32, 1.000000000000000000 ) ) ;
#19113=CARTESIAN_POINT ( 'NONE',  ( 21.09992658989239089, 27.34164230456639544, 47.04930799450051637 ) ) ;
#19114=CARTESIAN_POINT ( 'NONE',  ( 21.09992658989238734, 38.56284415653841791, 47.04930799450051637 ) ) ;
#19116=DIRECTION ( 'NONE',  ( -1.000000000000000000, -1.101824276508909887E-16, 0.000000000000000000 ) ) ;
#19118=VERTEX_POINT ( 'NONE', #10590 ) ;
#19119=FACE_OUTER_BOUND ( 'NONE', #12323, .T. ) ;
#19120=CARTESIAN_POINT ( 'NONE',  ( 8.474859994195282908, 38.56284415653841791, 47.04930799450051637 ) ) ;
#19122=AXIS2_PLACEMENT_3D ( 'NONE', #11291, #14241, #19139 ) ;
#19127=AXIS2_PLACEMENT_3D ( 'NONE', #17097, #26183, #18784 ) ;
#19131=ADVANCED_FACE ( 'NONE', ( #11219 ), #28143, .T. ) ;
#19134=EDGE_CURVE ( 'NONE', #22868, #13543, #8697, .T. ) ;
#19136=CIRCLE ( 'NONE', #14978, 12.62506659569710266 ) ;
#19139=DIRECTION ( 'NONE',  ( -1.000000000000000000, -1.101824276508909887E-16, 0.000000000000000000 ) ) ;
#19145=CARTESIAN_POINT ( 'NONE',  ( 33.37634396954519644, 31.59164230456639544, 47.04930799450051637 ) ) ;
#19147=AXIS2_PLACEMENT_3D ( 'NONE', #25668, #3496, #31247 ) ;
#19155=DIRECTION ( 'NONE',  ( 1.000000000000000000, 0.000000000000000000, 0.000000000000000000 ) ) ;
#19158=CARTESIAN_POINT ( 'NONE',  ( 8.474859994195281132, 38.56284415653841791, 47.04930799450051637 ) ) ;
#19160=DIRECTION ( 'NONE',  ( -1.000000000000000000, 0.000000000000000000, 0.000000000000000000 ) ) ;
#19163=AXIS2_PLACEMENT_3D ( 'NONE', #984, #8701, #11010 ) ;
#19165=LINE ( 'NONE', #6222, #27209 ) ;
#19166=ORIENTED_EDGE ( 'NONE', *, *, #7127, .F. ) ;
#19167=DIRECTION ( 'NONE',  ( -1.101824276508909887E-16, 1.000000000000000000, -0.000000000000000000 ) ) ;
#19169=CARTESIAN_POINT ( 'NONE',  ( 33.72499318558949000, 38.56284415653841791, 47.04930799450051637 ) ) ;
#19171=ORIENTED_EDGE ( 'NONE', *, *, #19006, .T. ) ;
#19178=FACE_OUTER_BOUND ( 'NONE', #435, .T. ) ;
#19185=ADVANCED_FACE ( 'NONE', ( #12026 ), #16608, .T. ) ;
#19188=ORIENTED_EDGE ( 'NONE', *, *, #11685, .F. ) ;
#19195=CARTESIAN_POINT ( 'NONE',  ( 21.09992658989238734, 38.56284415653841791, 47.04930799450051637 ) ) ;
#19196=CIRCLE ( 'NONE', #31784, 0.1250000000000001110 ) ;
#19205=EDGE_CURVE ( 'NONE', #1940, #13978, #25975, .T. ) ;
#19207=DIRECTION ( 'NONE',  ( 1.000000000000000000, 0.000000000000000000, 0.000000000000000000 ) ) ;
#19210=ORIENTED_EDGE ( 'NONE', *, *, #7218, .T. ) ;
#19211=CARTESIAN_POINT ( 'NONE',  ( 8.698509210239565803, 29.84164230456639899, 47.04930799450051637 ) ) ;
#19216=ORIENTED_EDGE ( 'NONE', *, *, #20678, .F. ) ;
#19219=EDGE_CURVE ( 'NONE', #11938, #5749, #9240, .T. ) ;
#19225=CARTESIAN_POINT ( 'NONE',  ( 21.09992658989238734, 31.34164230456639544, 47.04930799450051637 ) ) ;
#19228=CARTESIAN_POINT ( 'NONE',  ( 8.732853799281734553, 38.56284415653841791, 47.04930799450051637 ) ) ;
#19232=LINE ( 'NONE', #16780, #9484 ) ;
#19240=ORIENTED_EDGE ( 'NONE', *, *, #27994, .F. ) ;
#19245=ADVANCED_FACE ( 'NONE', ( #6773 ), #30707, .T. ) ;
#19246=DIRECTION ( 'NONE',  ( -1.101824276508909887E-16, 1.000000000000000000, -0.000000000000000000 ) ) ;
#19250=EDGE_CURVE ( 'NONE', #18749, #15685, #27035, .T. ) ;
#19252=TOROIDAL_SURFACE ( 'NONE', #13512, 12.40141737965280022, 0.1249999999999992228 ) ;
#19253=ORIENTED_EDGE ( 'NONE', *, *, #16334, .F. ) ;
#19254=ADVANCED_FACE ( 'NONE', ( #14006 ), #4144, .T. ) ;
#19259=CIRCLE ( 'NONE', #5143, 0.1249999999999983763 ) ;
#19263=EDGE_LOOP ( 'NONE', ( #15405, #14592, #12166, #22625 ) ) ;
#19265=CIRCLE ( 'NONE', #24526, 12.27641737965282154 ) ;
#19270=FACE_OUTER_BOUND ( 'NONE', #31991, .T. ) ;
#19273=CARTESIAN_POINT ( 'NONE',  ( 33.37634396954518934, 31.84164230456639544, 47.04930799450051637 ) ) ;
#19275=FACE_OUTER_BOUND ( 'NONE', #31822, .T. ) ;
#19277=ORIENTED_EDGE ( 'NONE', *, *, #19976, .T. ) ;
#19280=EDGE_CURVE ( 'NONE', #16708, #1140, #14824, .T. ) ;
#19282=FACE_OUTER_BOUND ( 'NONE', #9422, .T. ) ;
#19286=ORIENTED_EDGE ( 'NONE', *, *, #2797, .F. ) ;
#19287=ORIENTED_EDGE ( 'NONE', *, *, #29853, .F. ) ;
#19288=CIRCLE ( 'NONE', #5156, 0.1250000000000001110 ) ;
#19291=EDGE_CURVE ( 'NONE', #12553, #24565, #305, .T. ) ;
#19292=AXIS2_PLACEMENT_3D ( 'NONE', #28559, #3598, #6389 ) ;
#19294=AXIS2_PLACEMENT_3D ( 'NONE', #16131, #3665, #28775 ) ;
#19295=CIRCLE ( 'NONE', #5167, 12.36707279061065101 ) ;
#19299=VERTEX_POINT ( 'NONE', #24990 ) ;
#19301=CARTESIAN_POINT ( 'NONE',  ( 21.09992658989239089, 25.59164230456639899, 47.04930799450051637 ) ) ;
#19306=CARTESIAN_POINT ( 'NONE',  ( 33.50134396954519644, 31.59164230456639544, 47.04930799450051637 ) ) ;
#19314=DIRECTION ( 'NONE',  ( -1.000000000000000000, 0.000000000000000000, 0.000000000000000000 ) ) ;
#19323=CARTESIAN_POINT ( 'NONE',  ( 21.09992658989238734, 32.47145308207317527, 47.04930799450051637 ) ) ;
#19330=CARTESIAN_POINT ( 'NONE',  ( 33.72499318558949710, 25.84184655352419213, 47.04930799450051637 ) ) ;
#19331=EDGE_LOOP ( 'NONE', ( #17186, #5617, #16667, #18705 ) ) ;
#19333=DIRECTION ( 'NONE',  ( -1.000000000000000000, 0.000000000000000000, 0.000000000000000000 ) ) ;
#19337=EDGE_CURVE ( 'NONE', #23072, #7677, #7597, .T. ) ;
#19338=AXIS2_PLACEMENT_3D ( 'NONE', #26996, #14038, #29136 ) ;
#19342=DIRECTION ( 'NONE',  ( 1.000000000000000000, 0.000000000000000000, 0.000000000000000000 ) ) ;
#19345=VERTEX_POINT ( 'NONE', #24830 ) ;
#19346=DIRECTION ( 'NONE',  ( -1.101824276508909887E-16, 1.000000000000000000, -0.000000000000000000 ) ) ;
#19347=CIRCLE ( 'NONE', #5756, 12.36707279061065101 ) ;
#19351=ORIENTED_EDGE ( 'NONE', *, *, #11012, .F. ) ;
#19352=DIRECTION ( 'NONE',  ( -1.000000000000000000, 0.000000000000000000, 0.000000000000000000 ) ) ;
#19359=ORIENTED_EDGE ( 'NONE', *, *, #11566, .F. ) ;
#19363=AXIS2_PLACEMENT_3D ( 'NONE', #4158, #18600, #31418 ) ;
#19376=EDGE_CURVE ( 'NONE', #21925, #10074, #21233, .T. ) ;
#19377=AXIS2_PLACEMENT_3D ( 'NONE', #12557, #22547, #25185 ) ;
#19378=EDGE_CURVE ( 'NONE', #5687, #19469, #7102, .T. ) ;
#19379=AXIS2_PLACEMENT_3D ( 'NONE', #23050, #3184, #7804 ) ;
#19380=ORIENTED_EDGE ( 'NONE', *, *, #15375, .T. ) ;
#19381=CARTESIAN_POINT ( 'NONE',  ( 21.09992658989239089, 27.09164230456639899, 47.04930799450051637 ) ) ;
#19390=CIRCLE ( 'NONE', #7893, 0.1250000000000001110 ) ;
#19397=TOROIDAL_SURFACE ( 'NONE', #5270, 12.40141737965286595, 0.1249999999999979183 ) ;
#19400=CIRCLE ( 'NONE', #17847, 0.1250000000000001110 ) ;
#19402=EDGE_CURVE ( 'NONE', #3968, #3369, #18104, .T. ) ;
#19409=DIRECTION ( 'NONE',  ( -1.000000000000000000, 0.000000000000000000, 0.000000000000000000 ) ) ;
#19420=ADVANCED_FACE ( 'NONE', ( #4970 ), #15305, .F. ) ;
#19424=TOROIDAL_SURFACE ( 'NONE', #2665, 12.40141737965285529, 0.1250000000000000555 ) ;
#19431=DIRECTION ( 'NONE',  ( -1.101824276508909887E-16, 1.000000000000000000, -0.000000000000000000 ) ) ;
#19432=TOROIDAL_SURFACE ( 'NONE', #11573, 12.40141737965283042, 0.1249999999999995420 ) ;
#19434=ORIENTED_EDGE ( 'NONE', *, *, #11394, .T. ) ;
#19435=DIRECTION ( 'NONE',  ( 1.000000000000000000, 0.000000000000000000, 0.000000000000000000 ) ) ;
#19436=ORIENTED_EDGE ( 'NONE', *, *, #17029, .T. ) ;
#19437=CYLINDRICAL_SURFACE ( 'NONE', #19338, 12.36707279061065279 ) ;
#19438=DIRECTION ( 'NONE',  ( -1.101824276508909887E-16, 1.000000000000000000, -0.000000000000000000 ) ) ;
#19441=EDGE_CURVE ( 'NONE', #27386, #21015, #28738, .T. ) ;
#19447=FACE_OUTER_BOUND ( 'NONE', #12627, .T. ) ;
#19451=CIRCLE ( 'NONE', #23107, 12.27641737965287128 ) ;
#19453=DIRECTION ( 'NONE',  ( -1.224646799147353207E-16, -1.349345573449484691E-32, 1.000000000000000000 ) ) ;
#19456=CARTESIAN_POINT ( 'NONE',  ( 8.732853799281738105, 24.71183152705960140, 47.04930799450051637 ) ) ;
#19458=DIRECTION ( 'NONE',  ( -1.000000000000000000, 0.000000000000000000, 0.000000000000000000 ) ) ;
#19462=VERTEX_POINT ( 'NONE', #16095 ) ;
#19468=EDGE_CURVE ( 'NONE', #16672, #25906, #25475, .T. ) ;
#19469=VERTEX_POINT ( 'NONE', #3306 ) ;
#19470=ORIENTED_EDGE ( 'NONE', *, *, #29732, .T. ) ;
#19473=DIRECTION ( 'NONE',  ( -1.101824276508909887E-16, 1.000000000000000000, -0.000000000000000000 ) ) ;
#19477=DIRECTION ( 'NONE',  ( -1.101824276508909887E-16, 1.000000000000000000, -0.000000000000000000 ) ) ;
#19478=ORIENTED_EDGE ( 'NONE', *, *, #18551, .F. ) ;
#19494=DIRECTION ( 'NONE',  ( -1.000000000000000000, -1.101824276508909764E-16, 0.000000000000000000 ) ) ;
#19497=FACE_OUTER_BOUND ( 'NONE', #2767, .T. ) ;
#19502=ORIENTED_EDGE ( 'NONE', *, *, #18829, .T. ) ;
#19503=AXIS2_PLACEMENT_3D ( 'NONE', #29217, #9361, #7060 ) ;
#19506=DIRECTION ( 'NONE',  ( 0.000000000000000000, -0.000000000000000000, -1.000000000000000000 ) ) ;
#19515=EDGE_LOOP ( 'NONE', ( #30730, #7150, #6655, #19286 ) ) ;
#19516=EDGE_LOOP ( 'NONE', ( #4728, #2048, #31292, #19470 ) ) ;
#19519=ORIENTED_EDGE ( 'NONE', *, *, #21032, .F. ) ;
#19521=CARTESIAN_POINT ( 'NONE',  ( 21.09992658989239089, 26.34164230456639899, 47.04930799450051637 ) ) ;
#19522=DIRECTION ( 'NONE',  ( 0.000000000000000000, -0.000000000000000000, -1.000000000000000000 ) ) ;
#19526=ORIENTED_EDGE ( 'NONE', *, *, #1320, .T. ) ;
#19530=LINE ( 'NONE', #30051, #30899 ) ;
#19531=AXIS2_PLACEMENT_3D ( 'NONE', #16862, #31969, #16372 ) ;
#19532=ORIENTED_EDGE ( 'NONE', *, *, #10805, .F. ) ;
#19534=DIRECTION ( 'NONE',  ( -1.000000000000000000, 0.000000000000000000, 0.000000000000000000 ) ) ;
#19536=ORIENTED_EDGE ( 'NONE', *, *, #27906, .F. ) ;
#19538=CARTESIAN_POINT ( 'NONE',  ( 8.732853799281734553, 38.56284415653841791, 47.04930799450051637 ) ) ;
#19539=CARTESIAN_POINT ( 'NONE',  ( 21.09992658989238734, 31.09184655352422411, 47.04930799450051637 ) ) ;
#19542=DIRECTION ( 'NONE',  ( -1.000000000000000000, 0.000000000000000000, 0.000000000000000000 ) ) ;
#19548=DIRECTION ( 'NONE',  ( -1.000000000000000000, 0.000000000000000000, 0.000000000000000000 ) ) ;
#19550=CARTESIAN_POINT ( 'NONE',  ( 21.09992658989239089, 26.71183152705960495, 47.04930799450051637 ) ) ;
#19552=EDGE_CURVE ( 'NONE', #12341, #19026, #22867, .T. ) ;
#19553=CARTESIAN_POINT ( 'NONE',  ( 33.50134396954521776, 29.59164230456639899, 47.04930799450051637 ) ) ;
#19555=DIRECTION ( 'NONE',  ( -1.000000000000000000, 0.000000000000000000, 0.000000000000000000 ) ) ;
#19556=EDGE_CURVE ( 'NONE', #15217, #9970, #330, .T. ) ;
#19560=TOROIDAL_SURFACE ( 'NONE', #28483, 12.40141737965283930, 0.1250000000000007216 ) ;
#19577=ORIENTED_EDGE ( 'NONE', *, *, #25650, .T. ) ;
#19582=CIRCLE ( 'NONE', #30612, 0.1250000000000001110 ) ;
#19584=ORIENTED_EDGE ( 'NONE', *, *, #30868, .T. ) ;
#19585=EDGE_CURVE ( 'NONE', #7034, #28434, #18134, .T. ) ;
#19586=ORIENTED_EDGE ( 'NONE', *, *, #12465, .F. ) ;
#19589=DIRECTION ( 'NONE',  ( -1.101824276508909887E-16, 1.000000000000000000, -0.000000000000000000 ) ) ;
#19591=ORIENTED_EDGE ( 'NONE', *, *, #12952, .F. ) ;
#19594=EDGE_LOOP ( 'NONE', ( #1410, #21906, #11513, #22460 ) ) ;
#19595=DIRECTION ( 'NONE',  ( -1.224646799147353207E-16, -1.349345573449484691E-32, 1.000000000000000000 ) ) ;
#19596=VERTEX_POINT ( 'NONE', #13810 ) ;
#19599=EDGE_CURVE ( 'NONE', #16423, #27923, #4525, .T. ) ;
#19601=ORIENTED_EDGE ( 'NONE', *, *, #25247, .T. ) ;
#19608=DIRECTION ( 'NONE',  ( -1.101824276508909887E-16, 1.000000000000000000, -0.000000000000000000 ) ) ;
#19609=DIRECTION ( 'NONE',  ( -1.000000000000000000, 0.000000000000000000, 0.000000000000000000 ) ) ;
#19611=CARTESIAN_POINT ( 'NONE',  ( 21.09992658989239089, 25.34143805560860940, 47.04930799450051637 ) ) ;
#19612=CARTESIAN_POINT ( 'NONE',  ( 33.37634396954527460, 24.34164230456639544, 47.04930799450051637 ) ) ;
#19614=ADVANCED_FACE ( 'NONE', ( #19033 ), #21826, .T. ) ;
#19615=EDGE_LOOP ( 'NONE', ( #10769, #22309, #28715, #21656 ) ) ;
#19618=AXIS2_PLACEMENT_3D ( 'NONE', #1997, #27761, #15130 ) ;
#19619=CIRCLE ( 'NONE', #29603, 12.62506659569710443 ) ;
#19621=CIRCLE ( 'NONE', #30667, 12.36707279061065101 ) ;
#19629=CARTESIAN_POINT ( 'NONE',  ( 21.09992658989239089, 26.46664230456639899, 47.04930799450051637 ) ) ;
#19633=EDGE_LOOP ( 'NONE', ( #11578, #16703, #32092, #28417 ) ) ;
#19639=CARTESIAN_POINT ( 'NONE',  ( 8.732853799281729223, 27.72145308207318237, 47.04930799450051637 ) ) ;
#19642=CARTESIAN_POINT ( 'NONE',  ( 21.09992658989239089, 25.72145308207319303, 47.04930799450051637 ) ) ;
#19645=AXIS2_PLACEMENT_3D ( 'NONE', #190, #5113, #10208 ) ;
#19649=ORIENTED_EDGE ( 'NONE', *, *, #25255, .F. ) ;
#19653=CYLINDRICAL_SURFACE ( 'NONE', #32393, 12.36707279061065101 ) ;
#19658=EDGE_CURVE ( 'NONE', #18133, #3119, #11856, .T. ) ;
#19659=EDGE_LOOP ( 'NONE', ( #29400, #15257, #11935, #30348 ) ) ;
#19660=DIRECTION ( 'NONE',  ( -1.000000000000000000, 0.000000000000000000, 0.000000000000000000 ) ) ;
#19661=EDGE_CURVE ( 'NONE', #10922, #15685, #11322, .T. ) ;
#19662=ORIENTED_EDGE ( 'NONE', *, *, #16843, .F. ) ;
#19668=CARTESIAN_POINT ( 'NONE',  ( 8.732853799281731000, 27.22145308207318237, 47.04930799450051637 ) ) ;
#19671=AXIS2_PLACEMENT_3D ( 'NONE', #9923, #7630, #17467 ) ;
#19672=VERTEX_POINT ( 'NONE', #27577 ) ;
#19673=DIRECTION ( 'NONE',  ( -1.101824276508909887E-16, 1.000000000000000000, -0.000000000000000000 ) ) ;
#19674=CARTESIAN_POINT ( 'NONE',  ( 21.09992658989239089, 26.71664230456639899, 47.04930799450051637 ) ) ;
#19678=VERTEX_POINT ( 'NONE', #17066 ) ;
#19680=ORIENTED_EDGE ( 'NONE', *, *, #22751, .F. ) ;
#19688=ORIENTED_EDGE ( 'NONE', *, *, #27391, .F. ) ;
#19690=DIRECTION ( 'NONE',  ( -1.101824276508909887E-16, 1.000000000000000000, -0.000000000000000000 ) ) ;
#19695=CARTESIAN_POINT ( 'NONE',  ( 33.50134396954523197, 28.09164230456639544, 47.04930799450051637 ) ) ;
#19696=EDGE_CURVE ( 'NONE', #15433, #7860, #1348, .T. ) ;
#19697=ORIENTED_EDGE ( 'NONE', *, *, #5166, .T. ) ;
#19702=EDGE_CURVE ( 'NONE', #19678, #20658, #23900, .T. ) ;
#19703=LINE ( 'NONE', #10194, #7055 ) ;
#19704=EDGE_CURVE ( 'NONE', #2267, #31427, #9756, .T. ) ;
#19706=EDGE_LOOP ( 'NONE', ( #13351, #4809, #11576, #12375 ) ) ;
#19710=DIRECTION ( 'NONE',  ( -1.101824276508909887E-16, 1.000000000000000000, -0.000000000000000000 ) ) ;
#19711=FACE_OUTER_BOUND ( 'NONE', #12221, .T. ) ;
#19714=DIRECTION ( 'NONE',  ( -1.000000000000000000, 0.000000000000000000, 0.000000000000000000 ) ) ;
#19718=CARTESIAN_POINT ( 'NONE',  ( 33.46699938050304013, 23.97145308207319658, 47.04930799450050927 ) ) ;
#19721=CYLINDRICAL_SURFACE ( 'NONE', #12626, 12.36707279061065101 ) ;
#19736=ORIENTED_EDGE ( 'NONE', *, *, #10945, .F. ) ;
#19739=DIRECTION ( 'NONE',  ( -1.000000000000000000, 0.000000000000000000, 0.000000000000000000 ) ) ;
#19746=ADVANCED_FACE ( 'NONE', ( #5092 ), #32296, .T. ) ;
#19757=ORIENTED_EDGE ( 'NONE', *, *, #20678, .T. ) ;
#19758=CARTESIAN_POINT ( 'NONE',  ( 21.09992658989239089, 28.09143805560861296, 47.04930799450051637 ) ) ;
#19760=CARTESIAN_POINT ( 'NONE',  ( 21.09992658989239089, 24.34164230456639544, 47.04930799450051637 ) ) ;
#19764=TOROIDAL_SURFACE ( 'NONE', #4044, 12.40141737965284641, 0.1249999999999995698 ) ;
#19769=ORIENTED_EDGE ( 'NONE', *, *, #30948, .T. ) ;
#19770=DIRECTION ( 'NONE',  ( -1.000000000000000000, -1.101824276508909887E-16, 0.000000000000000000 ) ) ;
#19773=ORIENTED_EDGE ( 'NONE', *, *, #29808, .F. ) ;
#19774=DIRECTION ( 'NONE',  ( 1.000000000000000000, 0.000000000000000000, 0.000000000000000000 ) ) ;
#19781=VERTEX_POINT ( 'NONE', #29884 ) ;
#19785=EDGE_CURVE ( 'NONE', #15685, #2384, #23911, .T. ) ;
#19787=TOROIDAL_SURFACE ( 'NONE', #20376, 12.40141737965281266, 0.1249999999999994865 ) ;
#19788=VECTOR ( 'NONE', #14749, 1000.000000000000000 ) ;
#19790=TOROIDAL_SURFACE ( 'NONE', #5662, 12.40141737965287305, 0.1250000000000000833 ) ;
#19791=ORIENTED_EDGE ( 'NONE', *, *, #21443, .F. ) ;
#19792=CARTESIAN_POINT ( 'NONE',  ( 21.09992658989239089, 28.84164230456639544, 47.04930799450051637 ) ) ;
#19793=FACE_OUTER_BOUND ( 'NONE', #11020, .T. ) ;
#19797=ORIENTED_EDGE ( 'NONE', *, *, #8062, .T. ) ;
#19816=ORIENTED_EDGE ( 'NONE', *, *, #27391, .T. ) ;
#19820=CARTESIAN_POINT ( 'NONE',  ( 21.09992658989239089, 30.34164230456639544, 47.04930799450051637 ) ) ;
#19821=TOROIDAL_SURFACE ( 'NONE', #5674, 12.40141737965286239, 0.1250000000000005551 ) ;
#19822=VERTEX_POINT ( 'NONE', #20985 ) ;
#19826=AXIS2_PLACEMENT_3D ( 'NONE', #11364, #21688, #21351 ) ;
#19831=DIRECTION ( 'NONE',  ( -1.000000000000000000, 0.000000000000000000, 0.000000000000000000 ) ) ;
#19832=AXIS2_PLACEMENT_3D ( 'NONE', #26337, #3855, #1384 ) ;
#19838=EDGE_CURVE ( 'NONE', #10702, #17879, #23454, .T. ) ;
#19840=ORIENTED_EDGE ( 'NONE', *, *, #19006, .F. ) ;
#19842=CARTESIAN_POINT ( 'NONE',  ( 33.50134396954520355, 30.84164230456639544, 47.04930799450051637 ) ) ;
#19843=EDGE_LOOP ( 'NONE', ( #22085, #14111, #32434, #22202 ) ) ;
#19848=DIRECTION ( 'NONE',  ( -1.000000000000000000, 0.000000000000000000, 0.000000000000000000 ) ) ;
#19849=CARTESIAN_POINT ( 'NONE',  ( 21.09992658989239089, 27.84143805560860940, 47.04930799450051637 ) ) ;
#19854=EDGE_CURVE ( 'NONE', #13978, #15187, #863, .T. ) ;
#19855=CARTESIAN_POINT ( 'NONE',  ( 33.62240545574881878, 32.54735957529758394, 47.04930799450051637 ) ) ;
#19856=ADVANCED_FACE ( 'NONE', ( #8050 ), #10844, .T. ) ;
#19865=AXIS2_PLACEMENT_3D ( 'NONE', #7618, #24347, #29610 ) ;
#19868=ORIENTED_EDGE ( 'NONE', *, *, #31177, .F. ) ;
#19870=ORIENTED_EDGE ( 'NONE', *, *, #8560, .F. ) ;
#19877=EDGE_CURVE ( 'NONE', #15854, #29858, #6108, .T. ) ;
#19879=CIRCLE ( 'NONE', #3627, 12.36707279061065101 ) ;
#19881=EDGE_CURVE ( 'NONE', #26330, #2027, #29163, .T. ) ;
#19882=CARTESIAN_POINT ( 'NONE',  ( 21.09992658989239089, 29.09184655352418858, 47.04930799450051637 ) ) ;
#19884=DIRECTION ( 'NONE',  ( -1.101824276508909887E-16, 1.000000000000000000, -0.000000000000000000 ) ) ;
#19891=CARTESIAN_POINT ( 'NONE',  ( 21.09992658989238734, 31.46664230456641675, 47.04930799450051637 ) ) ;
#19894=AXIS2_PLACEMENT_3D ( 'NONE', #9411, #23853, #11873 ) ;
#19897=ORIENTED_EDGE ( 'NONE', *, *, #1746, .T. ) ;
#19898=FACE_OUTER_BOUND ( 'NONE', #2995, .T. ) ;
#19900=DIRECTION ( 'NONE',  ( -1.000000000000000000, 0.000000000000000000, 0.000000000000000000 ) ) ;
#19901=CARTESIAN_POINT ( 'NONE',  ( 8.474859994195281132, 32.09184655352418503, 47.04930799450051637 ) ) ;
#19906=AXIS2_PLACEMENT_3D ( 'NONE', #21221, #4156, #16141 ) ;
#19907=DIRECTION ( 'NONE',  ( 0.000000000000000000, -0.000000000000000000, -1.000000000000000000 ) ) ;
#19908=CARTESIAN_POINT ( 'NONE',  ( 8.698509210239574685, 31.09164230456639544, 47.04930799450051637 ) ) ;
#19911=TOROIDAL_SURFACE ( 'NONE', #28313, 12.40141737965282687, 0.1250000000000004718 ) ;
#19912=AXIS2_PLACEMENT_3D ( 'NONE', #8585, #23994, #23516 ) ;
#19914=DIRECTION ( 'NONE',  ( -1.000000000000000000, 0.000000000000000000, 0.000000000000000000 ) ) ;
#19915=AXIS2_PLACEMENT_3D ( 'NONE', #13604, #31805, #26394 ) ;
#19916=TOROIDAL_SURFACE ( 'NONE', #14160, 12.61792373059896732, 0.1249999999999974604 ) ;
#19918=AXIS2_PLACEMENT_3D ( 'NONE', #25506, #20247, #3005 ) ;
#19920=DIRECTION ( 'NONE',  ( -1.000000000000000000, -1.101824276508909887E-16, 0.000000000000000000 ) ) ;
#19922=EDGE_LOOP ( 'NONE', ( #28372, #3274, #3875, #2366 ) ) ;
#19925=DIRECTION ( 'NONE',  ( -1.000000000000000000, -1.101824276508909764E-16, 0.000000000000000000 ) ) ;
#19928=DIRECTION ( 'NONE',  ( -1.101824276508909887E-16, 1.000000000000000000, -0.000000000000000000 ) ) ;
#19929=EDGE_LOOP ( 'NONE', ( #2666, #11230, #17974, #16428 ) ) ;
#19939=CARTESIAN_POINT ( 'NONE',  ( 33.46699938050304013, 31.71183152705962272, 47.04930799450051637 ) ) ;
#19943=AXIS2_PLACEMENT_3D ( 'NONE', #11267, #31288, #8788 ) ;
#19944=CARTESIAN_POINT ( 'NONE',  ( 33.72499318558949000, 38.56284415653841791, 47.04930799450051637 ) ) ;
#19947=AXIS2_PLACEMENT_3D ( 'NONE', #18073, #22997, #24985 ) ;
#19952=ORIENTED_EDGE ( 'NONE', *, *, #28144, .F. ) ;
#19958=DIRECTION ( 'NONE',  ( -1.101824276508909887E-16, 1.000000000000000000, -0.000000000000000000 ) ) ;
#19960=DIRECTION ( 'NONE',  ( -1.101824276508909887E-16, 1.000000000000000000, -0.000000000000000000 ) ) ;
#19963=AXIS2_PLACEMENT_3D ( 'NONE', #27359, #4878, #7508 ) ;
#19970=ORIENTED_EDGE ( 'NONE', *, *, #30, .T. ) ;
#19976=EDGE_CURVE ( 'NONE', #30857, #30310, #19196, .T. ) ;
#19977=EDGE_CURVE ( 'NONE', #17800, #10801, #11883, .T. ) ;
#19979=EDGE_CURVE ( 'NONE', #10074, #4416, #15034, .T. ) ;
#19981=DIRECTION ( 'NONE',  ( -1.000000000000000000, 0.000000000000000000, 0.000000000000000000 ) ) ;
#19982=EDGE_CURVE ( 'NONE', #2064, #13866, #26537, .T. ) ;
#19983=EDGE_CURVE ( 'NONE', #20832, #24454, #28653, .T. ) ;
#19987=EDGE_LOOP ( 'NONE', ( #2446, #7527, #850, #24305 ) ) ;
#19988=AXIS2_PLACEMENT_3D ( 'NONE', #19090, #9101, #9427 ) ;
#19992=AXIS2_PLACEMENT_3D ( 'NONE', #12238, #15180, #15654 ) ;
#19994=AXIS2_PLACEMENT_3D ( 'NONE', #15346, #7483, #12245 ) ;
#20001=ORIENTED_EDGE ( 'NONE', *, *, #18520, .F. ) ;
#20003=FACE_OUTER_BOUND ( 'NONE', #473, .T. ) ;
#20006=ORIENTED_EDGE ( 'NONE', *, *, #2797, .T. ) ;
#20008=DIRECTION ( 'NONE',  ( -1.000000000000000000, -1.101824276508909887E-16, 0.000000000000000000 ) ) ;
#20010=CARTESIAN_POINT ( 'NONE',  ( 21.09992658989239089, 24.59143805560860940, 47.04930799450051637 ) ) ;
#20012=DIRECTION ( 'NONE',  ( -1.101824276508909887E-16, 1.000000000000000000, -0.000000000000000000 ) ) ;
#20014=AXIS2_PLACEMENT_3D ( 'NONE', #16520, #4220, #6519 ) ;
#20015=TOROIDAL_SURFACE ( 'NONE', #25777, 12.40141737965287838, 0.1249999999999998335 ) ;
#20018=ADVANCED_FACE ( 'NONE', ( #24418 ), #26023, .T. ) ;
#20026=CARTESIAN_POINT ( 'NONE',  ( 8.698509210239516065, 25.09164230456639899, 47.04930799450051637 ) ) ;
#20030=EDGE_CURVE ( 'NONE', #13402, #19462, #21135, .T. ) ;
#20031=CIRCLE ( 'NONE', #5390, 12.36707279061065101 ) ;
#20036=CIRCLE ( 'NONE', #22663, 0.1249999999999983763 ) ;
#20039=LINE ( 'NONE', #2163, #5590 ) ;
#20040=CARTESIAN_POINT ( 'NONE',  ( 21.09992658989239089, 27.59164230456639544, 47.04930799450051637 ) ) ;
#20051=DIRECTION ( 'NONE',  ( 0.000000000000000000, -0.000000000000000000, -1.000000000000000000 ) ) ;
#20052=AXIS2_PLACEMENT_3D ( 'NONE', #16091, #1000, #1154 ) ;
#20054=FACE_OUTER_BOUND ( 'NONE', #16403, .T. ) ;
#20055=TOROIDAL_SURFACE ( 'NONE', #32126, 12.40141737965288371, 0.1249999999999996253 ) ;
#20057=ADVANCED_FACE ( 'NONE', ( #26559 ), #18831, .F. ) ;
#20061=CARTESIAN_POINT ( 'NONE',  ( 33.37634396954519644, 31.34164230456639544, 47.04930799450051637 ) ) ;
#20064=CARTESIAN_POINT ( 'NONE',  ( 8.823509210239571132, 30.34164230456639544, 47.04930799450051637 ) ) ;
#20066=CIRCLE ( 'NONE', #15884, 0.1250000000000001110 ) ;
#20071=ORIENTED_EDGE ( 'NONE', *, *, #27161, .F. ) ;
#20075=DIRECTION ( 'NONE',  ( -1.224646799147353207E-16, -1.349345573449484691E-32, 1.000000000000000000 ) ) ;
#20077=EDGE_CURVE ( 'NONE', #13126, #14963, #16867, .T. ) ;
#20079=AXIS2_PLACEMENT_3D ( 'NONE', #10831, #15572, #22953 ) ;
#20081=DIRECTION ( 'NONE',  ( -1.101824276508909887E-16, 1.000000000000000000, -0.000000000000000000 ) ) ;
#20086=DIRECTION ( 'NONE',  ( -1.000000000000000000, 0.000000000000000000, 0.000000000000000000 ) ) ;
#20096=DIRECTION ( 'NONE',  ( -1.101824276508909887E-16, 1.000000000000000000, -0.000000000000000000 ) ) ;
#20097=CARTESIAN_POINT ( 'NONE',  ( 21.09992658989238734, 30.84164230456639544, 47.04930799450051637 ) ) ;
#20098=DIRECTION ( 'NONE',  ( -1.101824276508909887E-16, 1.000000000000000000, -0.000000000000000000 ) ) ;
#20103=DIRECTION ( 'NONE',  ( -1.101824276508909887E-16, 1.000000000000000000, -0.000000000000000000 ) ) ;
#20107=DIRECTION ( 'NONE',  ( -1.000000000000000000, 0.000000000000000000, 0.000000000000000000 ) ) ;
#20108=CARTESIAN_POINT ( 'NONE',  ( 8.732853799281732776, 32.22145308207317527, 47.04930799450051637 ) ) ;
#20112=DIRECTION ( 'NONE',  ( -1.000000000000000000, 0.000000000000000000, 0.000000000000000000 ) ) ;
#20120=ORIENTED_EDGE ( 'NONE', *, *, #17078, .F. ) ;
#20123=AXIS2_PLACEMENT_3D ( 'NONE', #9286, #19453, #14379 ) ;
#20126=DIRECTION ( 'NONE',  ( -1.101824276508909887E-16, 1.000000000000000000, -0.000000000000000000 ) ) ;
#20127=CARTESIAN_POINT ( 'NONE',  ( 21.09992658989239089, 26.84164230456639899, 47.04930799450051637 ) ) ;
#20131=CARTESIAN_POINT ( 'NONE',  ( 21.09992658989239089, 28.84143805560861296, 47.04930799450051637 ) ) ;
#20133=EDGE_LOOP ( 'NONE', ( #6645, #13682, #1995, #31439 ) ) ;
#20134=CARTESIAN_POINT ( 'NONE',  ( 21.09992658989239089, 28.21183152705961206, 47.04930799450051637 ) ) ;
#20135=DIRECTION ( 'NONE',  ( -1.000000000000000000, -1.101824276508910010E-16, 0.000000000000000000 ) ) ;
#20138=CARTESIAN_POINT ( 'NONE',  ( 33.37634396954525329, 25.84164230456639899, 47.04930799450051637 ) ) ;
#20141=CARTESIAN_POINT ( 'NONE',  ( 8.482002859293400476, 24.46664230456639899, 47.04930799450051637 ) ) ;
#20142=EDGE_LOOP ( 'NONE', ( #3537, #26045, #18907, #8798 ) ) ;
#20143=DIRECTION ( 'NONE',  ( -1.000000000000000000, 0.000000000000000000, 0.000000000000000000 ) ) ;
#20144=VERTEX_POINT ( 'NONE', #24092 ) ;
#20145=DIRECTION ( 'NONE',  ( -1.000000000000000000, 0.000000000000000000, 0.000000000000000000 ) ) ;
#20146=ORIENTED_EDGE ( 'NONE', *, *, #1338, .T. ) ;
#20153=ORIENTED_EDGE ( 'NONE', *, *, #17249, .F. ) ;
#20154=EDGE_CURVE ( 'NONE', #29646, #22098, #7696, .T. ) ;
#20155=EDGE_CURVE ( 'NONE', #30180, #27550, #21827, .T. ) ;
#20156=ADVANCED_FACE ( 'NONE', ( #2433 ), #28126, .T. ) ;
#20157=EDGE_CURVE ( 'NONE', #14214, #24454, #21844, .T. ) ;
#20160=FACE_OUTER_BOUND ( 'NONE', #4457, .T. ) ;
#20162=EDGE_LOOP ( 'NONE', ( #2367, #19591, #86, #18790 ) ) ;
#20164=DIRECTION ( 'NONE',  ( -1.000000000000000000, 0.000000000000000000, 0.000000000000000000 ) ) ;
#20167=AXIS2_PLACEMENT_3D ( 'NONE', #19882, #15134, #25142 ) ;
#20172=CIRCLE ( 'NONE', #16995, 0.1250000000000001110 ) ;
#20174=DIRECTION ( 'NONE',  ( -1.101824276508909887E-16, 1.000000000000000000, -0.000000000000000000 ) ) ;
#20179=FACE_OUTER_BOUND ( 'NONE', #17539, .T. ) ;
#20181=EDGE_LOOP ( 'NONE', ( #30278, #5920, #31735, #17417 ) ) ;
#20185=DIRECTION ( 'NONE',  ( -1.000000000000000000, -1.101824276508909887E-16, 0.000000000000000000 ) ) ;
#20196=CIRCLE ( 'NONE', #24389, 0.1250000000000001110 ) ;
#20197=CIRCLE ( 'NONE', #20722, 12.52641737965279489 ) ;
#20203=DIRECTION ( 'NONE',  ( -1.101824276508909887E-16, 1.000000000000000000, -0.000000000000000000 ) ) ;
#20210=CARTESIAN_POINT ( 'NONE',  ( 21.09992658989239089, 25.09143805560860940, 47.04930799450051637 ) ) ;
#20212=CARTESIAN_POINT ( 'NONE',  ( 21.09992658989238734, 38.56284415653841791, 47.04930799450051637 ) ) ;
#20216=ORIENTED_EDGE ( 'NONE', *, *, #3249, .T. ) ;
#20226=CARTESIAN_POINT ( 'NONE',  ( 21.09992658989238734, 32.09143805560860585, 47.04930799450051637 ) ) ;
#20241=AXIS2_PLACEMENT_3D ( 'NONE', #18871, #9204, #12324 ) ;
#20245=DIRECTION ( 'NONE',  ( 0.000000000000000000, -0.000000000000000000, -1.000000000000000000 ) ) ;
#20247=DIRECTION ( 'NONE',  ( 0.000000000000000000, -0.000000000000000000, -1.000000000000000000 ) ) ;
#20248=FACE_OUTER_BOUND ( 'NONE', #25559, .T. ) ;
#20250=DIRECTION ( 'NONE',  ( -1.000000000000000000, 0.000000000000000000, 0.000000000000000000 ) ) ;
#20252=ORIENTED_EDGE ( 'NONE', *, *, #31090, .T. ) ;
#20253=DIRECTION ( 'NONE',  ( -1.101824276508909887E-16, 1.000000000000000000, -0.000000000000000000 ) ) ;
#20255=DIRECTION ( 'NONE',  ( -1.224646799147353207E-16, -1.349345573449484691E-32, 1.000000000000000000 ) ) ;
#20279=ORIENTED_EDGE ( 'NONE', *, *, #7161, .T. ) ;
#20280=DIRECTION ( 'NONE',  ( -1.000000000000000000, 0.000000000000000000, 0.000000000000000000 ) ) ;
#20281=DIRECTION ( 'NONE',  ( -1.000000000000000000, 0.000000000000000000, 0.000000000000000000 ) ) ;
#20293=LINE ( 'NONE', #25720, #24636 ) ;
#20297=DIRECTION ( 'NONE',  ( -1.000000000000000000, 0.000000000000000000, 0.000000000000000000 ) ) ;
#20298=ORIENTED_EDGE ( 'NONE', *, *, #13597, .F. ) ;
#20305=AXIS2_PLACEMENT_3D ( 'NONE', #19381, #11610, #29006 ) ;
#20307=DIRECTION ( 'NONE',  ( -1.000000000000000000, 0.000000000000000000, 0.000000000000000000 ) ) ;
#20309=TOROIDAL_SURFACE ( 'NONE', #29767, 12.40141737965286239, 0.1250000000000005551 ) ;
#20310=ORIENTED_EDGE ( 'NONE', *, *, #4793, .T. ) ;
#20311=AXIS2_PLACEMENT_3D ( 'NONE', #10269, #30610, #729 ) ;
#20318=DIRECTION ( 'NONE',  ( 1.000000000000000000, 0.000000000000000000, 0.000000000000000000 ) ) ;
#20319=LINE ( 'NONE', #18505, #19009 ) ;
#20321=EDGE_LOOP ( 'NONE', ( #12624, #15461, #22174, #24720 ) ) ;
#20325=TOROIDAL_SURFACE ( 'NONE', #11954, 12.40141737965287660, 0.1250000000000007772 ) ;
#20326=ORIENTED_EDGE ( 'NONE', *, *, #18612, .F. ) ;
#20330=AXIS2_PLACEMENT_3D ( 'NONE', #2540, #18270, #22554 ) ;
#20331=AXIS2_PLACEMENT_3D ( 'NONE', #30092, #15464, #15145 ) ;
#20335=ORIENTED_EDGE ( 'NONE', *, *, #17828, .F. ) ;
#20338=EDGE_CURVE ( 'NONE', #23854, #3483, #6140, .T. ) ;
#20343=DIRECTION ( 'NONE',  ( 0.000000000000000000, -0.000000000000000000, -1.000000000000000000 ) ) ;
#20349=ORIENTED_EDGE ( 'NONE', *, *, #12358, .T. ) ;
#20353=DIRECTION ( 'NONE',  ( -1.000000000000000000, -1.101824276508909764E-16, 0.000000000000000000 ) ) ;
#20356=VECTOR ( 'NONE', #11033, 1000.000000000000000 ) ;
#20361=DIRECTION ( 'NONE',  ( -1.101824276508909887E-16, 1.000000000000000000, -0.000000000000000000 ) ) ;
#20363=FACE_OUTER_BOUND ( 'NONE', #172, .T. ) ;
#20366=CARTESIAN_POINT ( 'NONE',  ( 8.823509210239581790, 31.84164230456639544, 47.04930799450051637 ) ) ;
#20369=VERTEX_POINT ( 'NONE', #10909 ) ;
#20373=CARTESIAN_POINT ( 'NONE',  ( 21.09992658989238734, 38.56284415653841791, 47.04930799450051637 ) ) ;
#20376=AXIS2_PLACEMENT_3D ( 'NONE', #812, #28874, #16384 ) ;
#20378=DIRECTION ( 'NONE',  ( -1.000000000000000000, -1.101824276508909887E-16, 0.000000000000000000 ) ) ;
#20379=EDGE_CURVE ( 'NONE', #24621, #23072, #26568, .T. ) ;
#20394=DIRECTION ( 'NONE',  ( -1.000000000000000000, 0.000000000000000000, 0.000000000000000000 ) ) ;
#20398=TOROIDAL_SURFACE ( 'NONE', #22502, 12.61792373059897088, 0.1249999999999973216 ) ;
#20403=EDGE_CURVE ( 'NONE', #6908, #272, #9795, .T. ) ;
#20409=DIRECTION ( 'NONE',  ( -1.000000000000000000, 0.000000000000000000, 0.000000000000000000 ) ) ;
#20410=CIRCLE ( 'NONE', #1039, 12.62506659569710266 ) ;
#20411=DIRECTION ( 'NONE',  ( -1.101824276508909887E-16, 1.000000000000000000, -0.000000000000000000 ) ) ;
#20417=CARTESIAN_POINT ( 'NONE',  ( 21.09992658989239089, 27.96664230456639899, 47.04930799450051637 ) ) ;
#20421=FACE_OUTER_BOUND ( 'NONE', #7509, .T. ) ;
#20427=TOROIDAL_SURFACE ( 'NONE', #24623, 12.40141737965282687, 0.1250000000000004718 ) ;
#20430=VERTEX_POINT ( 'NONE', #31892 ) ;
#20433=CIRCLE ( 'NONE', #26215, 12.36707279061065101 ) ;
#20434=ORIENTED_EDGE ( 'NONE', *, *, #12952, .T. ) ;
#20435=CIRCLE ( 'NONE', #29364, 12.62506659569710266 ) ;
#20443=EDGE_CURVE ( 'NONE', #14267, #1229, #8230, .T. ) ;
#20444=TOROIDAL_SURFACE ( 'NONE', #28842, 12.40141737965280733, 0.1250000000000013878 ) ;
#20445=EDGE_CURVE ( 'NONE', #3912, #30065, #888, .T. ) ;
#20446=EDGE_LOOP ( 'NONE', ( #17811, #14025, #10670, #21072 ) ) ;
#20448=EDGE_CURVE ( 'NONE', #14608, #29845, #16593, .T. ) ;
#20454=DIRECTION ( 'NONE',  ( -1.000000000000000000, -1.101824276508910010E-16, 0.000000000000000000 ) ) ;
#20455=CARTESIAN_POINT ( 'NONE',  ( 33.50134396954523908, 27.34164230456639544, 47.04930799450051637 ) ) ;
#20456=DIRECTION ( 'NONE',  ( -1.101824276508909887E-16, 1.000000000000000000, -0.000000000000000000 ) ) ;
#20457=ORIENTED_EDGE ( 'NONE', *, *, #8060, .T. ) ;
#20459=CIRCLE ( 'NONE', #26736, 0.1250000000000001110 ) ;
#20460=AXIS2_PLACEMENT_3D ( 'NONE', #10121, #24435, #22744 ) ;
#20463=DIRECTION ( 'NONE',  ( -1.000000000000000000, -1.101824276508909887E-16, 0.000000000000000000 ) ) ;
#20467=DIRECTION ( 'NONE',  ( 0.000000000000000000, -0.000000000000000000, -1.000000000000000000 ) ) ;
#20477=DIRECTION ( 'NONE',  ( -1.000000000000000000, -1.101824276508909887E-16, 0.000000000000000000 ) ) ;
#20480=EDGE_CURVE ( 'NONE', #21385, #27343, #28165, .T. ) ;
#20481=CIRCLE ( 'NONE', #28883, 12.36707279061065279 ) ;
#20482=EDGE_CURVE ( 'NONE', #14283, #112, #23457, .T. ) ;
#20485=VECTOR ( 'NONE', #3123, 1000.000000000000000 ) ;
#20492=DIRECTION ( 'NONE',  ( -1.224646799147353207E-16, -1.349345573449484691E-32, 1.000000000000000000 ) ) ;
#20496=ORIENTED_EDGE ( 'NONE', *, *, #30948, .F. ) ;
#20498=AXIS2_PLACEMENT_3D ( 'NONE', #25468, #19884, #30564 ) ;
#20501=CARTESIAN_POINT ( 'NONE',  ( 8.482002859293416464, 25.96664230456639899, 47.04930799450051637 ) ) ;
#20502=DIRECTION ( 'NONE',  ( -1.000000000000000000, 0.000000000000000000, 0.000000000000000000 ) ) ;
#20505=ORIENTED_EDGE ( 'NONE', *, *, #16843, .T. ) ;
#20512=CARTESIAN_POINT ( 'NONE',  ( 8.474859994195286461, 25.84143805560860940, 47.04930799450051637 ) ) ;
#20513=VECTOR ( 'NONE', #28458, 1000.000000000000000 ) ;
#20517=ORIENTED_EDGE ( 'NONE', *, *, #31083, .T. ) ;
#20522=CARTESIAN_POINT ( 'NONE',  ( 21.09992658989239089, 27.34164230456639544, 47.04930799450051637 ) ) ;
#20535=DIRECTION ( 'NONE',  ( 0.000000000000000000, -0.000000000000000000, -1.000000000000000000 ) ) ;
#20536=DIRECTION ( 'NONE',  ( -1.101824276508909887E-16, 1.000000000000000000, -0.000000000000000000 ) ) ;
#20548=ORIENTED_EDGE ( 'NONE', *, *, #2984, .T. ) ;
#20551=CARTESIAN_POINT ( 'NONE',  ( 21.09992658989239089, 26.59164230456639899, 47.04930799450051637 ) ) ;
#20564=EDGE_CURVE ( 'NONE', #11017, #7677, #21340, .T. ) ;
#20565=EDGE_CURVE ( 'NONE', #9081, #2041, #2506, .T. ) ;
#20566=AXIS2_PLACEMENT_3D ( 'NONE', #23328, #10707, #25625 ) ;
#20568=EDGE_CURVE ( 'NONE', #27923, #104, #30787, .T. ) ;
#20576=DIRECTION ( 'NONE',  ( -1.000000000000000000, 0.000000000000000000, 0.000000000000000000 ) ) ;
#20579=LINE ( 'NONE', #3169, #32041 ) ;
#20580=DIRECTION ( 'NONE',  ( -1.000000000000000000, 0.000000000000000000, 0.000000000000000000 ) ) ;
#20581=VERTEX_POINT ( 'NONE', #363 ) ;
#20583=CARTESIAN_POINT ( 'NONE',  ( 8.482002859293801933, 31.46664230456641675, 47.04930799450051637 ) ) ;
#20589=FACE_OUTER_BOUND ( 'NONE', #30887, .T. ) ;
#20599=ORIENTED_EDGE ( 'NONE', *, *, #4418, .T. ) ;
#20604=CIRCLE ( 'NONE', #6452, 0.1250000000000001110 ) ;
#20607=LINE ( 'NONE', #22905, #25717 ) ;
#20608=DIRECTION ( 'NONE',  ( -1.101824276508909887E-16, 1.000000000000000000, -0.000000000000000000 ) ) ;
#20613=AXIS2_PLACEMENT_3D ( 'NONE', #13263, #13418, #8005 ) ;
#20619=VERTEX_POINT ( 'NONE', #13014 ) ;
#20620=DIRECTION ( 'NONE',  ( -1.101824276508909887E-16, 1.000000000000000000, -0.000000000000000000 ) ) ;
#20623=CARTESIAN_POINT ( 'NONE',  ( 8.698509210239576461, 31.34164230456639544, 47.04930799450051637 ) ) ;
#20624=EDGE_LOOP ( 'NONE', ( #25714, #16826, #23209, #13747 ) ) ;
#20627=CARTESIAN_POINT ( 'NONE',  ( 8.482002859293396924, 24.21664230456639899, 47.04930799450051637 ) ) ;
#20628=DIRECTION ( 'NONE',  ( -1.000000000000000000, -1.101824276508909887E-16, 0.000000000000000000 ) ) ;
#20632=AXIS2_PLACEMENT_3D ( 'NONE', #7685, #32467, #2908 ) ;
#20633=DIRECTION ( 'NONE',  ( -1.101824276508909887E-16, 1.000000000000000000, -0.000000000000000000 ) ) ;
#20635=ORIENTED_EDGE ( 'NONE', *, *, #10278, .F. ) ;
#20637=EDGE_CURVE ( 'NONE', #29330, #1073, #18717, .T. ) ;
#20644=ADVANCED_FACE ( 'NONE', ( #19898 ), #6156, .T. ) ;
#20645=VERTEX_POINT ( 'NONE', #15947 ) ;
#20646=CIRCLE ( 'NONE', #13828, 12.62506659569710266 ) ;
#20648=ORIENTED_EDGE ( 'NONE', *, *, #29691, .F. ) ;
#20651=VERTEX_POINT ( 'NONE', #5949 ) ;
#20656=ORIENTED_EDGE ( 'NONE', *, *, #9216, .T. ) ;
#20658=VERTEX_POINT ( 'NONE', #8566 ) ;
#20665=EDGE_CURVE ( 'NONE', #5065, #25423, #28698, .T. ) ;
#20667=EDGE_LOOP ( 'NONE', ( #25531, #9516, #8715, #15515 ) ) ;
#20668=DIRECTION ( 'NONE',  ( -1.000000000000000000, 0.000000000000000000, 0.000000000000000000 ) ) ;
#20669=CARTESIAN_POINT ( 'NONE',  ( 33.71785032049098874, 30.46664230456641675, 47.04930799450051637 ) ) ;
#20670=EDGE_CURVE ( 'NONE', #1027, #23957, #22388, .T. ) ;
#20678=EDGE_CURVE ( 'NONE', #8602, #26085, #27133, .T. ) ;
#20680=ORIENTED_EDGE ( 'NONE', *, *, #4783, .T. ) ;
#20685=CIRCLE ( 'NONE', #12866, 12.62506659569710266 ) ;
#20697=CARTESIAN_POINT ( 'NONE',  ( 21.09992658989239089, 27.09164230456639899, 47.04930799450051637 ) ) ;
#20698=DIRECTION ( 'NONE',  ( -1.101824276508909887E-16, 1.000000000000000000, -0.000000000000000000 ) ) ;
#20705=DIRECTION ( 'NONE',  ( -1.000000000000000000, 0.000000000000000000, 0.000000000000000000 ) ) ;
#20707=ADVANCED_FACE ( 'NONE', ( #8092 ), #3011, .T. ) ;
#20708=FACE_OUTER_BOUND ( 'NONE', #6854, .T. ) ;
#20712=CARTESIAN_POINT ( 'NONE',  ( 33.46699938050304013, 25.96183152705960140, 47.04930799450051637 ) ) ;
#20713=ORIENTED_EDGE ( 'NONE', *, *, #3134, .T. ) ;
#20714=CARTESIAN_POINT ( 'NONE',  ( 33.46699938050304013, 26.72145308207318948, 47.04930799450050927 ) ) ;
#20715=TOROIDAL_SURFACE ( 'NONE', #6560, 12.61792373059898864, 0.1249999999999962669 ) ;
#20720=EDGE_CURVE ( 'NONE', #28434, #28996, #1164, .T. ) ;
#20722=AXIS2_PLACEMENT_3D ( 'NONE', #15016, #10412, #12229 ) ;
#20723=EDGE_LOOP ( 'NONE', ( #21833, #6471, #14922, #5331 ) ) ;
#20724=DIRECTION ( 'NONE',  ( -1.101824276508909887E-16, 1.000000000000000000, -0.000000000000000000 ) ) ;
#20730=AXIS2_PLACEMENT_3D ( 'NONE', #14983, #10222, #29754 ) ;
#20739=CARTESIAN_POINT ( 'NONE',  ( 21.09992658989238734, 31.71183152705962272, 47.04930799450051637 ) ) ;
#20747=ORIENTED_EDGE ( 'NONE', *, *, #23515, .F. ) ;
#20751=ORIENTED_EDGE ( 'NONE', *, *, #2718, .T. ) ;
#20752=DIRECTION ( 'NONE',  ( -1.000000000000000000, 0.000000000000000000, 0.000000000000000000 ) ) ;
#20754=DIRECTION ( 'NONE',  ( -1.000000000000000000, 0.000000000000000000, 0.000000000000000000 ) ) ;
#20755=EDGE_CURVE ( 'NONE', #25773, #4682, #31331, .T. ) ;
#20758=ADVANCED_FACE ( 'NONE', ( #31218 ), #21873, .T. ) ;
#20759=ORIENTED_EDGE ( 'NONE', *, *, #2813, .T. ) ;
#20763=ADVANCED_FACE ( 'NONE', ( #18234 ), #28267, .T. ) ;
#20768=LINE ( 'NONE', #16159, #27568 ) ;
#20771=ORIENTED_EDGE ( 'NONE', *, *, #7201, .F. ) ;
#20773=ORIENTED_EDGE ( 'NONE', *, *, #14682, .F. ) ;
#20774=CYLINDRICAL_SURFACE ( 'NONE', #26694, 12.62506659569710443 ) ;
#20778=EDGE_LOOP ( 'NONE', ( #8551, #26019, #1751, #15645 ) ) ;
#20779=DIRECTION ( 'NONE',  ( -1.000000000000000000, 0.000000000000000000, 0.000000000000000000 ) ) ;
#20795=AXIS2_PLACEMENT_3D ( 'NONE', #24643, #19710, #22004 ) ;
#20797=ADVANCED_FACE ( 'NONE', ( #21831 ), #19764, .T. ) ;
#20799=EDGE_LOOP ( 'NONE', ( #8564, #12599, #6897, #6958 ) ) ;
#20807=CARTESIAN_POINT ( 'NONE',  ( 8.474859994195286461, 27.34143805560860940, 47.04930799450051637 ) ) ;
#20808=AXIS2_PLACEMENT_3D ( 'NONE', #14372, #11410, #6816 ) ;
#20812=DIRECTION ( 'NONE',  ( -1.000000000000000000, -1.101824276508909887E-16, 0.000000000000000000 ) ) ;
#20817=CARTESIAN_POINT ( 'NONE',  ( 33.72499318558949710, 29.84143805560861296, 47.04930799450051637 ) ) ;
#20828=CARTESIAN_POINT ( 'NONE',  ( 21.09992658989239089, 29.09164230456639899, 47.04930799450051637 ) ) ;
#20830=DIRECTION ( 'NONE',  ( -1.101824276508909887E-16, 1.000000000000000000, -0.000000000000000000 ) ) ;
#20832=VERTEX_POINT ( 'NONE', #18877 ) ;
#20835=EDGE_CURVE ( 'NONE', #28214, #19781, #23980, .T. ) ;
#20843=VECTOR ( 'NONE', #4933, 1000.000000000000227 ) ;
#20845=ORIENTED_EDGE ( 'NONE', *, *, #20448, .T. ) ;
#20847=CIRCLE ( 'NONE', #16139, 0.1250000000000001110 ) ;
#20849=FACE_OUTER_BOUND ( 'NONE', #8980, .T. ) ;
#20857=DIRECTION ( 'NONE',  ( -1.000000000000000000, 0.000000000000000000, 0.000000000000000000 ) ) ;
#20866=ORIENTED_EDGE ( 'NONE', *, *, #19696, .T. ) ;
#20869=ORIENTED_EDGE ( 'NONE', *, *, #20565, .T. ) ;
#20875=AXIS2_PLACEMENT_3D ( 'NONE', #16297, #18590, #10904 ) ;
#20876=AXIS2_PLACEMENT_3D ( 'NONE', #8325, #18322, #5876 ) ;
#20880=DIRECTION ( 'NONE',  ( -1.101824276508909887E-16, 1.000000000000000000, -0.000000000000000000 ) ) ;
#20882=ADVANCED_FACE ( 'NONE', ( #25762 ), #25597, .F. ) ;
#20883=EDGE_LOOP ( 'NONE', ( #31106, #30994, #12215, #13749 ) ) ;
#20887=VECTOR ( 'NONE', #19346, 1000.000000000000000 ) ;
#20888=EDGE_CURVE ( 'NONE', #11938, #7606, #8801, .T. ) ;
#20890=EDGE_LOOP ( 'NONE', ( #5260, #8871, #22495, #18924 ) ) ;
#20893=AXIS2_PLACEMENT_3D ( 'NONE', #26110, #11499, #3954 ) ;
#20897=VERTEX_POINT ( 'NONE', #23137 ) ;
#20902=AXIS2_PLACEMENT_3D ( 'NONE', #27943, #3308, #25949 ) ;
#20913=ORIENTED_EDGE ( 'NONE', *, *, #19059, .T. ) ;
#20917=AXIS2_PLACEMENT_3D ( 'NONE', #4411, #2551, #20112 ) ;
#20920=CIRCLE ( 'NONE', #22574, 12.36707279061065279 ) ;
#20927=ORIENTED_EDGE ( 'NONE', *, *, #20564, .T. ) ;
#20928=ADVANCED_FACE ( 'NONE', ( #8692 ), #23623, .F. ) ;
#20929=DIRECTION ( 'NONE',  ( -1.000000000000000000, 0.000000000000000000, 0.000000000000000000 ) ) ;
#20930=DIRECTION ( 'NONE',  ( -1.101824276508909887E-16, 1.000000000000000000, -0.000000000000000000 ) ) ;
#20932=DIRECTION ( 'NONE',  ( -1.101824276508909887E-16, 1.000000000000000000, -0.000000000000000000 ) ) ;
#20933=VERTEX_POINT ( 'NONE', #23940 ) ;
#20938=CIRCLE ( 'NONE', #12017, 12.36707279061065101 ) ;
#20939=ORIENTED_EDGE ( 'NONE', *, *, #8890, .T. ) ;
#20940=DIRECTION ( 'NONE',  ( -1.000000000000000000, 0.000000000000000000, 0.000000000000000000 ) ) ;
#20943=FACE_OUTER_BOUND ( 'NONE', #20799, .T. ) ;
#20945=CARTESIAN_POINT ( 'NONE',  ( 33.72499318558949710, 31.84184655352418503, 47.04930799450051637 ) ) ;
#20952=CARTESIAN_POINT ( 'NONE',  ( 8.482002859293402253, 24.71664230456639899, 47.04930799450051637 ) ) ;
#20959=ORIENTED_EDGE ( 'NONE', *, *, #24470, .F. ) ;
#20961=CIRCLE ( 'NONE', #28831, 12.36707279061065101 ) ;
#20962=CIRCLE ( 'NONE', #7894, 12.27641737965288371 ) ;
#20963=ORIENTED_EDGE ( 'NONE', *, *, #30871, .T. ) ;
#20968=FACE_OUTER_BOUND ( 'NONE', #24602, .T. ) ;
#20973=AXIS2_PLACEMENT_3D ( 'NONE', #14051, #19112, #24047 ) ;
#20981=DIRECTION ( 'NONE',  ( -1.000000000000000000, 0.000000000000000000, 0.000000000000000000 ) ) ;
#20982=DIRECTION ( 'NONE',  ( 1.000000000000000000, 0.000000000000000000, 0.000000000000000000 ) ) ;
#20985=CARTESIAN_POINT ( 'NONE',  ( 8.474859994195286461, 23.84184655352419213, 47.04930799450051637 ) ) ;
#20991=ORIENTED_EDGE ( 'NONE', *, *, #6994, .T. ) ;
#20993=LINE ( 'NONE', #3276, #7274 ) ;
#20996=AXIS2_PLACEMENT_3D ( 'NONE', #16725, #1967, #4592 ) ;
#21006=VERTEX_POINT ( 'NONE', #11803 ) ;
#21015=VERTEX_POINT ( 'NONE', #19330 ) ;
#21016=VERTEX_POINT ( 'NONE', #24098 ) ;
#21018=CIRCLE ( 'NONE', #21921, 12.62506659569710266 ) ;
#21021=EDGE_LOOP ( 'NONE', ( #1277, #28513, #6062, #24741 ) ) ;
#21025=ORIENTED_EDGE ( 'NONE', *, *, #8746, .F. ) ;
#21029=EDGE_CURVE ( 'NONE', #8460, #13336, #9842, .T. ) ;
#21032=EDGE_CURVE ( 'NONE', #17658, #16985, #28194, .T. ) ;
#21037=CARTESIAN_POINT ( 'NONE',  ( 21.09992658989239089, 28.84164230456639544, 47.04930799450051637 ) ) ;
#21039=ORIENTED_EDGE ( 'NONE', *, *, #13760, .F. ) ;
#21043=AXIS2_PLACEMENT_3D ( 'NONE', #20697, #30725, #18667 ) ;
#21045=VERTEX_POINT ( 'NONE', #21463 ) ;
#21048=DIRECTION ( 'NONE',  ( -1.000000000000000000, 0.000000000000000000, 0.000000000000000000 ) ) ;
#21051=ORIENTED_EDGE ( 'NONE', *, *, #29353, .F. ) ;
#21053=DIRECTION ( 'NONE',  ( -1.000000000000000000, 0.000000000000000000, 0.000000000000000000 ) ) ;
#21055=DIRECTION ( 'NONE',  ( 0.000000000000000000, -0.000000000000000000, -1.000000000000000000 ) ) ;
#21056=CIRCLE ( 'NONE', #24203, 0.1250000000000001110 ) ;
#21064=VERTEX_POINT ( 'NONE', #1784 ) ;
#21065=DIRECTION ( 'NONE',  ( -1.101824276508909887E-16, 1.000000000000000000, -0.000000000000000000 ) ) ;
#21066=DIRECTION ( 'NONE',  ( -1.000000000000000000, -1.101824276508909887E-16, 0.000000000000000000 ) ) ;
#21068=ADVANCED_FACE ( 'NONE', ( #21798 ), #9330, .T. ) ;
#21072=ORIENTED_EDGE ( 'NONE', *, *, #10951, .F. ) ;
#21075=ORIENTED_EDGE ( 'NONE', *, *, #22871, .T. ) ;
#21079=TOROIDAL_SURFACE ( 'NONE', #17411, 12.40141737965283575, 0.1250000000000000278 ) ;
#21080=DIRECTION ( 'NONE',  ( -1.101824276508909887E-16, 1.000000000000000000, -0.000000000000000000 ) ) ;
#21081=DIRECTION ( 'NONE',  ( -1.101824276508909887E-16, 1.000000000000000000, -0.000000000000000000 ) ) ;
#21083=ORIENTED_EDGE ( 'NONE', *, *, #24064, .T. ) ;
#21088=CARTESIAN_POINT ( 'NONE',  ( 21.09992658989239089, 24.59143805560860940, 47.04930799450051637 ) ) ;
#21090=CARTESIAN_POINT ( 'NONE',  ( 33.50134396954523197, 28.34164230456639544, 47.04930799450051637 ) ) ;
#21098=DIRECTION ( 'NONE',  ( -1.101824276508909887E-16, 1.000000000000000000, -0.000000000000000000 ) ) ;
#21104=CIRCLE ( 'NONE', #661, 0.1250000000000001110 ) ;
#21110=AXIS2_PLACEMENT_3D ( 'NONE', #7487, #2874, #14874 ) ;
#21114=AXIS2_PLACEMENT_3D ( 'NONE', #8355, #8682, #20502 ) ;
#21116=CIRCLE ( 'NONE', #9615, 12.36707279061065101 ) ;
#21123=DIRECTION ( 'NONE',  ( -1.000000000000000000, 0.000000000000000000, 0.000000000000000000 ) ) ;
#21125=ORIENTED_EDGE ( 'NONE', *, *, #30401, .T. ) ;
#21126=EDGE_LOOP ( 'NONE', ( #18013, #29909, #12362, #2020 ) ) ;
#21133=CARTESIAN_POINT ( 'NONE',  ( 21.09992658989238734, 38.56284415653841791, 47.04930799450051637 ) ) ;
#21135=LINE ( 'NONE', #29347, #24456 ) ;
#21139=DIRECTION ( 'NONE',  ( -1.101824276508909887E-16, 1.000000000000000000, -0.000000000000000000 ) ) ;
#21145=EDGE_CURVE ( 'NONE', #22098, #29646, #29781, .T. ) ;
#21152=EDGE_CURVE ( 'NONE', #4576, #27738, #906, .T. ) ;
#21156=CYLINDRICAL_SURFACE ( 'NONE', #14684, 12.36707279061065101 ) ;
#21161=CARTESIAN_POINT ( 'NONE',  ( 33.37634396954520355, 30.84164230456639544, 47.04930799450051637 ) ) ;
#21163=DIRECTION ( 'NONE',  ( -1.000000000000000000, 0.000000000000000000, 0.000000000000000000 ) ) ;
#21164=ORIENTED_EDGE ( 'NONE', *, *, #30903, .T. ) ;
#21169=EDGE_LOOP ( 'NONE', ( #27744, #7206, #1628, #23248 ) ) ;
#21170=EDGE_CURVE ( 'NONE', #26283, #1375, #19259, .T. ) ;
#21173=CYLINDRICAL_SURFACE ( 'NONE', #30341, 12.36707279061065101 ) ;
#21182=CIRCLE ( 'NONE', #8616, 12.27641737965281976 ) ;
#21184=AXIS2_PLACEMENT_3D ( 'NONE', #8865, #3947, #13966 ) ;
#21187=AXIS2_PLACEMENT_3D ( 'NONE', #10629, #20620, #30646 ) ;
#21195=CARTESIAN_POINT ( 'NONE',  ( 21.09992658989239089, 29.84184655352422411, 47.04930799450051637 ) ) ;
#21197=CARTESIAN_POINT ( 'NONE',  ( 21.09992658989238734, 32.55121380581068991, 47.04930799450051637 ) ) ;
#21198=VERTEX_POINT ( 'NONE', #5632 ) ;
#21200=LINE ( 'NONE', #18261, #7353 ) ;
#21205=ORIENTED_EDGE ( 'NONE', *, *, #20482, .T. ) ;
#21216=ORIENTED_EDGE ( 'NONE', *, *, #5594, .F. ) ;
#21218=FACE_OUTER_BOUND ( 'NONE', #17460, .T. ) ;
#21220=ORIENTED_EDGE ( 'NONE', *, *, #21032, .T. ) ;
#21221=CARTESIAN_POINT ( 'NONE',  ( 33.50134396954523908, 27.59164230456639544, 47.04930799450051637 ) ) ;
#21222=CARTESIAN_POINT ( 'NONE',  ( 21.09992658989239089, 29.71183152705961561, 47.04930799450051637 ) ) ;
#21223=DIRECTION ( 'NONE',  ( -1.101824276508909887E-16, 1.000000000000000000, -0.000000000000000000 ) ) ;
#21225=ORIENTED_EDGE ( 'NONE', *, *, #16033, .F. ) ;
#21228=EDGE_CURVE ( 'NONE', #460, #4539, #17726, .T. ) ;
#21229=ORIENTED_EDGE ( 'NONE', *, *, #23311, .F. ) ;
#21232=AXIS2_PLACEMENT_3D ( 'NONE', #9526, #14779, #14938 ) ;
#21233=CIRCLE ( 'NONE', #20730, 12.62506659569710443 ) ;
#21236=ADVANCED_FACE ( 'NONE', ( #5478 ), #30838, .T. ) ;
#21240=ADVANCED_FACE ( 'NONE', ( #2520 ), #25494, .T. ) ;
#21247=CARTESIAN_POINT ( 'NONE',  ( 33.46699938050304013, 38.56284415653841791, 47.04930799450051637 ) ) ;
#21251=DIRECTION ( 'NONE',  ( -1.000000000000000000, 0.000000000000000000, 0.000000000000000000 ) ) ;
#21253=DIRECTION ( 'NONE',  ( -1.101824276508909887E-16, 1.000000000000000000, -0.000000000000000000 ) ) ;
#21255=ORIENTED_EDGE ( 'NONE', *, *, #32291, .F. ) ;
#21259=DIRECTION ( 'NONE',  ( -1.101824276508909887E-16, 1.000000000000000000, -0.000000000000000000 ) ) ;
#21261=CARTESIAN_POINT ( 'NONE',  ( 21.09992658989239089, 28.34164230456639544, 47.04930799450051637 ) ) ;
#21265=ORIENTED_EDGE ( 'NONE', *, *, #22934, .T. ) ;
#21267=CIRCLE ( 'NONE', #18642, 12.36707279061065101 ) ;
#21272=ADVANCED_FACE ( 'NONE', ( #10571 ), #28213, .T. ) ;
#21273=AXIS2_PLACEMENT_3D ( 'NONE', #2372, #22713, #24692 ) ;
#21274=ORIENTED_EDGE ( 'NONE', *, *, #913, .T. ) ;
#21275=ORIENTED_EDGE ( 'NONE', *, *, #14449, .F. ) ;
#21278=AXIS2_PLACEMENT_3D ( 'NONE', #13010, #515, #6094 ) ;
#21279=ADVANCED_FACE ( 'NONE', ( #23020 ), #9344, .T. ) ;
#21285=EDGE_LOOP ( 'NONE', ( #21371, #9924, #13337, #13151 ) ) ;
#21287=DIRECTION ( 'NONE',  ( -1.101824276508909887E-16, 1.000000000000000000, -0.000000000000000000 ) ) ;
#21288=ADVANCED_FACE ( 'NONE', ( #28125 ), #17459, .T. ) ;
#21290=DIRECTION ( 'NONE',  ( -1.000000000000000000, -1.101824276508910010E-16, 0.000000000000000000 ) ) ;
#21301=DIRECTION ( 'NONE',  ( 1.000000000000000000, 0.000000000000000000, 0.000000000000000000 ) ) ;
#21302=DIRECTION ( 'NONE',  ( -1.000000000000000000, -1.101824276508909887E-16, 0.000000000000000000 ) ) ;
#21303=ORIENTED_EDGE ( 'NONE', *, *, #14764, .T. ) ;
#21307=CARTESIAN_POINT ( 'NONE',  ( 8.482002859293437780, 27.96664230456639899, 47.04930799450051637 ) ) ;
#21312=CARTESIAN_POINT ( 'NONE',  ( 33.46699938050304013, 26.21183152705960140, 47.04930799450051637 ) ) ;
#21315=ORIENTED_EDGE ( 'NONE', *, *, #31062, .F. ) ;
#21316=DIRECTION ( 'NONE',  ( -1.000000000000000000, 0.000000000000000000, 0.000000000000000000 ) ) ;
#21323=EDGE_LOOP ( 'NONE', ( #19970, #16972, #2843, #20120 ) ) ;
#21326=ADVANCED_FACE ( 'NONE', ( #5323 ), #8294, .T. ) ;
#21328=EDGE_LOOP ( 'NONE', ( #26193, #19171, #27811, #19478 ) ) ;
#21336=ORIENTED_EDGE ( 'NONE', *, *, #3852, .F. ) ;
#21339=FACE_OUTER_BOUND ( 'NONE', #12953, .T. ) ;
#21340=CIRCLE ( 'NONE', #12459, 12.62506659569710266 ) ;
#21344=CYLINDRICAL_SURFACE ( 'NONE', #9295, 12.36707279061065101 ) ;
#21345=CARTESIAN_POINT ( 'NONE',  ( 21.09992658989238734, 38.56284415653841791, 47.04930799450051637 ) ) ;
#21348=AXIS2_PLACEMENT_3D ( 'NONE', #7625, #23026, #27318 ) ;
#21351=DIRECTION ( 'NONE',  ( -1.000000000000000000, 0.000000000000000000, 0.000000000000000000 ) ) ;
#21357=EDGE_CURVE ( 'NONE', #25631, #7606, #15114, .T. ) ;
#21358=EDGE_CURVE ( 'NONE', #27840, #26531, #10923, .T. ) ;
#21359=FACE_OUTER_BOUND ( 'NONE', #13960, .T. ) ;
#21363=CARTESIAN_POINT ( 'NONE',  ( 21.09992658989239089, 26.09184655352419213, 47.04930799450051637 ) ) ;
#21371=ORIENTED_EDGE ( 'NONE', *, *, #11433, .F. ) ;
#21372=DIRECTION ( 'NONE',  ( -1.000000000000000000, 0.000000000000000000, 0.000000000000000000 ) ) ;
#21373=CARTESIAN_POINT ( 'NONE',  ( 8.474859994195286461, 25.09184655352419213, 47.04930799450051637 ) ) ;
#21375=AXIS2_PLACEMENT_3D ( 'NONE', #16383, #6699, #6871 ) ;
#21384=ORIENTED_EDGE ( 'NONE', *, *, #23632, .F. ) ;
#21385=VERTEX_POINT ( 'NONE', #31070 ) ;
#21386=ADVANCED_FACE ( 'NONE', ( #8730 ), #13544, .T. ) ;
#21392=CARTESIAN_POINT ( 'NONE',  ( 33.72499318558949710, 24.59143805560860940, 47.04930799450051637 ) ) ;
#21393=CARTESIAN_POINT ( 'NONE',  ( 21.09992658989238734, 38.56284415653841791, 47.04930799450051637 ) ) ;
#21394=DIRECTION ( 'NONE',  ( -1.101824276508909887E-16, 1.000000000000000000, -0.000000000000000000 ) ) ;
#21396=AXIS2_PLACEMENT_3D ( 'NONE', #17069, #12493, #29888 ) ;
#21401=EDGE_CURVE ( 'NONE', #17692, #21567, #4085, .T. ) ;
#21402=ORIENTED_EDGE ( 'NONE', *, *, #27994, .T. ) ;
#21403=DIRECTION ( 'NONE',  ( -1.224646799147353207E-16, -1.349345573449484691E-32, 1.000000000000000000 ) ) ;
#21404=CYLINDRICAL_SURFACE ( 'NONE', #30496, 12.36707279061065279 ) ;
#21407=ORIENTED_EDGE ( 'NONE', *, *, #7537, .T. ) ;
#21416=ORIENTED_EDGE ( 'NONE', *, *, #19337, .T. ) ;
#21421=CIRCLE ( 'NONE', #4585, 0.1249999999999983763 ) ;
#21426=EDGE_CURVE ( 'NONE', #2250, #24311, #19288, .T. ) ;
#21430=ADVANCED_FACE ( 'NONE', ( #11358 ), #3643, .F. ) ;
#21432=EDGE_CURVE ( 'NONE', #10697, #17732, #13198, .T. ) ;
#21435=AXIS2_PLACEMENT_3D ( 'NONE', #31474, #27028, #14076 ) ;
#21438=DIRECTION ( 'NONE',  ( -1.101824276508909887E-16, 1.000000000000000000, -0.000000000000000000 ) ) ;
#21443=EDGE_CURVE ( 'NONE', #15900, #12078, #7782, .T. ) ;
#21445=ORIENTED_EDGE ( 'NONE', *, *, #18427, .T. ) ;
#21449=CIRCLE ( 'NONE', #26198, 12.27641737965285174 ) ;
#21451=FACE_OUTER_BOUND ( 'NONE', #13707, .T. ) ;
#21454=AXIS2_PLACEMENT_3D ( 'NONE', #29194, #26895, #4566 ) ;
#21458=CARTESIAN_POINT ( 'NONE',  ( 21.09992658989239089, 25.09164230456639899, 47.04930799450051637 ) ) ;
#21462=EDGE_LOOP ( 'NONE', ( #13972, #18869, #29440, #11013 ) ) ;
#21463=CARTESIAN_POINT ( 'NONE',  ( 8.474859994195286461, 30.59184655352422411, 47.04930799450051637 ) ) ;
#21472=AXIS2_PLACEMENT_3D ( 'NONE', #19695, #12330, #14792 ) ;
#21475=CIRCLE ( 'NONE', #19918, 0.1249999999999983763 ) ;
#21478=CARTESIAN_POINT ( 'NONE',  ( 8.698509210239521394, 25.59164230456639899, 47.04930799450051637 ) ) ;
#21480=DIRECTION ( 'NONE',  ( -1.000000000000000000, 0.000000000000000000, 0.000000000000000000 ) ) ;
#21483=DIRECTION ( 'NONE',  ( -1.000000000000000000, 0.000000000000000000, 0.000000000000000000 ) ) ;
#21485=ORIENTED_EDGE ( 'NONE', *, *, #32178, .T. ) ;
#21490=CARTESIAN_POINT ( 'NONE',  ( 21.09992658989239089, 24.84184655352419213, 47.04930799450051637 ) ) ;
#21495=DIRECTION ( 'NONE',  ( -1.101824276508909887E-16, 1.000000000000000000, -0.000000000000000000 ) ) ;
#21500=VECTOR ( 'NONE', #30532, 1000.000000000000000 ) ;
#21507=CIRCLE ( 'NONE', #24063, 0.1250000000000001110 ) ;
#21514=DIRECTION ( 'NONE',  ( -1.000000000000000000, 0.000000000000000000, 0.000000000000000000 ) ) ;
#21518=AXIS2_PLACEMENT_3D ( 'NONE', #29797, #27330, #5017 ) ;
#21520=AXIS2_PLACEMENT_3D ( 'NONE', #18161, #18006, #31139 ) ;
#21522=DIRECTION ( 'NONE',  ( -1.101824276508909887E-16, 1.000000000000000000, -0.000000000000000000 ) ) ;
#21523=AXIS2_PLACEMENT_3D ( 'NONE', #24207, #3863, #1228 ) ;
#21526=CARTESIAN_POINT ( 'NONE',  ( 8.732853799281734553, 38.56284415653841791, 47.04930799450051637 ) ) ;
#21528=CARTESIAN_POINT ( 'NONE',  ( 8.474859994195286461, 29.59143805560861296, 47.04930799450051637 ) ) ;
#21530=ORIENTED_EDGE ( 'NONE', *, *, #4528, .F. ) ;
#21533=VECTOR ( 'NONE', #1870, 1000.000000000000000 ) ;
#21534=CARTESIAN_POINT ( 'NONE',  ( 8.474859994195282908, 38.56284415653841791, 47.04930799450051637 ) ) ;
#21536=DIRECTION ( 'NONE',  ( -1.000000000000000000, 0.000000000000000000, 0.000000000000000000 ) ) ;
#21539=CARTESIAN_POINT ( 'NONE',  ( 21.09992658989238734, 38.56284415653841791, 47.04930799450051637 ) ) ;
#21543=DIRECTION ( 'NONE',  ( -1.000000000000000000, -1.101824276508910010E-16, 0.000000000000000000 ) ) ;
#21544=DIRECTION ( 'NONE',  ( -1.224646799147353207E-16, -1.349345573449484691E-32, 1.000000000000000000 ) ) ;
#21545=DIRECTION ( 'NONE',  ( -1.000000000000000000, 0.000000000000000000, 0.000000000000000000 ) ) ;
#21550=ORIENTED_EDGE ( 'NONE', *, *, #6390, .F. ) ;
#21551=AXIS2_PLACEMENT_3D ( 'NONE', #11535, #19065, #11217 ) ;
#21552=VECTOR ( 'NONE', #6327, 1000.000000000000000 ) ;
#21557=CIRCLE ( 'NONE', #5975, 12.27641737965286772 ) ;
#21560=CARTESIAN_POINT ( 'NONE',  ( 33.72499318558949000, 38.56284415653841791, 47.04930799450051637 ) ) ;
#21562=FACE_OUTER_BOUND ( 'NONE', #12759, .T. ) ;
#21567=VERTEX_POINT ( 'NONE', #1499 ) ;
#21569=CIRCLE ( 'NONE', #3243, 12.36707279061065279 ) ;
#21570=CARTESIAN_POINT ( 'NONE',  ( 8.698509210239548040, 28.09164230456639544, 47.04930799450051637 ) ) ;
#21573=VERTEX_POINT ( 'NONE', #21682 ) ;
#21575=DIRECTION ( 'NONE',  ( -1.101824276508909887E-16, 1.000000000000000000, -0.000000000000000000 ) ) ;
#21576=DIRECTION ( 'NONE',  ( -1.101824276508909887E-16, 1.000000000000000000, -0.000000000000000000 ) ) ;
#21579=DIRECTION ( 'NONE',  ( -1.101824276508909887E-16, 1.000000000000000000, -0.000000000000000000 ) ) ;
#21588=CARTESIAN_POINT ( 'NONE',  ( 21.09992658989239089, 26.59164230456639899, 47.04930799450051637 ) ) ;
#21592=CIRCLE ( 'NONE', #1748, 12.62506659569710266 ) ;
#21596=AXIS2_PLACEMENT_3D ( 'NONE', #28858, #21287, #30840 ) ;
#21603=LINE ( 'NONE', #17001, #13221 ) ;
#21604=AXIS2_PLACEMENT_3D ( 'NONE', #3295, #25943, #16251 ) ;
#21606=CARTESIAN_POINT ( 'NONE',  ( 33.50134396954522487, 28.84164230456639544, 47.04930799450051637 ) ) ;
#21608=CIRCLE ( 'NONE', #8539, 12.36707279061065101 ) ;
#21613=FACE_OUTER_BOUND ( 'NONE', #5482, .T. ) ;
#21614=EDGE_LOOP ( 'NONE', ( #16434, #4904, #13277, #11125 ) ) ;
#21617=EDGE_CURVE ( 'NONE', #1140, #4802, #9665, .T. ) ;
#21618=CARTESIAN_POINT ( 'NONE',  ( 33.71785032049137953, 24.46664230456639899, 47.04930799450051637 ) ) ;
#21620=DIRECTION ( 'NONE',  ( -1.101824276508909887E-16, 1.000000000000000000, -0.000000000000000000 ) ) ;
#21621=DIRECTION ( 'NONE',  ( 0.000000000000000000, -0.000000000000000000, -1.000000000000000000 ) ) ;
#21623=TOROIDAL_SURFACE ( 'NONE', #4342, 12.40141737965284996, 0.1250000000000002776 ) ;
#21638=CYLINDRICAL_SURFACE ( 'NONE', #26685, 12.62506659569710266 ) ;
#21640=AXIS2_PLACEMENT_3D ( 'NONE', #18824, #3905, #11454 ) ;
#21645=ORIENTED_EDGE ( 'NONE', *, *, #30511, .T. ) ;
#21646=CARTESIAN_POINT ( 'NONE',  ( 8.474859994195282908, 38.56284415653841791, 47.04930799450051637 ) ) ;
#21647=DIRECTION ( 'NONE',  ( -1.101824276508909887E-16, 1.000000000000000000, -0.000000000000000000 ) ) ;
#21648=FACE_OUTER_BOUND ( 'NONE', #2076, .T. ) ;
#21656=ORIENTED_EDGE ( 'NONE', *, *, #19250, .T. ) ;
#21657=ADVANCED_FACE ( 'NONE', ( #7902 ), #14920, .T. ) ;
#21660=CIRCLE ( 'NONE', #20613, 12.36707279061065279 ) ;
#21661=DIRECTION ( 'NONE',  ( -1.101824276508909887E-16, 1.000000000000000000, -0.000000000000000000 ) ) ;
#21663=EDGE_LOOP ( 'NONE', ( #21765, #17615, #293, #9661 ) ) ;
#21664=ORIENTED_EDGE ( 'NONE', *, *, #17036, .F. ) ;
#21671=ORIENTED_EDGE ( 'NONE', *, *, #19468, .T. ) ;
#21675=CIRCLE ( 'NONE', #24304, 12.62506659569710443 ) ;
#21676=ORIENTED_EDGE ( 'NONE', *, *, #17597, .F. ) ;
#21677=CARTESIAN_POINT ( 'NONE',  ( 8.732853799281732776, 32.21183152705962272, 47.04930799450051637 ) ) ;
#21679=DIRECTION ( 'NONE',  ( -1.224646799147353207E-16, -1.349345573449484691E-32, 1.000000000000000000 ) ) ;
#21682=CARTESIAN_POINT ( 'NONE',  ( 8.732853799281732776, 23.97145308207319303, 47.04930799450051637 ) ) ;
#21688=DIRECTION ( 'NONE',  ( 0.000000000000000000, -0.000000000000000000, -1.000000000000000000 ) ) ;
#21694=DIRECTION ( 'NONE',  ( -1.101824276508909887E-16, 1.000000000000000000, -0.000000000000000000 ) ) ;
#21698=CARTESIAN_POINT ( 'NONE',  ( 21.09992658989238734, 38.56284415653841791, 47.04930799450051637 ) ) ;
#21704=ORIENTED_EDGE ( 'NONE', *, *, #13951, .T. ) ;
#21707=DIRECTION ( 'NONE',  ( -1.101824276508909887E-16, 1.000000000000000000, -0.000000000000000000 ) ) ;
#21708=ORIENTED_EDGE ( 'NONE', *, *, #18018, .T. ) ;
#21712=CARTESIAN_POINT ( 'NONE',  ( 33.50134396954522487, 28.59164230456639544, 47.04930799450051637 ) ) ;
#21714=AXIS2_PLACEMENT_3D ( 'NONE', #24161, #11699, #26948 ) ;
#21718=ORIENTED_EDGE ( 'NONE', *, *, #17874, .F. ) ;
#21726=AXIS2_PLACEMENT_3D ( 'NONE', #13330, #13002, #5932 ) ;
#21727=CARTESIAN_POINT ( 'NONE',  ( 8.698509210239532052, 26.59164230456639899, 47.04930799450051637 ) ) ;
#21728=CIRCLE ( 'NONE', #12309, 12.27641737965285529 ) ;
#21729=AXIS2_PLACEMENT_3D ( 'NONE', #2419, #22421, #2573 ) ;
#21733=AXIS2_PLACEMENT_3D ( 'NONE', #15555, #628, #10660 ) ;
#21734=CARTESIAN_POINT ( 'NONE',  ( 21.09992658989239089, 23.84164230456639544, 47.04930799450051637 ) ) ;
#21739=CARTESIAN_POINT ( 'NONE',  ( 21.09992658989239089, 24.21664230456639899, 47.04930799450051637 ) ) ;
#21741=DIRECTION ( 'NONE',  ( -1.101824276508909887E-16, 1.000000000000000000, -0.000000000000000000 ) ) ;
#21743=CARTESIAN_POINT ( 'NONE',  ( 33.37634396954518223, 32.34164230456639899, 47.04930799450051637 ) ) ;
#21747=EDGE_CURVE ( 'NONE', #32154, #20897, #26429, .T. ) ;
#21749=DIRECTION ( 'NONE',  ( -1.101824276508909887E-16, 1.000000000000000000, -0.000000000000000000 ) ) ;
#21750=CARTESIAN_POINT ( 'NONE',  ( 8.732853799281734553, 38.56284415653841791, 47.04930799450051637 ) ) ;
#21755=AXIS2_PLACEMENT_3D ( 'NONE', #3567, #947, #11139 ) ;
#21761=ORIENTED_EDGE ( 'NONE', *, *, #29250, .T. ) ;
#21765=ORIENTED_EDGE ( 'NONE', *, *, #21029, .F. ) ;
#21766=DIRECTION ( 'NONE',  ( -1.101824276508909887E-16, 1.000000000000000000, -0.000000000000000000 ) ) ;
#21768=DIRECTION ( 'NONE',  ( 0.000000000000000000, -0.000000000000000000, -1.000000000000000000 ) ) ;
#21770=VERTEX_POINT ( 'NONE', #21312 ) ;
#21776=ORIENTED_EDGE ( 'NONE', *, *, #5761, .T. ) ;
#21779=DIRECTION ( 'NONE',  ( -1.101824276508909887E-16, 1.000000000000000000, -0.000000000000000000 ) ) ;
#21780=CARTESIAN_POINT ( 'NONE',  ( 21.09992658989239089, 24.46183152705960140, 47.04930799450051637 ) ) ;
#21782=EDGE_CURVE ( 'NONE', #3066, #3389, #30640, .T. ) ;
#21788=EDGE_CURVE ( 'NONE', #3389, #9948, #757, .T. ) ;
#21793=FACE_OUTER_BOUND ( 'NONE', #28889, .T. ) ;
#21794=AXIS2_PLACEMENT_3D ( 'NONE', #3201, #5518, #23235 ) ;
#21797=ORIENTED_EDGE ( 'NONE', *, *, #15559, .T. ) ;
#21798=FACE_OUTER_BOUND ( 'NONE', #19706, .T. ) ;
#21809=DIRECTION ( 'NONE',  ( -1.000000000000000000, 0.000000000000000000, 0.000000000000000000 ) ) ;
#21811=CIRCLE ( 'NONE', #6104, 12.27641737965284996 ) ;
#21814=CARTESIAN_POINT ( 'NONE',  ( 33.46699938050304013, 38.56284415653841791, 47.04930799450051637 ) ) ;
#21816=ORIENTED_EDGE ( 'NONE', *, *, #13987, .T. ) ;
#21824=EDGE_LOOP ( 'NONE', ( #5744, #3427, #30177, #6885 ) ) ;
#21826=CYLINDRICAL_SURFACE ( 'NONE', #25495, 12.62506659569710443 ) ;
#21827=CIRCLE ( 'NONE', #15535, 0.1250000000000001110 ) ;
#21831=FACE_OUTER_BOUND ( 'NONE', #23723, .T. ) ;
#21832=DIRECTION ( 'NONE',  ( 1.000000000000000000, 0.000000000000000000, 0.000000000000000000 ) ) ;
#21833=ORIENTED_EDGE ( 'NONE', *, *, #1621, .F. ) ;
#21834=FACE_OUTER_BOUND ( 'NONE', #21169, .T. ) ;
#21840=ORIENTED_EDGE ( 'NONE', *, *, #5946, .F. ) ;
#21844=CIRCLE ( 'NONE', #18697, 0.1249999999999983763 ) ;
#21850=DIRECTION ( 'NONE',  ( -1.101824276508909887E-16, 1.000000000000000000, -0.000000000000000000 ) ) ;
#21854=CARTESIAN_POINT ( 'NONE',  ( 21.09992658989239089, 28.09164230456639544, 47.04930799450051637 ) ) ;
#21856=DIRECTION ( 'NONE',  ( -1.101824276508909887E-16, 1.000000000000000000, -0.000000000000000000 ) ) ;
#21858=EDGE_CURVE ( 'NONE', #32154, #13543, #28060, .T. ) ;
#21859=EDGE_LOOP ( 'NONE', ( #19736, #27559, #2510, #7063 ) ) ;
#21864=ORIENTED_EDGE ( 'NONE', *, *, #31430, .F. ) ;
#21865=CARTESIAN_POINT ( 'NONE',  ( 8.698509210239585343, 32.09164230456639899, 47.04930799450051637 ) ) ;
#21866=AXIS2_PLACEMENT_3D ( 'NONE', #3969, #24312, #28926 ) ;
#21870=ORIENTED_EDGE ( 'NONE', *, *, #4750, .F. ) ;
#21873=TOROIDAL_SURFACE ( 'NONE', #25562, 12.40141737965281621, 0.1250000000000009159 ) ;
#21879=ORIENTED_EDGE ( 'NONE', *, *, #2737, .T. ) ;
#21884=EDGE_CURVE ( 'NONE', #19026, #13441, #8124, .T. ) ;
#21885=ORIENTED_EDGE ( 'NONE', *, *, #21029, .T. ) ;
#21890=ORIENTED_EDGE ( 'NONE', *, *, #17286, .T. ) ;
#21891=CARTESIAN_POINT ( 'NONE',  ( 33.50134396954528171, 23.59164230456639544, 47.04930799450051637 ) ) ;
#21893=DIRECTION ( 'NONE',  ( 0.000000000000000000, -0.000000000000000000, -1.000000000000000000 ) ) ;
#21899=CARTESIAN_POINT ( 'NONE',  ( 33.72499318558949710, 27.59184655352419568, 47.04930799450051637 ) ) ;
#21902=DIRECTION ( 'NONE',  ( -1.224646799147353207E-16, -1.349345573449484691E-32, 1.000000000000000000 ) ) ;
#21905=DIRECTION ( 'NONE',  ( -1.000000000000000000, 0.000000000000000000, 0.000000000000000000 ) ) ;
#21906=ORIENTED_EDGE ( 'NONE', *, *, #7680, .T. ) ;
#21908=FACE_OUTER_BOUND ( 'NONE', #23341, .T. ) ;
#21911=DIRECTION ( 'NONE',  ( -1.101824276508909887E-16, 1.000000000000000000, -0.000000000000000000 ) ) ;
#21912=ORIENTED_EDGE ( 'NONE', *, *, #10892, .T. ) ;
#21914=AXIS2_PLACEMENT_3D ( 'NONE', #21345, #20880, #13670 ) ;
#21916=CIRCLE ( 'NONE', #7784, 12.27641737965288726 ) ;
#21917=VERTEX_POINT ( 'NONE', #24277 ) ;
#21918=TOROIDAL_SURFACE ( 'NONE', #6188, 12.61792373059895311, 0.1249999999999983485 ) ;
#21921=AXIS2_PLACEMENT_3D ( 'NONE', #4974, #17104, #2346 ) ;
#21923=CARTESIAN_POINT ( 'NONE',  ( 21.09992658989238734, 38.56284415653841791, 47.04930799450051637 ) ) ;
#21924=VERTEX_POINT ( 'NONE', #1793 ) ;
#21925=VERTEX_POINT ( 'NONE', #1947 ) ;
#21927=CARTESIAN_POINT ( 'NONE',  ( 21.09992658989239089, 26.59143805560860940, 47.04930799450051637 ) ) ;
#21929=LINE ( 'NONE', #7506, #22706 ) ;
#21933=ORIENTED_EDGE ( 'NONE', *, *, #19658, .F. ) ;
#21935=DIRECTION ( 'NONE',  ( -1.000000000000000000, 0.000000000000000000, 0.000000000000000000 ) ) ;
#21940=CARTESIAN_POINT ( 'NONE',  ( 21.09992658989239089, 27.09143805560860940, 47.04930799450051637 ) ) ;
#21949=CARTESIAN_POINT ( 'NONE',  ( 21.09992658989238734, 38.56284415653841791, 47.04930799450051637 ) ) ;
#21951=ORIENTED_EDGE ( 'NONE', *, *, #8229, .F. ) ;
#21953=DIRECTION ( 'NONE',  ( -1.000000000000000000, 0.000000000000000000, 0.000000000000000000 ) ) ;
#21955=CIRCLE ( 'NONE', #16730, 12.62506659569710266 ) ;
#21959=EDGE_CURVE ( 'NONE', #22635, #3066, #26995, .T. ) ;
#21961=EDGE_CURVE ( 'NONE', #30111, #8095, #29627, .T. ) ;
#21963=CARTESIAN_POINT ( 'NONE',  ( 21.09992658989239089, 29.59164230456639899, 47.04930799450051637 ) ) ;
#21964=CARTESIAN_POINT ( 'NONE',  ( 8.482002859293439556, 28.21664230456639899, 47.04930799450051637 ) ) ;
#21965=DIRECTION ( 'NONE',  ( -1.101824276508909887E-16, 1.000000000000000000, -0.000000000000000000 ) ) ;
#21968=CYLINDRICAL_SURFACE ( 'NONE', #16709, 12.36707279061065279 ) ;
#21969=DIRECTION ( 'NONE',  ( -1.000000000000000000, 0.000000000000000000, 0.000000000000000000 ) ) ;
#21972=VERTEX_POINT ( 'NONE', #1459 ) ;
#21974=CARTESIAN_POINT ( 'NONE',  ( 21.09992658989239089, 28.96183152705961206, 47.04930799450051637 ) ) ;
#21976=DIRECTION ( 'NONE',  ( 1.000000000000000000, 0.000000000000000000, 0.000000000000000000 ) ) ;
#21980=ORIENTED_EDGE ( 'NONE', *, *, #17148, .T. ) ;
#21985=CIRCLE ( 'NONE', #7858, 0.1250000000000001110 ) ;
#21987=ORIENTED_EDGE ( 'NONE', *, *, #19877, .T. ) ;
#21995=CIRCLE ( 'NONE', #16747, 12.36707279061065101 ) ;
#22001=DIRECTION ( 'NONE',  ( -1.101824276508909887E-16, 1.000000000000000000, -0.000000000000000000 ) ) ;
#22002=EDGE_CURVE ( 'NONE', #593, #22606, #11813, .T. ) ;
#22004=DIRECTION ( 'NONE',  ( -1.000000000000000000, 0.000000000000000000, 0.000000000000000000 ) ) ;
#22008=CARTESIAN_POINT ( 'NONE',  ( 33.72499318558949710, 26.34143805560860940, 47.04930799450051637 ) ) ;
#22016=FACE_OUTER_BOUND ( 'NONE', #11574, .T. ) ;
#22028=EDGE_LOOP ( 'NONE', ( #9412, #8456, #2189, #29809 ) ) ;
#22029=CARTESIAN_POINT ( 'NONE',  ( 21.09992658989239089, 27.59184655352419568, 47.04930799450051637 ) ) ;
#22032=VERTEX_POINT ( 'NONE', #32325 ) ;
#22041=ORIENTED_EDGE ( 'NONE', *, *, #15559, .F. ) ;
#22048=CIRCLE ( 'NONE', #16285, 12.62506659569710266 ) ;
#22049=ADVANCED_FACE ( 'NONE', ( #20160 ), #25430, .T. ) ;
#22055=AXIS2_PLACEMENT_3D ( 'NONE', #26652, #19589, #32244 ) ;
#22059=DIRECTION ( 'NONE',  ( -1.224646799147353207E-16, -1.349345573449484691E-32, 1.000000000000000000 ) ) ;
#22061=DIRECTION ( 'NONE',  ( -1.000000000000000000, 0.000000000000000000, 0.000000000000000000 ) ) ;
#22072=CIRCLE ( 'NONE', #11103, 12.50967055512594150 ) ;
#22076=AXIS2_PLACEMENT_3D ( 'NONE', #18111, #556, #22879 ) ;
#22079=VECTOR ( 'NONE', #6498, 1000.000000000000000 ) ;
#22081=CARTESIAN_POINT ( 'NONE',  ( 21.09992658989239089, 30.09164230456639544, 47.04930799450051637 ) ) ;
#22084=CIRCLE ( 'NONE', #12138, 0.1249999999999983763 ) ;
#22085=ORIENTED_EDGE ( 'NONE', *, *, #6487, .F. ) ;
#22095=DIRECTION ( 'NONE',  ( -1.000000000000000000, 0.000000000000000000, 0.000000000000000000 ) ) ;
#22098=VERTEX_POINT ( 'NONE', #20807 ) ;
#22099=DIRECTION ( 'NONE',  ( 1.000000000000000000, 0.000000000000000000, 0.000000000000000000 ) ) ;
#22103=CIRCLE ( 'NONE', #9547, 0.1250000000000001110 ) ;
#22106=DIRECTION ( 'NONE',  ( -1.000000000000000000, 0.000000000000000000, 0.000000000000000000 ) ) ;
#22109=DIRECTION ( 'NONE',  ( -1.000000000000000000, -1.101824276508909887E-16, 0.000000000000000000 ) ) ;
#22113=ORIENTED_EDGE ( 'NONE', *, *, #29460, .F. ) ;
#22116=CARTESIAN_POINT ( 'NONE',  ( 21.09992658989239089, 26.09164230456639899, 47.04930799450051637 ) ) ;
#22118=TOROIDAL_SURFACE ( 'NONE', #31637, 12.40141737965283930, 0.1250000000000007216 ) ;
#22123=ORIENTED_EDGE ( 'NONE', *, *, #10805, .T. ) ;
#22124=DIRECTION ( 'NONE',  ( -1.000000000000000000, 0.000000000000000000, 0.000000000000000000 ) ) ;
#22127=CIRCLE ( 'NONE', #21604, 12.36707279061065101 ) ;
#22128=VERTEX_POINT ( 'NONE', #28043 ) ;
#22136=CARTESIAN_POINT ( 'NONE',  ( 21.09992658989238734, 31.46183152705961561, 47.04930799450051637 ) ) ;
#22137=CARTESIAN_POINT ( 'NONE',  ( 21.09992658989239089, 27.46183152705960850, 47.04930799450051637 ) ) ;
#22139=VERTEX_POINT ( 'NONE', #30830 ) ;
#22140=EDGE_LOOP ( 'NONE', ( #28404, #18491, #12147, #30224 ) ) ;
#22144=DIRECTION ( 'NONE',  ( -1.000000000000000000, 0.000000000000000000, 0.000000000000000000 ) ) ;
#22157=CIRCLE ( 'NONE', #9590, 12.62506659569710266 ) ;
#22169=VERTEX_POINT ( 'NONE', #788 ) ;
#22172=FACE_OUTER_BOUND ( 'NONE', #25556, .T. ) ;
#22174=ORIENTED_EDGE ( 'NONE', *, *, #11980, .T. ) ;
#22175=CIRCLE ( 'NONE', #24812, 12.62506659569710443 ) ;
#22176=DIRECTION ( 'NONE',  ( -1.224646799147353207E-16, -1.349345573449484691E-32, 1.000000000000000000 ) ) ;
#22178=ADVANCED_FACE ( 'NONE', ( #8663 ), #24890, .T. ) ;
#22182=DIRECTION ( 'NONE',  ( -1.000000000000000000, 0.000000000000000000, 0.000000000000000000 ) ) ;
#22185=CIRCLE ( 'NONE', #24801, 12.62506659569710443 ) ;
#22186=AXIS2_PLACEMENT_3D ( 'NONE', #8009, #18007, #5544 ) ;
#22187=CYLINDRICAL_SURFACE ( 'NONE', #14443, 12.36707279061065101 ) ;
#22191=DIRECTION ( 'NONE',  ( -1.000000000000000000, 0.000000000000000000, 0.000000000000000000 ) ) ;
#22196=EDGE_CURVE ( 'NONE', #20369, #25423, #785, .T. ) ;
#22197=EDGE_CURVE ( 'NONE', #21385, #7469, #31707, .T. ) ;
#22198=ORIENTED_EDGE ( 'NONE', *, *, #28029, .T. ) ;
#22199=DIRECTION ( 'NONE',  ( -1.101824276508909887E-16, 1.000000000000000000, -0.000000000000000000 ) ) ;
#22201=DIRECTION ( 'NONE',  ( -1.000000000000000000, -1.101824276508909887E-16, 0.000000000000000000 ) ) ;
#22202=ORIENTED_EDGE ( 'NONE', *, *, #32119, .F. ) ;
#22203=EDGE_LOOP ( 'NONE', ( #12918, #29036, #4714, #5226 ) ) ;
#22206=DIRECTION ( 'NONE',  ( -1.224646799147353207E-16, -1.349345573449484691E-32, 1.000000000000000000 ) ) ;
#22209=CARTESIAN_POINT ( 'NONE',  ( 8.482002859293421793, 26.46664230456639899, 47.04930799450051637 ) ) ;
#22214=VERTEX_POINT ( 'NONE', #5717 ) ;
#22216=CYLINDRICAL_SURFACE ( 'NONE', #26082, 12.36707279061065101 ) ;
#22218=EDGE_CURVE ( 'NONE', #31343, #17323, #29033, .T. ) ;
#22226=ORIENTED_EDGE ( 'NONE', *, *, #2118, .F. ) ;
#22228=FACE_OUTER_BOUND ( 'NONE', #9257, .T. ) ;
#22229=CARTESIAN_POINT ( 'NONE',  ( 21.09992658989238734, 38.56284415653841791, 47.04930799450051637 ) ) ;
#22231=CARTESIAN_POINT ( 'NONE',  ( 33.50134396954521065, 29.84164230456639899, 47.04930799450051637 ) ) ;
#22235=CARTESIAN_POINT ( 'NONE',  ( 33.50134396954522487, 29.09164230456639899, 47.04930799450051637 ) ) ;
#22240=CARTESIAN_POINT ( 'NONE',  ( 8.698509210239576461, 31.34164230456639544, 47.04930799450051637 ) ) ;
#22254=VERTEX_POINT ( 'NONE', #16355 ) ;
#22258=DIRECTION ( 'NONE',  ( -1.000000000000000000, 0.000000000000000000, 0.000000000000000000 ) ) ;
#22259=CARTESIAN_POINT ( 'NONE',  ( 33.46699938050304013, 29.21183152705961206, 47.04930799450051637 ) ) ;
#22262=EDGE_LOOP ( 'NONE', ( #12134, #6551, #5159, #8990 ) ) ;
#22268=FACE_OUTER_BOUND ( 'NONE', #29064, .T. ) ;
#22269=CARTESIAN_POINT ( 'NONE',  ( 21.09992658989239089, 23.59164230456639544, 47.04930799450051637 ) ) ;
#22281=DIRECTION ( 'NONE',  ( -1.000000000000000000, -1.101824276508909887E-16, 0.000000000000000000 ) ) ;
#22283=ORIENTED_EDGE ( 'NONE', *, *, #6346, .T. ) ;
#22285=CIRCLE ( 'NONE', #11302, 0.1250000000000001110 ) ;
#22290=DIRECTION ( 'NONE',  ( -1.000000000000000000, -1.101824276508909764E-16, 0.000000000000000000 ) ) ;
#22292=ADVANCED_FACE ( 'NONE', ( #7001 ), #16997, .T. ) ;
#22293=EDGE_CURVE ( 'NONE', #27591, #21064, #1583, .T. ) ;
#22294=CIRCLE ( 'NONE', #13349, 12.52247886585643677 ) ;
#22296=VERTEX_POINT ( 'NONE', #13750 ) ;
#22299=AXIS2_PLACEMENT_3D ( 'NONE', #17756, #17265, #4804 ) ;
#22302=ORIENTED_EDGE ( 'NONE', *, *, #21152, .F. ) ;
#22309=ORIENTED_EDGE ( 'NONE', *, *, #18692, .F. ) ;
#22313=CARTESIAN_POINT ( 'NONE',  ( 21.09992658989238734, 32.59164230456639899, 47.04930799450051637 ) ) ;
#22314=DIRECTION ( 'NONE',  ( -1.000000000000000000, -1.101824276508909764E-16, 0.000000000000000000 ) ) ;
#22315=CARTESIAN_POINT ( 'NONE',  ( 21.09992658989238734, 38.56284415653841791, 47.04930799450051637 ) ) ;
#22316=CARTESIAN_POINT ( 'NONE',  ( 33.46699938050304013, 26.97145308207318948, 47.04930799450050927 ) ) ;
#22318=ORIENTED_EDGE ( 'NONE', *, *, #28617, .T. ) ;
#22319=ORIENTED_EDGE ( 'NONE', *, *, #30298, .T. ) ;
#22321=FACE_OUTER_BOUND ( 'NONE', #15835, .T. ) ;
#22323=ORIENTED_EDGE ( 'NONE', *, *, #7781, .F. ) ;
#22328=DIRECTION ( 'NONE',  ( -1.101824276508909887E-16, 1.000000000000000000, -0.000000000000000000 ) ) ;
#22341=AXIS2_PLACEMENT_3D ( 'NONE', #19323, #14419, #11461 ) ;
#22343=CARTESIAN_POINT ( 'NONE',  ( 21.09992658989238734, 31.71183152705962272, 47.04930799450051637 ) ) ;
#22344=DIRECTION ( 'NONE',  ( 1.000000000000000000, 0.000000000000000000, 0.000000000000000000 ) ) ;
#22348=CARTESIAN_POINT ( 'NONE',  ( 8.732853799281734553, 38.56284415653841791, 47.04930799450051637 ) ) ;
#22349=DIRECTION ( 'NONE',  ( -1.101824276508909887E-16, 1.000000000000000000, -0.000000000000000000 ) ) ;
#22366=DIRECTION ( 'NONE',  ( -1.000000000000000000, 0.000000000000000000, 0.000000000000000000 ) ) ;
#22367=CYLINDRICAL_SURFACE ( 'NONE', #27964, 12.62506659569710443 ) ;
#22368=DIRECTION ( 'NONE',  ( -1.000000000000000000, 0.000000000000000000, 0.000000000000000000 ) ) ;
#22371=DIRECTION ( 'NONE',  ( -1.000000000000000000, -1.101824276508909764E-16, 0.000000000000000000 ) ) ;
#22378=CARTESIAN_POINT ( 'NONE',  ( 21.09992658989238734, 30.84164230456639544, 47.04930799450051637 ) ) ;
#22380=ORIENTED_EDGE ( 'NONE', *, *, #4783, .F. ) ;
#22381=DIRECTION ( 'NONE',  ( -1.000000000000000000, 0.000000000000000000, 0.000000000000000000 ) ) ;
#22382=VERTEX_POINT ( 'NONE', #27024 ) ;
#22388=CIRCLE ( 'NONE', #10359, 0.1250000000000001110 ) ;
#22390=CARTESIAN_POINT ( 'NONE',  ( 21.09992658989239089, 29.59143805560861296, 47.04930799450051637 ) ) ;
#22394=DIRECTION ( 'NONE',  ( 1.000000000000000000, 0.000000000000000000, 0.000000000000000000 ) ) ;
#22395=DIRECTION ( 'NONE',  ( -1.101824276508909887E-16, 1.000000000000000000, -0.000000000000000000 ) ) ;
#22396=AXIS2_PLACEMENT_3D ( 'NONE', #5341, #25987, #8441 ) ;
#22402=ORIENTED_EDGE ( 'NONE', *, *, #32178, .F. ) ;
#22405=ORIENTED_EDGE ( 'NONE', *, *, #31832, .T. ) ;
#22407=CIRCLE ( 'NONE', #8854, 0.1250000000000001110 ) ;
#22409=DIRECTION ( 'NONE',  ( -1.000000000000000000, 0.000000000000000000, 0.000000000000000000 ) ) ;
#22410=ADVANCED_FACE ( 'NONE', ( #4699 ), #12503, .T. ) ;
#22412=VECTOR ( 'NONE', #228, 1000.000000000000000 ) ;
#22413=ORIENTED_EDGE ( 'NONE', *, *, #15719, .T. ) ;
#22421=DIRECTION ( 'NONE',  ( -1.101824276508909887E-16, 1.000000000000000000, -0.000000000000000000 ) ) ;
#22424=DIRECTION ( 'NONE',  ( -1.000000000000000000, 0.000000000000000000, 0.000000000000000000 ) ) ;
#22425=DIRECTION ( 'NONE',  ( -1.101824276508909887E-16, 1.000000000000000000, -0.000000000000000000 ) ) ;
#22434=DIRECTION ( 'NONE',  ( 1.000000000000000000, 0.000000000000000000, 0.000000000000000000 ) ) ;
#22435=AXIS2_PLACEMENT_3D ( 'NONE', #22708, #27477, #223 ) ;
#22445=EDGE_CURVE ( 'NONE', #25766, #28443, #23474, .T. ) ;
#22450=EDGE_CURVE ( 'NONE', #460, #7622, #1984, .T. ) ;
#22452=AXIS2_PLACEMENT_3D ( 'NONE', #21727, #14202, #6644 ) ;
#22458=CARTESIAN_POINT ( 'NONE',  ( 21.09992658989239089, 28.34184655352419213, 47.04930799450051637 ) ) ;
#22460=ORIENTED_EDGE ( 'NONE', *, *, #21358, .F. ) ;
#22469=FACE_OUTER_BOUND ( 'NONE', #7658, .T. ) ;
#22473=EDGE_LOOP ( 'NONE', ( #19840, #25035, #362, #18968 ) ) ;
#22474=DIRECTION ( 'NONE',  ( -1.000000000000000000, 0.000000000000000000, 0.000000000000000000 ) ) ;
#22475=CARTESIAN_POINT ( 'NONE',  ( 8.474859994195286461, 25.59143805560860940, 47.04930799450051637 ) ) ;
#22476=EDGE_CURVE ( 'NONE', #19469, #9081, #7771, .T. ) ;
#22480=ORIENTED_EDGE ( 'NONE', *, *, #13470, .F. ) ;
#22483=AXIS2_PLACEMENT_3D ( 'NONE', #792, #16199, #15560 ) ;
#22490=AXIS2_PLACEMENT_3D ( 'NONE', #15582, #5099, #25599 ) ;
#22495=ORIENTED_EDGE ( 'NONE', *, *, #3021, .T. ) ;
#22497=FACE_OUTER_BOUND ( 'NONE', #21663, .T. ) ;
#22500=CARTESIAN_POINT ( 'NONE',  ( 21.09992658989239089, 26.72145308207318948, 47.04930799450051637 ) ) ;
#22502=AXIS2_PLACEMENT_3D ( 'NONE', #6467, #28474, #23702 ) ;
#22511=ORIENTED_EDGE ( 'NONE', *, *, #14170, .T. ) ;
#22512=ORIENTED_EDGE ( 'NONE', *, *, #10439, .F. ) ;
#22513=DIRECTION ( 'NONE',  ( -1.101824276508909887E-16, 1.000000000000000000, -0.000000000000000000 ) ) ;
#22515=LINE ( 'NONE', #25478, #8806 ) ;
#22516=CIRCLE ( 'NONE', #1032, 12.62506659569710443 ) ;
#22528=CIRCLE ( 'NONE', #19906, 0.1250000000000001110 ) ;
#22532=CARTESIAN_POINT ( 'NONE',  ( 21.09992658989238734, 38.56284415653841791, 47.04930799450051637 ) ) ;
#22535=TOROIDAL_SURFACE ( 'NONE', #19912, 12.40141737965288726, 0.1250000000000003331 ) ;
#22536=VERTEX_POINT ( 'NONE', #903 ) ;
#22537=CARTESIAN_POINT ( 'NONE',  ( 33.50134396954518934, 31.84164230456639544, 47.04930799450051637 ) ) ;
#22539=ORIENTED_EDGE ( 'NONE', *, *, #11433, .T. ) ;
#22540=CARTESIAN_POINT ( 'NONE',  ( 21.09992658989238734, 32.09184655352418503, 47.04930799450051637 ) ) ;
#22542=AXIS2_PLACEMENT_3D ( 'NONE', #4544, #2736, #25058 ) ;
#22545=DIRECTION ( 'NONE',  ( 1.000000000000000000, 0.000000000000000000, 0.000000000000000000 ) ) ;
#22546=EDGE_LOOP ( 'NONE', ( #7648, #24806, #2340, #22511 ) ) ;
#22547=DIRECTION ( 'NONE',  ( -1.101824276508909887E-16, 1.000000000000000000, -0.000000000000000000 ) ) ;
#22554=DIRECTION ( 'NONE',  ( -1.000000000000000000, 0.000000000000000000, 0.000000000000000000 ) ) ;
#22558=DIRECTION ( 'NONE',  ( -1.000000000000000000, 0.000000000000000000, 0.000000000000000000 ) ) ;
#22559=CARTESIAN_POINT ( 'NONE',  ( 8.482002859293432451, 27.46664230456639899, 47.04930799450051637 ) ) ;
#22561=CARTESIAN_POINT ( 'NONE',  ( 21.09992658989239089, 27.71183152705960850, 47.04930799450051637 ) ) ;
#22562=ADVANCED_FACE ( 'NONE', ( #15366 ), #20325, .T. ) ;
#22569=VECTOR ( 'NONE', #14940, 1000.000000000000000 ) ;
#22570=ORIENTED_EDGE ( 'NONE', *, *, #28461, .T. ) ;
#22572=EDGE_CURVE ( 'NONE', #21015, #414, #10394, .T. ) ;
#22574=AXIS2_PLACEMENT_3D ( 'NONE', #18049, #22813, #27910 ) ;
#22575=AXIS2_PLACEMENT_3D ( 'NONE', #19114, #16821, #9283 ) ;
#22581=ORIENTED_EDGE ( 'NONE', *, *, #27468, .T. ) ;
#22583=DIRECTION ( 'NONE',  ( -1.101824276508909887E-16, 1.000000000000000000, -0.000000000000000000 ) ) ;
#22584=DIRECTION ( 'NONE',  ( -1.101824276508909887E-16, 1.000000000000000000, -0.000000000000000000 ) ) ;
#22586=DIRECTION ( 'NONE',  ( -1.224646799147353207E-16, -1.349345573449484691E-32, 1.000000000000000000 ) ) ;
#22588=DIRECTION ( 'NONE',  ( -1.101824276508909887E-16, 1.000000000000000000, -0.000000000000000000 ) ) ;
#22597=ORIENTED_EDGE ( 'NONE', *, *, #13837, .T. ) ;
#22598=CARTESIAN_POINT ( 'NONE',  ( 21.09992658989238734, 38.56284415653841791, 47.04930799450051637 ) ) ;
#22602=CARTESIAN_POINT ( 'NONE',  ( 21.09992658989238734, 31.84184655352418503, 47.04930799450051637 ) ) ;
#22606=VERTEX_POINT ( 'NONE', #8148 ) ;
#22607=CARTESIAN_POINT ( 'NONE',  ( 21.09992658989239089, 25.84164230456639899, 47.04930799450051637 ) ) ;
#22610=TOROIDAL_SURFACE ( 'NONE', #22055, 12.61792373059891048, 0.1250000000000026368 ) ;
#22614=ORIENTED_EDGE ( 'NONE', *, *, #671, .T. ) ;
#22616=EDGE_CURVE ( 'NONE', #8103, #29193, #15682, .T. ) ;
#22621=ORIENTED_EDGE ( 'NONE', *, *, #1114, .F. ) ;
#22623=AXIS2_PLACEMENT_3D ( 'NONE', #22598, #24908, #2424 ) ;
#22624=EDGE_CURVE ( 'NONE', #31962, #18298, #31351, .T. ) ;
#22625=ORIENTED_EDGE ( 'NONE', *, *, #10423, .F. ) ;
#22632=EDGE_LOOP ( 'NONE', ( #21255, #31936, #9460, #10220 ) ) ;
#22633=DIRECTION ( 'NONE',  ( -1.101824276508909887E-16, 1.000000000000000000, -0.000000000000000000 ) ) ;
#22635=VERTEX_POINT ( 'NONE', #16805 ) ;
#22638=CARTESIAN_POINT ( 'NONE',  ( 8.474859994195281132, 30.84143805560860585, 47.04930799450051637 ) ) ;
#22644=EDGE_LOOP ( 'NONE', ( #5140, #23559, #8849, #7778 ) ) ;
#22646=CARTESIAN_POINT ( 'NONE',  ( 21.09992658989239089, 27.22145308207318593, 47.04930799450051637 ) ) ;
#22647=CARTESIAN_POINT ( 'NONE',  ( 8.474859994195282908, 38.56284415653841791, 47.04930799450051637 ) ) ;
#22648=DIRECTION ( 'NONE',  ( -1.101824276508909887E-16, 1.000000000000000000, -0.000000000000000000 ) ) ;
#22649=ORIENTED_EDGE ( 'NONE', *, *, #3070, .T. ) ;
#22662=EDGE_CURVE ( 'NONE', #7469, #4474, #10958, .T. ) ;
#22663=AXIS2_PLACEMENT_3D ( 'NONE', #17135, #12071, #17306 ) ;
#22664=DIRECTION ( 'NONE',  ( -1.000000000000000000, 0.000000000000000000, 0.000000000000000000 ) ) ;
#22668=VERTEX_POINT ( 'NONE', #18935 ) ;
#22670=DIRECTION ( 'NONE',  ( -1.000000000000000000, -1.101824276508909887E-16, 0.000000000000000000 ) ) ;
#22671=EDGE_CURVE ( 'NONE', #19672, #6679, #6746, .T. ) ;
#22673=ADVANCED_FACE ( 'NONE', ( #26657 ), #25095, .T. ) ;
#22686=EDGE_LOOP ( 'NONE', ( #15770, #28836, #25978, #17930 ) ) ;
#22688=DIRECTION ( 'NONE',  ( -1.000000000000000000, -1.101824276508909764E-16, 0.000000000000000000 ) ) ;
#22689=DIRECTION ( 'NONE',  ( -1.000000000000000000, 0.000000000000000000, 0.000000000000000000 ) ) ;
#22697=ORIENTED_EDGE ( 'NONE', *, *, #12275, .F. ) ;
#22698=ORIENTED_EDGE ( 'NONE', *, *, #27759, .F. ) ;
#22702=CYLINDRICAL_SURFACE ( 'NONE', #16956, 12.36707279061065279 ) ;
#22703=CARTESIAN_POINT ( 'NONE',  ( 21.09992658989239089, 24.34164230456639544, 47.04930799450051637 ) ) ;
#22706=VECTOR ( 'NONE', #7009, 1000.000000000000000 ) ;
#22707=ADVANCED_FACE ( 'NONE', ( #31755 ), #5702, .T. ) ;
#22708=CARTESIAN_POINT ( 'NONE',  ( 21.09992658989238734, 38.56284415653841791, 47.04930799450051637 ) ) ;
#22711=AXIS2_PLACEMENT_3D ( 'NONE', #9943, #25038, #2549 ) ;
#22713=DIRECTION ( 'NONE',  ( -1.101824276508909887E-16, 1.000000000000000000, -0.000000000000000000 ) ) ;
#22715=EDGE_CURVE ( 'NONE', #22032, #29832, #28237, .T. ) ;
#22718=ORIENTED_EDGE ( 'NONE', *, *, #11980, .F. ) ;
#22720=DIRECTION ( 'NONE',  ( -1.000000000000000000, -1.101824276508909887E-16, 0.000000000000000000 ) ) ;
#22722=CARTESIAN_POINT ( 'NONE',  ( 8.474859994195286461, 24.34184655352419213, 47.04930799450051637 ) ) ;
#22723=ORIENTED_EDGE ( 'NONE', *, *, #29500, .F. ) ;
#22725=DIRECTION ( 'NONE',  ( -1.101824276508909887E-16, 1.000000000000000000, -0.000000000000000000 ) ) ;
#22726=CARTESIAN_POINT ( 'NONE',  ( 21.09992658989239089, 28.59164230456639544, 47.04930799450051637 ) ) ;
#22730=ORIENTED_EDGE ( 'NONE', *, *, #26901, .F. ) ;
#22731=CARTESIAN_POINT ( 'NONE',  ( 21.09992658989239089, 24.34184655352419213, 47.04930799450051637 ) ) ;
#22739=AXIS2_PLACEMENT_3D ( 'NONE', #14674, #17612, #15158 ) ;
#22743=CIRCLE ( 'NONE', #5546, 0.1249999999999966416 ) ;
#22744=DIRECTION ( 'NONE',  ( -1.000000000000000000, 0.000000000000000000, 0.000000000000000000 ) ) ;
#22750=LINE ( 'NONE', #7167, #6794 ) ;
#22751=EDGE_CURVE ( 'NONE', #13336, #8460, #25604, .T. ) ;
#22767=CARTESIAN_POINT ( 'NONE',  ( 21.09992658989238734, 38.56284415653841791, 47.04930799450051637 ) ) ;
#22776=AXIS2_PLACEMENT_3D ( 'NONE', #16289, #13840, #9393 ) ;
#22779=ORIENTED_EDGE ( 'NONE', *, *, #16604, .F. ) ;
#22785=AXIS2_PLACEMENT_3D ( 'NONE', #30072, #4790, #22670 ) ;
#22787=EDGE_CURVE ( 'NONE', #16102, #21972, #16683, .T. ) ;
#22795=VERTEX_POINT ( 'NONE', #26989 ) ;
#22801=AXIS2_PLACEMENT_3D ( 'NONE', #21478, #19506, #14593 ) ;
#22803=DIRECTION ( 'NONE',  ( -1.000000000000000000, 0.000000000000000000, 0.000000000000000000 ) ) ;
#22807=EDGE_LOOP ( 'NONE', ( #20071, #27217, #17174, #10499 ) ) ;
#22813=DIRECTION ( 'NONE',  ( -1.101824276508909887E-16, 1.000000000000000000, -0.000000000000000000 ) ) ;
#22816=AXIS2_PLACEMENT_3D ( 'NONE', #2927, #12959, #10494 ) ;
#22826=AXIS2_PLACEMENT_3D ( 'NONE', #3607, #13631, #21480 ) ;
#22827=ORIENTED_EDGE ( 'NONE', *, *, #26223, .T. ) ;
#22841=ORIENTED_EDGE ( 'NONE', *, *, #19376, .T. ) ;
#22842=DIRECTION ( 'NONE',  ( -1.101824276508909887E-16, 1.000000000000000000, -0.000000000000000000 ) ) ;
#22845=FACE_OUTER_BOUND ( 'NONE', #6957, .T. ) ;
#22847=CARTESIAN_POINT ( 'NONE',  ( 21.09992658989239089, 25.09164230456639899, 47.04930799450051637 ) ) ;
#22853=ORIENTED_EDGE ( 'NONE', *, *, #3070, .F. ) ;
#22854=ORIENTED_EDGE ( 'NONE', *, *, #531, .F. ) ;
#22855=CARTESIAN_POINT ( 'NONE',  ( 21.09992658989239089, 25.09164230456639899, 47.04930799450051637 ) ) ;
#22860=FACE_OUTER_BOUND ( 'NONE', #14437, .T. ) ;
#22865=EDGE_CURVE ( 'NONE', #19678, #6679, #8823, .T. ) ;
#22867=CIRCLE ( 'NONE', #26003, 0.1250000000000001110 ) ;
#22868=VERTEX_POINT ( 'NONE', #6083 ) ;
#22871=EDGE_CURVE ( 'NONE', #1121, #5504, #30334, .T. ) ;
#22872=AXIS2_PLACEMENT_3D ( 'NONE', #4502, #9432, #16962 ) ;
#22879=DIRECTION ( 'NONE',  ( -1.000000000000000000, -1.101824276508909764E-16, 0.000000000000000000 ) ) ;
#22889=CARTESIAN_POINT ( 'NONE',  ( 33.71785032049134401, 27.96664230456639899, 47.04930799450051637 ) ) ;
#22894=VECTOR ( 'NONE', #3752, 1000.000000000000000 ) ;
#22898=EDGE_LOOP ( 'NONE', ( #1250, #28924, #1249, #14854 ) ) ;
#22899=FACE_OUTER_BOUND ( 'NONE', #28225, .T. ) ;
#22901=EDGE_CURVE ( 'NONE', #10687, #30925, #8326, .T. ) ;
#22902=AXIS2_PLACEMENT_3D ( 'NONE', #22703, #32337, #4923 ) ;
#22905=CARTESIAN_POINT ( 'NONE',  ( 8.732853799281734553, 38.56284415653841791, 47.04930799450051637 ) ) ;
#22912=DIRECTION ( 'NONE',  ( -1.000000000000000000, 0.000000000000000000, 0.000000000000000000 ) ) ;
#22913=ORIENTED_EDGE ( 'NONE', *, *, #9794, .T. ) ;
#22915=DIRECTION ( 'NONE',  ( -1.000000000000000000, 0.000000000000000000, 0.000000000000000000 ) ) ;
#22917=DIRECTION ( 'NONE',  ( -1.101824276508909887E-16, 1.000000000000000000, -0.000000000000000000 ) ) ;
#22922=DIRECTION ( 'NONE',  ( -1.101824276508909887E-16, 1.000000000000000000, -0.000000000000000000 ) ) ;
#22924=CARTESIAN_POINT ( 'NONE',  ( 21.09992658989239089, 25.34164230456639899, 47.04930799450051637 ) ) ;
#22925=DIRECTION ( 'NONE',  ( 0.000000000000000000, -0.000000000000000000, -1.000000000000000000 ) ) ;
#22932=DIRECTION ( 'NONE',  ( -1.101824276508909887E-16, 1.000000000000000000, -0.000000000000000000 ) ) ;
#22934=EDGE_CURVE ( 'NONE', #30065, #3912, #21916, .T. ) ;
#22937=AXIS2_PLACEMENT_3D ( 'NONE', #9079, #14010, #31408 ) ;
#22938=CIRCLE ( 'NONE', #31852, 12.27641737965281798 ) ;
#22953=DIRECTION ( 'NONE',  ( -1.000000000000000000, -1.101824276508909764E-16, 0.000000000000000000 ) ) ;
#22954=AXIS2_PLACEMENT_3D ( 'NONE', #27941, #5301, #25151 ) ;
#22955=AXIS2_PLACEMENT_3D ( 'NONE', #26239, #11795, #31173 ) ;
#22957=CARTESIAN_POINT ( 'NONE',  ( 21.09992658989238734, 38.56284415653841791, 47.04930799450051637 ) ) ;
#22959=ORIENTED_EDGE ( 'NONE', *, *, #3807, .T. ) ;
#22960=DIRECTION ( 'NONE',  ( 1.000000000000000000, 0.000000000000000000, 0.000000000000000000 ) ) ;
#22961=CYLINDRICAL_SURFACE ( 'NONE', #28240, 12.36707279061065101 ) ;
#22963=CARTESIAN_POINT ( 'NONE',  ( 21.09992658989239089, 29.71664230456640254, 47.04930799450051637 ) ) ;
#22965=ORIENTED_EDGE ( 'NONE', *, *, #1214, .T. ) ;
#22966=CARTESIAN_POINT ( 'NONE',  ( 33.46699938050303302, 38.56284415653841791, 47.04930799450051637 ) ) ;
#22970=ORIENTED_EDGE ( 'NONE', *, *, #5793, .F. ) ;
#22972=EDGE_CURVE ( 'NONE', #15854, #32455, #27065, .T. ) ;
#22976=AXIS2_PLACEMENT_3D ( 'NONE', #25289, #27586, #13143 ) ;
#22983=LINE ( 'NONE', #498, #25529 ) ;
#22986=ORIENTED_EDGE ( 'NONE', *, *, #18561, .F. ) ;
#22987=CARTESIAN_POINT ( 'NONE',  ( 21.09992658989238734, 31.59184655352418503, 47.04930799450051637 ) ) ;
#22990=EDGE_CURVE ( 'NONE', #29832, #22032, #1490, .T. ) ;
#22991=CARTESIAN_POINT ( 'NONE',  ( 21.09992658989239089, 26.21183152705960140, 47.04930799450051637 ) ) ;
#22996=DIRECTION ( 'NONE',  ( -1.000000000000000000, -1.101824276508909887E-16, 0.000000000000000000 ) ) ;
#22997=DIRECTION ( 'NONE',  ( -1.101824276508909887E-16, 1.000000000000000000, -0.000000000000000000 ) ) ;
#23001=ORIENTED_EDGE ( 'NONE', *, *, #18885, .F. ) ;
#23002=ADVANCED_FACE ( 'NONE', ( #4577 ), #21968, .F. ) ;
#23005=AXIS2_PLACEMENT_3D ( 'NONE', #17810, #5666, #15671 ) ;
#23012=ORIENTED_EDGE ( 'NONE', *, *, #20155, .F. ) ;
#23013=ORIENTED_EDGE ( 'NONE', *, *, #14475, .F. ) ;
#23020=FACE_OUTER_BOUND ( 'NONE', #1264, .T. ) ;
#23022=AXIS2_PLACEMENT_3D ( 'NONE', #29167, #16521, #11772 ) ;
#23023=AXIS2_PLACEMENT_3D ( 'NONE', #6628, #13701, #1205 ) ;
#23026=DIRECTION ( 'NONE',  ( -1.224646799147353207E-16, -1.349345573449484691E-32, 1.000000000000000000 ) ) ;
#23028=AXIS2_PLACEMENT_3D ( 'NONE', #2188, #4979, #22201 ) ;
#23031=DIRECTION ( 'NONE',  ( 1.000000000000000000, 0.000000000000000000, 0.000000000000000000 ) ) ;
#23033=CYLINDRICAL_SURFACE ( 'NONE', #7857, 12.62506659569710266 ) ;
#23038=CIRCLE ( 'NONE', #1545, 12.27641737965287838 ) ;
#23044=CARTESIAN_POINT ( 'NONE',  ( 21.09992658989239089, 25.71183152705960140, 47.04930799450051637 ) ) ;
#23048=DIRECTION ( 'NONE',  ( -1.000000000000000000, 0.000000000000000000, 0.000000000000000000 ) ) ;
#23050=CARTESIAN_POINT ( 'NONE',  ( 8.698509210239501854, 23.59164230456639544, 47.04930799450051637 ) ) ;
#23051=DIRECTION ( 'NONE',  ( -1.000000000000000000, 0.000000000000000000, 0.000000000000000000 ) ) ;
#23057=ORIENTED_EDGE ( 'NONE', *, *, #13760, .T. ) ;
#23058=ADVANCED_FACE ( 'NONE', ( #4423 ), #16185, .T. ) ;
#23063=VECTOR ( 'NONE', #11786, 1000.000000000000000 ) ;
#23067=CARTESIAN_POINT ( 'NONE',  ( 33.46699938050304013, 29.72145308207318237, 47.04930799450050927 ) ) ;
#23072=VERTEX_POINT ( 'NONE', #16562 ) ;
#23074=EDGE_LOOP ( 'NONE', ( #16081, #22718, #23272, #15922 ) ) ;
#23080=DIRECTION ( 'NONE',  ( -1.101824276508909887E-16, 1.000000000000000000, -0.000000000000000000 ) ) ;
#23085=VERTEX_POINT ( 'NONE', #4752 ) ;
#23088=AXIS2_PLACEMENT_3D ( 'NONE', #10618, #21965, #4420 ) ;
#23092=EDGE_CURVE ( 'NONE', #414, #21015, #32457, .T. ) ;
#23097=ORIENTED_EDGE ( 'NONE', *, *, #7038, .T. ) ;
#23098=DIRECTION ( 'NONE',  ( -1.000000000000000000, 0.000000000000000000, 0.000000000000000000 ) ) ;
#23101=ORIENTED_EDGE ( 'NONE', *, *, #13951, .F. ) ;
#23106=CIRCLE ( 'NONE', #31508, 0.1250000000000001110 ) ;
#23107=AXIS2_PLACEMENT_3D ( 'NONE', #22924, #442, #9980 ) ;
#23108=EDGE_LOOP ( 'NONE', ( #12785, #27149, #25888, #24667 ) ) ;
#23109=AXIS2_PLACEMENT_3D ( 'NONE', #20210, #7429, #10536 ) ;
#23114=EDGE_CURVE ( 'NONE', #14267, #5457, #17376, .T. ) ;
#23115=ORIENTED_EDGE ( 'NONE', *, *, #4854, .T. ) ;
#23118=FACE_OUTER_BOUND ( 'NONE', #7500, .T. ) ;
#23126=DIRECTION ( 'NONE',  ( -1.224646799147353207E-16, -1.349345573449484691E-32, 1.000000000000000000 ) ) ;
#23133=ORIENTED_EDGE ( 'NONE', *, *, #17571, .F. ) ;
#23134=CARTESIAN_POINT ( 'NONE',  ( 33.50134396954527460, 24.34164230456639544, 47.04930799450051637 ) ) ;
#23137=CARTESIAN_POINT ( 'NONE',  ( 33.37634396954526039, 25.59164230456639899, 47.04930799450051637 ) ) ;
#23139=ORIENTED_EDGE ( 'NONE', *, *, #7160, .T. ) ;
#23140=STYLED_ITEM('',(#32522),#11688);
#23141=DIRECTION ( 'NONE',  ( -1.101824276508909887E-16, 1.000000000000000000, -0.000000000000000000 ) ) ;
#23143=AXIS2_PLACEMENT_3D ( 'NONE', #28982, #3707, #14217 ) ;
#23144=DIRECTION ( 'NONE',  ( -1.101824276508909887E-16, 1.000000000000000000, -0.000000000000000000 ) ) ;
#23147=ORIENTED_EDGE ( 'NONE', *, *, #29579, .F. ) ;
#23150=CARTESIAN_POINT ( 'NONE',  ( 21.09992658989239089, 25.84164230456639899, 47.04930799450051637 ) ) ;
#23151=CARTESIAN_POINT ( 'NONE',  ( 8.823509210239588896, 32.59164230456639899, 47.04930799450051637 ) ) ;
#23159=EDGE_CURVE ( 'NONE', #9936, #19822, #30890, .T. ) ;
#23163=ADVANCED_FACE ( 'NONE', ( #27722 ), #1006, .T. ) ;
#23165=CARTESIAN_POINT ( 'NONE',  ( 21.09992658989239089, 26.47145308207318593, 47.04930799450051637 ) ) ;
#23171=ORIENTED_EDGE ( 'NONE', *, *, #3134, .F. ) ;
#23173=AXIS2_PLACEMENT_3D ( 'NONE', #23729, #1084, #8787 ) ;
#23178=DIRECTION ( 'NONE',  ( 1.000000000000000000, 0.000000000000000000, 0.000000000000000000 ) ) ;
#23185=TOROIDAL_SURFACE ( 'NONE', #30527, 12.40141737965287128, 0.1249999999999993477 ) ;
#23189=DIRECTION ( 'NONE',  ( -1.101824276508909887E-16, 1.000000000000000000, -0.000000000000000000 ) ) ;
#23191=CARTESIAN_POINT ( 'NONE',  ( 33.50134396954526750, 25.09164230456639899, 47.04930799450051637 ) ) ;
#23193=AXIS2_PLACEMENT_3D ( 'NONE', #31528, #19028, #29057 ) ;
#23197=DIRECTION ( 'NONE',  ( -1.101824276508909887E-16, 1.000000000000000000, -0.000000000000000000 ) ) ;
#23203=EDGE_CURVE ( 'NONE', #10661, #14676, #29309, .T. ) ;
#23209=ORIENTED_EDGE ( 'NONE', *, *, #22972, .T. ) ;
#23217=CARTESIAN_POINT ( 'NONE',  ( 33.72499318558949710, 28.09143805560861296, 47.04930799450051637 ) ) ;
#23219=EDGE_LOOP ( 'NONE', ( #7672, #23427, #16567, #21275 ) ) ;
#23220=DIRECTION ( 'NONE',  ( -1.101824276508909887E-16, 1.000000000000000000, -0.000000000000000000 ) ) ;
#23221=FACE_OUTER_BOUND ( 'NONE', #7793, .T. ) ;
#23225=EDGE_LOOP ( 'NONE', ( #26012, #21407, #16127, #1548 ) ) ;
#23231=AXIS2_PLACEMENT_3D ( 'NONE', #19908, #30259, #19739 ) ;
#23234=EDGE_CURVE ( 'NONE', #30824, #29832, #15143, .T. ) ;
#23235=DIRECTION ( 'NONE',  ( -1.000000000000000000, 0.000000000000000000, 0.000000000000000000 ) ) ;
#23246=DIRECTION ( 'NONE',  ( 1.000000000000000000, 0.000000000000000000, 0.000000000000000000 ) ) ;
#23247=EDGE_CURVE ( 'NONE', #22296, #4270, #25633, .T. ) ;
#23248=ORIENTED_EDGE ( 'NONE', *, *, #2155, .F. ) ;
#23249=DIRECTION ( 'NONE',  ( 1.000000000000000000, 0.000000000000000000, 0.000000000000000000 ) ) ;
#23258=CIRCLE ( 'NONE', #9099, 0.1250000000000001110 ) ;
#23272=ORIENTED_EDGE ( 'NONE', *, *, #17331, .T. ) ;
#23275=ADVANCED_FACE ( 'NONE', ( #18975 ), #8982, .T. ) ;
#23278=ORIENTED_EDGE ( 'NONE', *, *, #23814, .F. ) ;
#23280=ORIENTED_EDGE ( 'NONE', *, *, #9157, .F. ) ;
#23281=DIRECTION ( 'NONE',  ( -1.000000000000000000, 0.000000000000000000, 0.000000000000000000 ) ) ;
#23295=AXIS2_PLACEMENT_3D ( 'NONE', #15528, #22586, #107 ) ;
#23297=CARTESIAN_POINT ( 'NONE',  ( 21.09992658989239089, 24.34143805560860940, 47.04930799450051637 ) ) ;
#23298=AXIS2_PLACEMENT_3D ( 'NONE', #28454, #8739, #3655 ) ;
#23299=DIRECTION ( 'NONE',  ( -1.000000000000000000, -1.101824276508910010E-16, 0.000000000000000000 ) ) ;
#23301=CARTESIAN_POINT ( 'NONE',  ( 8.732853799281738105, 23.96183152705959785, 47.04930799450051637 ) ) ;
#23304=EDGE_LOOP ( 'NONE', ( #27362, #13554, #25013, #13471 ) ) ;
#23305=DIRECTION ( 'NONE',  ( -1.101824276508909887E-16, 1.000000000000000000, -0.000000000000000000 ) ) ;
#23309=EDGE_CURVE ( 'NONE', #20897, #32154, #13070, .T. ) ;
#23311=EDGE_CURVE ( 'NONE', #20144, #15199, #15695, .T. ) ;
#23315=DIRECTION ( 'NONE',  ( 1.000000000000000000, 0.000000000000000000, 0.000000000000000000 ) ) ;
#23319=CIRCLE ( 'NONE', #18567, 12.62506659569710443 ) ;
#23328=CARTESIAN_POINT ( 'NONE',  ( 21.09992658989239089, 27.71664230456639899, 47.04930799450051637 ) ) ;
#23333=EDGE_LOOP ( 'NONE', ( #2032, #4990, #4447, #13704 ) ) ;
#23339=DIRECTION ( 'NONE',  ( -1.101824276508909887E-16, 1.000000000000000000, -0.000000000000000000 ) ) ;
#23341=EDGE_LOOP ( 'NONE', ( #23604, #16573, #1479, #30949 ) ) ;
#23345=AXIS2_PLACEMENT_3D ( 'NONE', #17474, #17956, #27493 ) ;
#23349=AXIS2_PLACEMENT_3D ( 'NONE', #27639, #20245, #7957 ) ;
#23351=EDGE_CURVE ( 'NONE', #893, #25766, #15190, .T. ) ;
#23354=DIRECTION ( 'NONE',  ( -1.224646799147353207E-16, -1.349345573449484691E-32, 1.000000000000000000 ) ) ;
#23357=DIRECTION ( 'NONE',  ( -1.000000000000000000, 0.000000000000000000, 0.000000000000000000 ) ) ;
#23360=CARTESIAN_POINT ( 'NONE',  ( 8.698509210239537381, 27.09164230456639899, 47.04930799450051637 ) ) ;
#23373=CIRCLE ( 'NONE', #29132, 12.36707279061065279 ) ;
#23377=DIRECTION ( 'NONE',  ( 0.000000000000000000, -0.000000000000000000, -1.000000000000000000 ) ) ;
#23382=DIRECTION ( 'NONE',  ( -1.101824276508909887E-16, 1.000000000000000000, -0.000000000000000000 ) ) ;
#23383=DIRECTION ( 'NONE',  ( -1.101824276508909887E-16, 1.000000000000000000, -0.000000000000000000 ) ) ;
#23384=EDGE_LOOP ( 'NONE', ( #20771, #1732, #9174, #27638 ) ) ;
#23385=CARTESIAN_POINT ( 'NONE',  ( 21.09992658989239089, 30.21664230456641675, 47.04930799450051637 ) ) ;
#23386=ORIENTED_EDGE ( 'NONE', *, *, #303, .T. ) ;
#23390=ADVANCED_FACE ( 'NONE', ( #13917 ), #16674, .T. ) ;
#23393=CIRCLE ( 'NONE', #26006, 12.62506659569710443 ) ;
#23401=CARTESIAN_POINT ( 'NONE',  ( 21.09992658989239089, 24.21664230456639899, 47.04930799450051637 ) ) ;
#23405=ORIENTED_EDGE ( 'NONE', *, *, #5116, .F. ) ;
#23413=DIRECTION ( 'NONE',  ( 0.000000000000000000, -0.000000000000000000, -1.000000000000000000 ) ) ;
#23415=CARTESIAN_POINT ( 'NONE',  ( 33.72499318558949710, 29.34143805560861296, 47.04930799450051637 ) ) ;
#23427=ORIENTED_EDGE ( 'NONE', *, *, #7757, .T. ) ;
#23432=ORIENTED_EDGE ( 'NONE', *, *, #8178, .F. ) ;
#23435=ORIENTED_EDGE ( 'NONE', *, *, #20480, .T. ) ;
#23439=EDGE_CURVE ( 'NONE', #30111, #12384, #22750, .T. ) ;
#23445=ADVANCED_FACE ( 'NONE', ( #19793 ), #1024, .T. ) ;
#23450=TOROIDAL_SURFACE ( 'NONE', #17685, 12.40141737965280555, 0.1250000000000006939 ) ;
#23451=CARTESIAN_POINT ( 'NONE',  ( 21.09992658989238734, 31.84164230456639544, 47.04930799450051637 ) ) ;
#23454=LINE ( 'NONE', #25914, #31284 ) ;
#23457=CIRCLE ( 'NONE', #24503, 12.62506659569710266 ) ;
#23458=FACE_OUTER_BOUND ( 'NONE', #20321, .T. ) ;
#23462=TOROIDAL_SURFACE ( 'NONE', #5631, 12.40141737965288904, 0.1249999999999998612 ) ;
#23470=CARTESIAN_POINT ( 'NONE',  ( 33.50134396954527460, 24.09164230456639544, 47.04930799450051637 ) ) ;
#23473=CARTESIAN_POINT ( 'NONE',  ( 21.09992658989239089, 24.09164230456639544, 47.04930799450051637 ) ) ;
#23474=CIRCLE ( 'NONE', #17704, 0.1250000000000001110 ) ;
#23475=ORIENTED_EDGE ( 'NONE', *, *, #4942, .T. ) ;
#23476=CARTESIAN_POINT ( 'NONE',  ( 21.09992658989239089, 26.59164230456639899, 47.04930799450051637 ) ) ;
#23479=CARTESIAN_POINT ( 'NONE',  ( 21.09992658989238734, 38.56284415653841791, 47.04930799450051637 ) ) ;
#23480=EDGE_CURVE ( 'NONE', #22795, #29858, #28791, .T. ) ;
#23484=ADVANCED_FACE ( 'NONE', ( #12596 ), #17332, .T. ) ;
#23485=CARTESIAN_POINT ( 'NONE',  ( 21.09992658989239089, 30.59184655352422411, 47.04930799450051637 ) ) ;
#23494=EDGE_CURVE ( 'NONE', #28828, #23854, #19879, .T. ) ;
#23504=AXIS2_PLACEMENT_3D ( 'NONE', #22987, #19431, #25137 ) ;
#23508=CIRCLE ( 'NONE', #27677, 12.27641737965284463 ) ;
#23509=VERTEX_POINT ( 'NONE', #16165 ) ;
#23515=EDGE_CURVE ( 'NONE', #7622, #24404, #5747, .T. ) ;
#23516=DIRECTION ( 'NONE',  ( -1.000000000000000000, -1.101824276508909887E-16, 0.000000000000000000 ) ) ;
#23517=AXIS2_PLACEMENT_3D ( 'NONE', #5075, #30190, #12636 ) ;
#23520=CYLINDRICAL_SURFACE ( 'NONE', #23298, 12.36707279061065101 ) ;
#23521=AXIS2_PLACEMENT_3D ( 'NONE', #2670, #17923, #13011 ) ;
#23523=CARTESIAN_POINT ( 'NONE',  ( 21.09992658989238734, 38.56284415653841791, 47.04930799450051637 ) ) ;
#23530=TOROIDAL_SURFACE ( 'NONE', #2025, 12.61792373059898864, 0.1249999999999962669 ) ;
#23544=CIRCLE ( 'NONE', #27216, 12.62506659569710266 ) ;
#23549=AXIS2_PLACEMENT_3D ( 'NONE', #1786, #17035, #21953 ) ;
#23552=ORIENTED_EDGE ( 'NONE', *, *, #11315, .F. ) ;
#23554=ORIENTED_EDGE ( 'NONE', *, *, #30815, .T. ) ;
#23555=DIRECTION ( 'NONE',  ( -1.101824276508909887E-16, 1.000000000000000000, -0.000000000000000000 ) ) ;
#23556=DIRECTION ( 'NONE',  ( -1.101824276508909887E-16, 1.000000000000000000, -0.000000000000000000 ) ) ;
#23557=CARTESIAN_POINT ( 'NONE',  ( 33.72499318558949000, 38.56284415653841791, 47.04930799450051637 ) ) ;
#23558=LINE ( 'NONE', #30644, #31512 ) ;
#23559=ORIENTED_EDGE ( 'NONE', *, *, #13788, .T. ) ;
#23561=ORIENTED_EDGE ( 'NONE', *, *, #7781, .T. ) ;
#23564=CIRCLE ( 'NONE', #14153, 0.1250000000000001110 ) ;
#23568=ADVANCED_FACE ( 'NONE', ( #3372 ), #20774, .T. ) ;
#23570=DIRECTION ( 'NONE',  ( -1.101824276508909887E-16, 1.000000000000000000, -0.000000000000000000 ) ) ;
#23571=ADVANCED_FACE ( 'NONE', ( #1075 ), #10452, .F. ) ;
#23576=CARTESIAN_POINT ( 'NONE',  ( 21.09992658989239089, 25.47145308207319303, 47.04930799450051637 ) ) ;
#23577=DIRECTION ( 'NONE',  ( -1.101824276508909887E-16, 1.000000000000000000, -0.000000000000000000 ) ) ;
#23578=EDGE_CURVE ( 'NONE', #28996, #26728, #5230, .T. ) ;
#23582=CIRCLE ( 'NONE', #5237, 0.1250000000000001110 ) ;
#23583=CARTESIAN_POINT ( 'NONE',  ( 21.09992658989239089, 28.59164230456639544, 47.04930799450051637 ) ) ;
#23586=ORIENTED_EDGE ( 'NONE', *, *, #30909, .T. ) ;
#23588=AXIS2_PLACEMENT_3D ( 'NONE', #14017, #8756, #24015 ) ;
#23590=ORIENTED_EDGE ( 'NONE', *, *, #27759, .T. ) ;
#23591=TOROIDAL_SURFACE ( 'NONE', #7329, 12.40141737965285529, 0.1250000000000000555 ) ;
#23594=EDGE_CURVE ( 'NONE', #20651, #22795, #21955, .T. ) ;
#23598=AXIS2_PLACEMENT_3D ( 'NONE', #27077, #24781, #14293 ) ;
#23599=FACE_OUTER_BOUND ( 'NONE', #15206, .T. ) ;
#23600=DIRECTION ( 'NONE',  ( -1.101824276508909887E-16, 1.000000000000000000, -0.000000000000000000 ) ) ;
#23604=ORIENTED_EDGE ( 'NONE', *, *, #7458, .F. ) ;
#23607=EDGE_LOOP ( 'NONE', ( #31049, #835, #16365, #8882 ) ) ;
#23612=EDGE_CURVE ( 'NONE', #32203, #22254, #20938, .T. ) ;
#23614=DIRECTION ( 'NONE',  ( -1.101824276508909887E-16, 1.000000000000000000, -0.000000000000000000 ) ) ;
#23620=CARTESIAN_POINT ( 'NONE',  ( 21.09992658989239089, 29.34164230456639899, 47.04930799450051637 ) ) ;
#23623=CYLINDRICAL_SURFACE ( 'NONE', #2513, 12.36707279061065101 ) ;
#23624=ORIENTED_EDGE ( 'NONE', *, *, #18727, .F. ) ;
#23627=TOROIDAL_SURFACE ( 'NONE', #3705, 12.61792373059859962, 0.1250000000000011380 ) ;
#23628=ORIENTED_EDGE ( 'NONE', *, *, #28051, .T. ) ;
#23630=CIRCLE ( 'NONE', #3194, 0.1250000000000001110 ) ;
#23632=EDGE_CURVE ( 'NONE', #26531, #22668, #8306, .T. ) ;
#23635=EDGE_CURVE ( 'NONE', #1229, #14267, #26167, .T. ) ;
#23636=DIRECTION ( 'NONE',  ( -1.101824276508909887E-16, 1.000000000000000000, -0.000000000000000000 ) ) ;
#23645=DIRECTION ( 'NONE',  ( -1.000000000000000000, -1.101824276508910010E-16, 0.000000000000000000 ) ) ;
#23648=CARTESIAN_POINT ( 'NONE',  ( 21.09992658989239089, 30.22145308207317527, 47.04930799450051637 ) ) ;
#23651=DIRECTION ( 'NONE',  ( -1.101824276508909887E-16, 1.000000000000000000, -0.000000000000000000 ) ) ;
#23653=ADVANCED_FACE ( 'NONE', ( #4017 ), #19437, .F. ) ;
#23657=VECTOR ( 'NONE', #12443, 1000.000000000000000 ) ;
#23658=LINE ( 'NONE', #8399, #31381 ) ;
#23659=CARTESIAN_POINT ( 'NONE',  ( 33.46699938050303302, 38.56284415653841791, 47.04930799450051637 ) ) ;
#23660=ORIENTED_EDGE ( 'NONE', *, *, #27050, .F. ) ;
#23666=TOROIDAL_SURFACE ( 'NONE', #27872, 12.40141737965283930, 0.1250000000000007216 ) ;
#23669=EDGE_CURVE ( 'NONE', #3912, #14963, #5207, .T. ) ;
#23670=EDGE_LOOP ( 'NONE', ( #18761, #19526, #22123, #4248 ) ) ;
#23678=ADVANCED_FACE ( 'NONE', ( #4350 ), #19103, .T. ) ;
#23680=CARTESIAN_POINT ( 'NONE',  ( 21.09992658989239089, 25.59164230456639899, 47.04930799450051637 ) ) ;
#23682=CIRCLE ( 'NONE', #21043, 12.27641737965285174 ) ;
#23683=DIRECTION ( 'NONE',  ( 0.000000000000000000, -0.000000000000000000, -1.000000000000000000 ) ) ;
#23686=CARTESIAN_POINT ( 'NONE',  ( 8.732853799281738105, 27.21183152705960495, 47.04930799450051637 ) ) ;
#23687=DIRECTION ( 'NONE',  ( -1.101824276508909887E-16, 1.000000000000000000, -0.000000000000000000 ) ) ;
#23688=EDGE_CURVE ( 'NONE', #28361, #3559, #18807, .T. ) ;
#23690=LINE ( 'NONE', #3663, #12365 ) ;
#23692=DIRECTION ( 'NONE',  ( -1.101824276508909887E-16, 1.000000000000000000, -0.000000000000000000 ) ) ;
#23700=ORIENTED_EDGE ( 'NONE', *, *, #14276, .T. ) ;
#23702=DIRECTION ( 'NONE',  ( -1.000000000000000000, -1.101824276508909887E-16, 0.000000000000000000 ) ) ;
#23705=ORIENTED_EDGE ( 'NONE', *, *, #3551, .T. ) ;
#23708=ADVANCED_FACE ( 'NONE', ( #13881 ), #29859, .T. ) ;
#23713=AXIS2_PLACEMENT_3D ( 'NONE', #23772, #28876, #15312 ) ;
#23714=FACE_OUTER_BOUND ( 'NONE', #30115, .T. ) ;
#23716=CARTESIAN_POINT ( 'NONE',  ( 21.09992658989239089, 25.97145308207318593, 47.04930799450051637 ) ) ;
#23717=ORIENTED_EDGE ( 'NONE', *, *, #15128, .F. ) ;
#23720=DIRECTION ( 'NONE',  ( -1.101824276508909887E-16, 1.000000000000000000, -0.000000000000000000 ) ) ;
#23723=EDGE_LOOP ( 'NONE', ( #9746, #21912, #30710, #13285 ) ) ;
#23725=DIRECTION ( 'NONE',  ( -1.000000000000000000, -1.101824276508909887E-16, 0.000000000000000000 ) ) ;
#23727=DIRECTION ( 'NONE',  ( -1.101824276508909887E-16, 1.000000000000000000, -0.000000000000000000 ) ) ;
#23729=CARTESIAN_POINT ( 'NONE',  ( 33.50134396954518934, 31.84164230456639544, 47.04930799450051637 ) ) ;
#23730=DIRECTION ( 'NONE',  ( -1.101824276508909887E-16, 1.000000000000000000, -0.000000000000000000 ) ) ;
#23731=DIRECTION ( 'NONE',  ( -1.224646799147353207E-16, -1.349345573449484691E-32, 1.000000000000000000 ) ) ;
#23734=EDGE_LOOP ( 'NONE', ( #27025, #31974, #23435, #31801 ) ) ;
#23745=ADVANCED_FACE ( 'NONE', ( #14207 ), #8388, .T. ) ;
#23746=VECTOR ( 'NONE', #17674, 1000.000000000000000 ) ;
#23758=ORIENTED_EDGE ( 'NONE', *, *, #13279, .T. ) ;
#23759=ORIENTED_EDGE ( 'NONE', *, *, #81, .F. ) ;
#23764=CARTESIAN_POINT ( 'NONE',  ( 8.482002859293412911, 25.71664230456640254, 47.04930799450051637 ) ) ;
#23769=DIRECTION ( 'NONE',  ( -1.101824276508909887E-16, 1.000000000000000000, -0.000000000000000000 ) ) ;
#23772=CARTESIAN_POINT ( 'NONE',  ( 21.09992658989239089, 30.09164230456639544, 47.04930799450051637 ) ) ;
#23778=DIRECTION ( 'NONE',  ( -1.000000000000000000, 0.000000000000000000, 0.000000000000000000 ) ) ;
#23784=EDGE_CURVE ( 'NONE', #28525, #2007, #24102, .T. ) ;
#23787=ADVANCED_FACE ( 'NONE', ( #32415 ), #1055, .T. ) ;
#23795=DIRECTION ( 'NONE',  ( -1.000000000000000000, 0.000000000000000000, 0.000000000000000000 ) ) ;
#23802=FILL_AREA_STYLE ('',( #15783 ) ) ;
#23809=DIRECTION ( 'NONE',  ( -1.000000000000000000, -1.101824276508909887E-16, 0.000000000000000000 ) ) ;
#23810=DIRECTION ( 'NONE',  ( -1.000000000000000000, -1.101824276508909887E-16, 0.000000000000000000 ) ) ;
#23812=CARTESIAN_POINT ( 'NONE',  ( 21.09992658989239089, 29.59164230456639899, 47.04930799450051637 ) ) ;
#23814=EDGE_CURVE ( 'NONE', #25906, #231, #23564, .T. ) ;
#23815=ADVANCED_FACE ( 'NONE', ( #27485 ), #23591, .T. ) ;
#23816=DIRECTION ( 'NONE',  ( -1.101824276508909887E-16, 1.000000000000000000, -0.000000000000000000 ) ) ;
#23823=ORIENTED_EDGE ( 'NONE', *, *, #20448, .F. ) ;
#23826=CARTESIAN_POINT ( 'NONE',  ( 21.09992658989239089, 28.84164230456639544, 47.04930799450051637 ) ) ;
#23834=DIRECTION ( 'NONE',  ( -1.000000000000000000, -1.101824276508909887E-16, 0.000000000000000000 ) ) ;
#23844=VECTOR ( 'NONE', #4023, 1000.000000000000000 ) ;
#23845=CYLINDRICAL_SURFACE ( 'NONE', #5162, 12.62506659569710266 ) ;
#23853=DIRECTION ( 'NONE',  ( -1.101824276508909887E-16, 1.000000000000000000, -0.000000000000000000 ) ) ;
#23854=VERTEX_POINT ( 'NONE', #7634 ) ;
#23857=EDGE_CURVE ( 'NONE', #29931, #9420, #15720, .T. ) ;
#23859=DIRECTION ( 'NONE',  ( 1.000000000000000000, 0.000000000000000000, 0.000000000000000000 ) ) ;
#23861=EDGE_CURVE ( 'NONE', #25724, #26085, #9423, .T. ) ;
#23862=VERTEX_POINT ( 'NONE', #5165 ) ;
#23870=VECTOR ( 'NONE', #5490, 1000.000000000000000 ) ;
#23871=AXIS2_PLACEMENT_3D ( 'NONE', #12394, #5160, #22381 ) ;
#23874=DIRECTION ( 'NONE',  ( -1.101824276508909887E-16, 1.000000000000000000, -0.000000000000000000 ) ) ;
#23875=CIRCLE ( 'NONE', #8689, 0.1249999999999931721 ) ;
#23879=DIRECTION ( 'NONE',  ( -1.101824276508909887E-16, 1.000000000000000000, -0.000000000000000000 ) ) ;
#23885=CARTESIAN_POINT ( 'NONE',  ( 21.09992658989238734, 38.56284415653841791, 47.04930799450051637 ) ) ;
#23900=CIRCLE ( 'NONE', #15007, 0.1250000000000001110 ) ;
#23903=CARTESIAN_POINT ( 'NONE',  ( 21.09992658989239089, 25.59164230456639899, 47.04930799450051637 ) ) ;
#23904=ADVANCED_FACE ( 'NONE', ( #20248 ), #20427, .T. ) ;
#23911=CIRCLE ( 'NONE', #14515, 0.1250000000000001110 ) ;
#23912=EDGE_LOOP ( 'NONE', ( #1254, #29142, #1355, #13850 ) ) ;
#23921=ORIENTED_EDGE ( 'NONE', *, *, #21884, .T. ) ;
#23922=CARTESIAN_POINT ( 'NONE',  ( 33.71785032049132980, 29.46664230456640254, 47.04930799450051637 ) ) ;
#23932=FACE_OUTER_BOUND ( 'NONE', #24138, .T. ) ;
#23934=ADVANCED_FACE ( 'NONE', ( #29628 ), #19911, .T. ) ;
#23937=CARTESIAN_POINT ( 'NONE',  ( 8.732853799281738105, 26.21183152705960140, 47.04930799450051637 ) ) ;
#23940=CARTESIAN_POINT ( 'NONE',  ( 8.474859994195286461, 26.34184655352419213, 47.04930799450051637 ) ) ;
#23941=EDGE_LOOP ( 'NONE', ( #23624, #15918, #31012, #30517 ) ) ;
#23948=CARTESIAN_POINT ( 'NONE',  ( 21.09992658989238734, 32.21183152705962272, 47.04930799450051637 ) ) ;
#23952=CARTESIAN_POINT ( 'NONE',  ( 21.09992658989239089, 30.22145308207317527, 47.04930799450051637 ) ) ;
#23957=VERTEX_POINT ( 'NONE', #18426 ) ;
#23960=TOROIDAL_SURFACE ( 'NONE', #15079, 12.61792373059899397, 0.1249999999999959616 ) ;
#23963=ORIENTED_EDGE ( 'NONE', *, *, #21959, .F. ) ;
#23966=CYLINDRICAL_SURFACE ( 'NONE', #5705, 12.62506659569710266 ) ;
#23969=DIRECTION ( 'NONE',  ( -1.101824276508909887E-16, 1.000000000000000000, -0.000000000000000000 ) ) ;
#23971=EDGE_CURVE ( 'NONE', #27727, #18298, #6817, .T. ) ;
#23974=DIRECTION ( 'NONE',  ( -1.101824276508909887E-16, 1.000000000000000000, -0.000000000000000000 ) ) ;
#23979=CARTESIAN_POINT ( 'NONE',  ( 21.09992658989238734, 38.56284415653841791, 47.04930799450051637 ) ) ;
#23980=CIRCLE ( 'NONE', #13524, 12.62506659569710443 ) ;
#23982=ORIENTED_EDGE ( 'NONE', *, *, #11257, .T. ) ;
#23984=CYLINDRICAL_SURFACE ( 'NONE', #3856, 12.36707279061065101 ) ;
#23990=CARTESIAN_POINT ( 'NONE',  ( 33.46699938050304013, 23.96183152705959785, 47.04930799450051637 ) ) ;
#23992=ADVANCED_FACE ( 'NONE', ( #13520 ), #23033, .T. ) ;
#23994=DIRECTION ( 'NONE',  ( -1.101824276508909887E-16, 1.000000000000000000, -0.000000000000000000 ) ) ;
#23996=DIRECTION ( 'NONE',  ( -1.000000000000000000, 0.000000000000000000, 0.000000000000000000 ) ) ;
#24000=ORIENTED_EDGE ( 'NONE', *, *, #11266, .T. ) ;
#24002=AXIS2_PLACEMENT_3D ( 'NONE', #10684, #2946, #12977 ) ;
#24004=DIRECTION ( 'NONE',  ( -1.101824276508909887E-16, 1.000000000000000000, -0.000000000000000000 ) ) ;
#24007=DIRECTION ( 'NONE',  ( -1.101824276508909887E-16, 1.000000000000000000, -0.000000000000000000 ) ) ;
#24012=DIRECTION ( 'NONE',  ( -1.000000000000000000, 0.000000000000000000, 0.000000000000000000 ) ) ;
#24015=DIRECTION ( 'NONE',  ( -1.000000000000000000, -1.101824276508910010E-16, 0.000000000000000000 ) ) ;
#24018=DIRECTION ( 'NONE',  ( -1.000000000000000000, 0.000000000000000000, 0.000000000000000000 ) ) ;
#24026=AXIS2_PLACEMENT_3D ( 'NONE', #27911, #12980, #5100 ) ;
#24041=DIRECTION ( 'NONE',  ( -1.000000000000000000, 0.000000000000000000, 0.000000000000000000 ) ) ;
#24044=ORIENTED_EDGE ( 'NONE', *, *, #5227, .T. ) ;
#24047=DIRECTION ( 'NONE',  ( 1.000000000000000000, 0.000000000000000000, 0.000000000000000000 ) ) ;
#24049=DIRECTION ( 'NONE',  ( -1.101824276508909887E-16, 1.000000000000000000, -0.000000000000000000 ) ) ;
#24050=ORIENTED_EDGE ( 'NONE', *, *, #10247, .T. ) ;
#24051=CARTESIAN_POINT ( 'NONE',  ( 33.50134396954525329, 25.84164230456639899, 47.04930799450051637 ) ) ;
#24054=EDGE_CURVE ( 'NONE', #25102, #18493, #8897, .T. ) ;
#24063=AXIS2_PLACEMENT_3D ( 'NONE', #11470, #8846, #23778 ) ;
#24064=EDGE_CURVE ( 'NONE', #25197, #22536, #2108, .T. ) ;
#24068=AXIS2_PLACEMENT_3D ( 'NONE', #21222, #31259, #8757 ) ;
#24071=EDGE_CURVE ( 'NONE', #25102, #13965, #6284, .T. ) ;
#24076=ORIENTED_EDGE ( 'NONE', *, *, #31628, .T. ) ;
#24079=ORIENTED_EDGE ( 'NONE', *, *, #11852, .T. ) ;
#24082=VECTOR ( 'NONE', #26441, 1000.000000000000000 ) ;
#24085=DIRECTION ( 'NONE',  ( -1.000000000000000000, 0.000000000000000000, 0.000000000000000000 ) ) ;
#24092=CARTESIAN_POINT ( 'NONE',  ( 8.474859994195286461, 26.59143805560860940, 47.04930799450051637 ) ) ;
#24094=FACE_OUTER_BOUND ( 'NONE', #29557, .T. ) ;
#24097=EDGE_LOOP ( 'NONE', ( #7040, #14502, #13808, #528 ) ) ;
#24098=CARTESIAN_POINT ( 'NONE',  ( 33.72499318558949710, 24.84143805560860940, 47.04930799450051637 ) ) ;
#24100=DIRECTION ( 'NONE',  ( -1.101824276508909887E-16, 1.000000000000000000, -0.000000000000000000 ) ) ;
#24102=CIRCLE ( 'NONE', #505, 0.1250000000000001110 ) ;
#24112=DIRECTION ( 'NONE',  ( -1.101824276508909887E-16, 1.000000000000000000, -0.000000000000000000 ) ) ;
#24113=DIRECTION ( 'NONE',  ( -1.101824276508909887E-16, 1.000000000000000000, -0.000000000000000000 ) ) ;
#24116=ORIENTED_EDGE ( 'NONE', *, *, #31907, .F. ) ;
#24124=DIRECTION ( 'NONE',  ( -1.000000000000000000, 0.000000000000000000, 0.000000000000000000 ) ) ;
#24125=DIRECTION ( 'NONE',  ( 0.000000000000000000, -0.000000000000000000, -1.000000000000000000 ) ) ;
#24126=CARTESIAN_POINT ( 'NONE',  ( 21.09992658989239089, 25.46664230456640254, 47.04930799450051637 ) ) ;
#24129=VERTEX_POINT ( 'NONE', #21528 ) ;
#24131=AXIS2_PLACEMENT_3D ( 'NONE', #20583, #6129, #16129 ) ;
#24133=AXIS2_PLACEMENT_3D ( 'NONE', #16176, #16022, #28657 ) ;
#24138=EDGE_LOOP ( 'NONE', ( #8549, #32472, #12150, #9640 ) ) ;
#24141=DIRECTION ( 'NONE',  ( -1.000000000000000000, 0.000000000000000000, 0.000000000000000000 ) ) ;
#24143=CIRCLE ( 'NONE', #8430, 12.62506659569710443 ) ;
#24157=DIRECTION ( 'NONE',  ( -1.101824276508909887E-16, 1.000000000000000000, -0.000000000000000000 ) ) ;
#24158=AXIS2_PLACEMENT_3D ( 'NONE', #2895, #15689, #3213 ) ;
#24161=CARTESIAN_POINT ( 'NONE',  ( 33.71785032049133690, 28.71664230456639899, 47.04930799450051637 ) ) ;
#24162=LINE ( 'NONE', #21526, #14799 ) ;
#24171=CARTESIAN_POINT ( 'NONE',  ( 33.46699938050304013, 30.46183152705961561, 47.04930799450051637 ) ) ;
#24183=LINE ( 'NONE', #19086, #5720 ) ;
#24184=CIRCLE ( 'NONE', #27882, 12.27641737965284108 ) ;
#24189=VERTEX_POINT ( 'NONE', #16603 ) ;
#24193=EDGE_CURVE ( 'NONE', #13402, #21924, #13136, .T. ) ;
#24194=ADVANCED_FACE ( 'NONE', ( #13685 ), #16450, .F. ) ;
#24203=AXIS2_PLACEMENT_3D ( 'NONE', #15502, #5819, #28463 ) ;
#24207=CARTESIAN_POINT ( 'NONE',  ( 21.09992658989239089, 24.84164230456639544, 47.04930799450051637 ) ) ;
#24210=FACE_OUTER_BOUND ( 'NONE', #15525, .T. ) ;
#24211=CYLINDRICAL_SURFACE ( 'NONE', #3229, 12.62506659569710266 ) ;
#24212=FACE_OUTER_BOUND ( 'NONE', #23108, .T. ) ;
#24213=ORIENTED_EDGE ( 'NONE', *, *, #2803, .F. ) ;
#24217=LINE ( 'NONE', #31453, #5959 ) ;
#24228=EDGE_CURVE ( 'NONE', #16912, #31503, #18863, .T. ) ;
#24232=DIRECTION ( 'NONE',  ( -1.000000000000000000, 0.000000000000000000, 0.000000000000000000 ) ) ;
#24233=EDGE_CURVE ( 'NONE', #19067, #30753, #16247, .T. ) ;
#24237=DIRECTION ( 'NONE',  ( -1.000000000000000000, 0.000000000000000000, 0.000000000000000000 ) ) ;
#24242=CARTESIAN_POINT ( 'NONE',  ( 21.09992658989239089, 30.34184655352422411, 47.04930799450051637 ) ) ;
#24252=CIRCLE ( 'NONE', #15364, 0.1249999999999983763 ) ;
#24255=EDGE_CURVE ( 'NONE', #4827, #12851, #9467, .T. ) ;
#24257=CARTESIAN_POINT ( 'NONE',  ( 21.09992658989239089, 27.34143805560860940, 47.04930799450051637 ) ) ;
#24266=DIRECTION ( 'NONE',  ( -1.101824276508909887E-16, 1.000000000000000000, -0.000000000000000000 ) ) ;
#24274=AXIS2_PLACEMENT_3D ( 'NONE', #10918, #5663, #31103 ) ;
#24277=CARTESIAN_POINT ( 'NONE',  ( 33.72499318558949710, 24.09143805560860940, 47.04930799450051637 ) ) ;
#24279=DIRECTION ( 'NONE',  ( -1.000000000000000000, -1.101824276508910010E-16, 0.000000000000000000 ) ) ;
#24280=CARTESIAN_POINT ( 'NONE',  ( 21.09992658989238734, 38.56284415653841791, 47.04930799450051637 ) ) ;
#24291=CARTESIAN_POINT ( 'NONE',  ( 33.72499318558949000, 38.56284415653841791, 47.04930799450051637 ) ) ;
#24294=EDGE_LOOP ( 'NONE', ( #4538, #8001, #30509, #3478 ) ) ;
#24300=ORIENTED_EDGE ( 'NONE', *, *, #24255, .F. ) ;
#24301=CIRCLE ( 'NONE', #1241, 12.62506659569710266 ) ;
#24303=DIRECTION ( 'NONE',  ( -1.000000000000000000, 0.000000000000000000, 0.000000000000000000 ) ) ;
#24304=AXIS2_PLACEMENT_3D ( 'NONE', #2430, #12938, #29844 ) ;
#24305=ORIENTED_EDGE ( 'NONE', *, *, #17217, .F. ) ;
#24306=CARTESIAN_POINT ( 'NONE',  ( 8.823509210239528500, 26.34164230456639899, 47.04930799450051637 ) ) ;
#24308=EDGE_CURVE ( 'NONE', #22635, #22214, #29379, .T. ) ;
#24311=VERTEX_POINT ( 'NONE', #14653 ) ;
#24312=DIRECTION ( 'NONE',  ( -1.101824276508909887E-16, 1.000000000000000000, -0.000000000000000000 ) ) ;
#24320=FACE_OUTER_BOUND ( 'NONE', #13034, .T. ) ;
#24321=CARTESIAN_POINT ( 'NONE',  ( 21.09992658989238734, 31.84143805560860940, 47.04930799450051637 ) ) ;
#24324=EDGE_LOOP ( 'NONE', ( #6204, #8063, #18177, #17646 ) ) ;
#24325=DIRECTION ( 'NONE',  ( -1.101824276508909887E-16, 1.000000000000000000, -0.000000000000000000 ) ) ;
#24326=FACE_OUTER_BOUND ( 'NONE', #16320, .T. ) ;
#24334=ORIENTED_EDGE ( 'NONE', *, *, #14233, .T. ) ;
#24337=TOROIDAL_SURFACE ( 'NONE', #10200, 12.61792373059899219, 0.1249999999999961003 ) ;
#24347=DIRECTION ( 'NONE',  ( 0.000000000000000000, -0.000000000000000000, -1.000000000000000000 ) ) ;
#24348=EDGE_LOOP ( 'NONE', ( #5689, #9766, #32406, #2277 ) ) ;
#24355=DIRECTION ( 'NONE',  ( -1.101824276508909887E-16, 1.000000000000000000, -0.000000000000000000 ) ) ;
#24357=DIRECTION ( 'NONE',  ( -1.000000000000000000, -1.101824276508909887E-16, 0.000000000000000000 ) ) ;
#24362=ORIENTED_EDGE ( 'NONE', *, *, #9597, .T. ) ;
#24369=DIRECTION ( 'NONE',  ( -1.000000000000000000, 0.000000000000000000, 0.000000000000000000 ) ) ;
#24372=CARTESIAN_POINT ( 'NONE',  ( 8.474859994195286461, 29.34184655352418858, 47.04930799450051637 ) ) ;
#24373=DIRECTION ( 'NONE',  ( 1.000000000000000000, 0.000000000000000000, 0.000000000000000000 ) ) ;
#24379=FACE_OUTER_BOUND ( 'NONE', #22807, .T. ) ;
#24380=ADVANCED_FACE ( 'NONE', ( #2004 ), #19721, .F. ) ;
#24385=ADVANCED_FACE ( 'NONE', ( #12023 ), #20444, .T. ) ;
#24386=AXIS2_PLACEMENT_3D ( 'NONE', #21780, #21620, #24085 ) ;
#24387=ADVANCED_FACE ( 'NONE', ( #22016 ), #27266, .T. ) ;
#24388=AXIS2_PLACEMENT_3D ( 'NONE', #12070, #6491, #4021 ) ;
#24389=AXIS2_PLACEMENT_3D ( 'NONE', #29588, #29750, #13887 ) ;
#24394=ORIENTED_EDGE ( 'NONE', *, *, #12784, .T. ) ;
#24401=ADVANCED_FACE ( 'NONE', ( #5608 ), #8941, .T. ) ;
#24404=VERTEX_POINT ( 'NONE', #20366 ) ;
#24405=VECTOR ( 'NONE', #16128, 1000.000000000000000 ) ;
#24408=ORIENTED_EDGE ( 'NONE', *, *, #16659, .F. ) ;
#24413=DIRECTION ( 'NONE',  ( -1.000000000000000000, 0.000000000000000000, 0.000000000000000000 ) ) ;
#24416=LINE ( 'NONE', #19158, #18005 ) ;
#24418=FACE_OUTER_BOUND ( 'NONE', #30790, .T. ) ;
#24426=FACE_OUTER_BOUND ( 'NONE', #17327, .T. ) ;
#24427=DIRECTION ( 'NONE',  ( -1.101824276508909887E-16, 1.000000000000000000, -0.000000000000000000 ) ) ;
#24429=ORIENTED_EDGE ( 'NONE', *, *, #23114, .T. ) ;
#24435=DIRECTION ( 'NONE',  ( 0.000000000000000000, -0.000000000000000000, -1.000000000000000000 ) ) ;
#24436=ADVANCED_FACE ( 'NONE', ( #13167 ), #7391, .T. ) ;
#24437=AXIS2_PLACEMENT_3D ( 'NONE', #26172, #748, #28328 ) ;
#24446=EDGE_CURVE ( 'NONE', #21006, #18493, #30988, .T. ) ;
#24447=EDGE_LOOP ( 'NONE', ( #29954, #22539, #19105, #11472 ) ) ;
#24454=VERTEX_POINT ( 'NONE', #8237 ) ;
#24456=VECTOR ( 'NONE', #8686, 1000.000000000000000 ) ;
#24464=CARTESIAN_POINT ( 'NONE',  ( 21.09992658989238734, 31.46664230456641675, 47.04930799450051637 ) ) ;
#24465=CYLINDRICAL_SURFACE ( 'NONE', #450, 12.62506659569710266 ) ;
#24468=DIRECTION ( 'NONE',  ( -1.000000000000000000, 0.000000000000000000, 0.000000000000000000 ) ) ;
#24470=EDGE_CURVE ( 'NONE', #19118, #20658, #28873, .T. ) ;
#24473=CARTESIAN_POINT ( 'NONE',  ( 21.09992658989239089, 26.22145308207318593, 47.04930799450051637 ) ) ;
#24483=CARTESIAN_POINT ( 'NONE',  ( 21.09992658989239089, 30.09184655352422411, 47.04930799450051637 ) ) ;
#24485=FACE_OUTER_BOUND ( 'NONE', #20883, .T. ) ;
#24488=CARTESIAN_POINT ( 'NONE',  ( 21.09992658989238734, 38.56284415653841791, 47.04930799450051637 ) ) ;
#24496=DIRECTION ( 'NONE',  ( -1.000000000000000000, 0.000000000000000000, 0.000000000000000000 ) ) ;
#24499=ORIENTED_EDGE ( 'NONE', *, *, #31062, .T. ) ;
#24500=ORIENTED_EDGE ( 'NONE', *, *, #19704, .T. ) ;
#24503=AXIS2_PLACEMENT_3D ( 'NONE', #22029, #29759, #31736 ) ;
#24506=ORIENTED_EDGE ( 'NONE', *, *, #32176, .F. ) ;
#24508=VECTOR ( 'NONE', #397, 1000.000000000000000 ) ;
#24510=AXIS2_PLACEMENT_3D ( 'NONE', #8939, #21081, #8769 ) ;
#24515=DIRECTION ( 'NONE',  ( -1.000000000000000000, -1.101824276508909764E-16, 0.000000000000000000 ) ) ;
#24526=AXIS2_PLACEMENT_3D ( 'NONE', #14985, #12701, #22689 ) ;
#24527=CARTESIAN_POINT ( 'NONE',  ( 21.09992658989238734, 38.56284415653841791, 47.04930799450051637 ) ) ;
#24531=FACE_OUTER_BOUND ( 'NONE', #11723, .T. ) ;
#24536=CARTESIAN_POINT ( 'NONE',  ( 33.50134396954526039, 25.59164230456639899, 47.04930799450051637 ) ) ;
#24538=VERTEX_POINT ( 'NONE', #26550 ) ;
#24541=ORIENTED_EDGE ( 'NONE', *, *, #17860, .T. ) ;
#24546=AXIS2_PLACEMENT_3D ( 'NONE', #12547, #20081, #19914 ) ;
#24549=ORIENTED_EDGE ( 'NONE', *, *, #19402, .F. ) ;
#24551=AXIS2_PLACEMENT_3D ( 'NONE', #3955, #18552, #13977 ) ;
#24557=EDGE_CURVE ( 'NONE', #7034, #26728, #18988, .T. ) ;
#24562=FACE_OUTER_BOUND ( 'NONE', #27191, .T. ) ;
#24563=EDGE_CURVE ( 'NONE', #2124, #21917, #6872, .T. ) ;
#24565=VERTEX_POINT ( 'NONE', #11024 ) ;
#24567=ORIENTED_EDGE ( 'NONE', *, *, #20338, .F. ) ;
#24572=CARTESIAN_POINT ( 'NONE',  ( 8.474859994195286461, 27.09143805560860940, 47.04930799450051637 ) ) ;
#24573=AXIS2_PLACEMENT_3D ( 'NONE', #22209, #10081, #29771 ) ;
#24576=CARTESIAN_POINT ( 'NONE',  ( 21.09992658989239089, 25.71664230456640254, 47.04930799450051637 ) ) ;
#24582=DIRECTION ( 'NONE',  ( -1.101824276508909887E-16, 1.000000000000000000, -0.000000000000000000 ) ) ;
#24587=DIRECTION ( 'NONE',  ( -1.224646799147353207E-16, -1.349345573449484691E-32, 1.000000000000000000 ) ) ;
#24590=CARTESIAN_POINT ( 'NONE',  ( 21.09992658989239089, 24.47145308207319303, 47.04930799450051637 ) ) ;
#24594=CIRCLE ( 'NONE', #16197, 12.36707279061065101 ) ;
#24596=ORIENTED_EDGE ( 'NONE', *, *, #2072, .T. ) ;
#24601=CIRCLE ( 'NONE', #9429, 0.1250000000000001110 ) ;
#24602=EDGE_LOOP ( 'NONE', ( #4353, #12616, #19277, #22723 ) ) ;
#24604=DIRECTION ( 'NONE',  ( -1.101824276508909887E-16, 1.000000000000000000, -0.000000000000000000 ) ) ;
#24605=ADVANCED_FACE ( 'NONE', ( #9487 ), #12096, .T. ) ;
#24612=DIRECTION ( 'NONE',  ( -1.101824276508909887E-16, 1.000000000000000000, -0.000000000000000000 ) ) ;
#24613=ORIENTED_EDGE ( 'NONE', *, *, #5423, .F. ) ;
#24616=CYLINDRICAL_SURFACE ( 'NONE', #19503, 12.62506659569710443 ) ;
#24617=CARTESIAN_POINT ( 'NONE',  ( 21.09992658989239089, 26.84164230456639899, 47.04930799450051637 ) ) ;
#24621=VERTEX_POINT ( 'NONE', #24572 ) ;
#24623=AXIS2_PLACEMENT_3D ( 'NONE', #17301, #12231, #9769 ) ;
#24630=CARTESIAN_POINT ( 'NONE',  ( 8.474859994195286461, 25.09143805560860940, 47.04930799450051637 ) ) ;
#24632=AXIS2_PLACEMENT_3D ( 'NONE', #27039, #27533, #9975 ) ;
#24636=VECTOR ( 'NONE', #25390, 1000.000000000000000 ) ;
#24640=ORIENTED_EDGE ( 'NONE', *, *, #4828, .T. ) ;
#24641=ORIENTED_EDGE ( 'NONE', *, *, #9950, .T. ) ;
#24643=CARTESIAN_POINT ( 'NONE',  ( 21.09992658989238734, 32.46183152705962272, 47.04930799450051637 ) ) ;
#24647=CARTESIAN_POINT ( 'NONE',  ( 33.50134396954521776, 29.34164230456639899, 47.04930799450051637 ) ) ;
#24648=DIRECTION ( 'NONE',  ( -1.000000000000000000, 0.000000000000000000, 0.000000000000000000 ) ) ;
#24650=CIRCLE ( 'NONE', #19915, 12.36707279061065101 ) ;
#24651=CIRCLE ( 'NONE', #20460, 0.1250000000000001110 ) ;
#24652=DIRECTION ( 'NONE',  ( -1.101824276508909887E-16, 1.000000000000000000, -0.000000000000000000 ) ) ;
#24658=LINE ( 'NONE', #8784, #23844 ) ;
#24660=AXIS2_PLACEMENT_3D ( 'NONE', #16977, #32100, #4358 ) ;
#24661=ORIENTED_EDGE ( 'NONE', *, *, #25244, .F. ) ;
#24667=ORIENTED_EDGE ( 'NONE', *, *, #3851, .F. ) ;
#24671=EDGE_CURVE ( 'NONE', #2915, #8103, #32031, .T. ) ;
#24676=AXIS2_PLACEMENT_3D ( 'NONE', #18391, #13487, #10544 ) ;
#24678=EDGE_CURVE ( 'NONE', #21924, #22032, #4245, .T. ) ;
#24679=DIRECTION ( 'NONE',  ( -1.224646799147353207E-16, -1.349345573449484691E-32, 1.000000000000000000 ) ) ;
#24684=CIRCLE ( 'NONE', #9469, 0.1250000000000001110 ) ;
#24687=VECTOR ( 'NONE', #15907, 1000.000000000000000 ) ;
#24692=DIRECTION ( 'NONE',  ( -1.000000000000000000, 0.000000000000000000, 0.000000000000000000 ) ) ;
#24693=CARTESIAN_POINT ( 'NONE',  ( 21.09992658989238734, 38.56284415653841791, 47.04930799450051637 ) ) ;
#24694=EDGE_CURVE ( 'NONE', #24565, #15433, #6318, .T. ) ;
#24696=ORIENTED_EDGE ( 'NONE', *, *, #24193, .T. ) ;
#24705=DIRECTION ( 'NONE',  ( -1.101824276508909887E-16, 1.000000000000000000, -0.000000000000000000 ) ) ;
#24711=ADVANCED_FACE ( 'NONE', ( #27368 ), #19432, .T. ) ;
#24715=AXIS2_PLACEMENT_3D ( 'NONE', #12926, #8478, #22915 ) ;
#24717=ADVANCED_FACE ( 'NONE', ( #5210 ), #15256, .T. ) ;
#24718=DIRECTION ( 'NONE',  ( -1.101824276508909887E-16, 1.000000000000000000, -0.000000000000000000 ) ) ;
#24719=ORIENTED_EDGE ( 'NONE', *, *, #18801, .T. ) ;
#24720=ORIENTED_EDGE ( 'NONE', *, *, #6236, .T. ) ;
#24721=CIRCLE ( 'NONE', #17372, 0.1250000000000001110 ) ;
#24723=ORIENTED_EDGE ( 'NONE', *, *, #22572, .T. ) ;
#24727=CARTESIAN_POINT ( 'NONE',  ( 21.09992658989239089, 23.59164230456639544, 47.04930799450051637 ) ) ;
#24728=ORIENTED_EDGE ( 'NONE', *, *, #21782, .F. ) ;
#24730=DIRECTION ( 'NONE',  ( 1.000000000000000000, 0.000000000000000000, 0.000000000000000000 ) ) ;
#24731=DIRECTION ( 'NONE',  ( -1.224646799147353207E-16, -1.349345573449484691E-32, 1.000000000000000000 ) ) ;
#24732=CARTESIAN_POINT ( 'NONE',  ( 21.09992658989238734, 38.56284415653841791, 47.04930799450051637 ) ) ;
#24734=CARTESIAN_POINT ( 'NONE',  ( 21.09992658989239089, 30.21183152705961561, 47.04930799450051637 ) ) ;
#24735=ORIENTED_EDGE ( 'NONE', *, *, #31083, .F. ) ;
#24736=CARTESIAN_POINT ( 'NONE',  ( 33.46699938050304013, 32.46183152705962272, 47.04930799450051637 ) ) ;
#24737=ORIENTED_EDGE ( 'NONE', *, *, #7821, .F. ) ;
#24741=ORIENTED_EDGE ( 'NONE', *, *, #7160, .F. ) ;
#24742=DIRECTION ( 'NONE',  ( -1.101824276508909887E-16, 1.000000000000000000, -0.000000000000000000 ) ) ;
#24743=DIRECTION ( 'NONE',  ( -1.224646799147353207E-16, -1.349345573449484691E-32, 1.000000000000000000 ) ) ;
#24755=CYLINDRICAL_SURFACE ( 'NONE', #29490, 12.36707279061065101 ) ;
#24757=VERTEX_POINT ( 'NONE', #9810 ) ;
#24768=CIRCLE ( 'NONE', #662, 0.1250000000000001110 ) ;
#24772=CARTESIAN_POINT ( 'NONE',  ( 8.732853799281738105, 24.46183152705960140, 47.04930799450051637 ) ) ;
#24773=DIRECTION ( 'NONE',  ( -1.000000000000000000, 0.000000000000000000, 0.000000000000000000 ) ) ;
#24775=ORIENTED_EDGE ( 'NONE', *, *, #860, .T. ) ;
#24776=ORIENTED_EDGE ( 'NONE', *, *, #15663, .T. ) ;
#24780=CARTESIAN_POINT ( 'NONE',  ( 33.46699938050304013, 27.96183152705961206, 47.04930799450051637 ) ) ;
#24781=DIRECTION ( 'NONE',  ( -1.101824276508909887E-16, 1.000000000000000000, -0.000000000000000000 ) ) ;
#24784=EDGE_LOOP ( 'NONE', ( #43, #22319, #21550, #10558 ) ) ;
#24785=EDGE_LOOP ( 'NONE', ( #11779, #10316, #28378, #22614 ) ) ;
#24786=DIRECTION ( 'NONE',  ( -1.101824276508909887E-16, 1.000000000000000000, -0.000000000000000000 ) ) ;
#24789=CIRCLE ( 'NONE', #21640, 0.1250000000000018319 ) ;
#24795=DIRECTION ( 'NONE',  ( -1.101824276508909887E-16, 1.000000000000000000, -0.000000000000000000 ) ) ;
#24801=AXIS2_PLACEMENT_3D ( 'NONE', #9419, #32069, #21545 ) ;
#24805=EDGE_CURVE ( 'NONE', #27840, #2021, #24850, .T. ) ;
#24806=ORIENTED_EDGE ( 'NONE', *, *, #23612, .F. ) ;
#24807=ORIENTED_EDGE ( 'NONE', *, *, #19552, .F. ) ;
#24811=ORIENTED_EDGE ( 'NONE', *, *, #1405, .F. ) ;
#24812=AXIS2_PLACEMENT_3D ( 'NONE', #22602, #12119, #12281 ) ;
#24814=AXIS2_PLACEMENT_3D ( 'NONE', #15372, #15529, #5685 ) ;
#24818=CARTESIAN_POINT ( 'NONE',  ( 21.09992658989239089, 30.21664230456641675, 47.04930799450051637 ) ) ;
#24820=AXIS2_PLACEMENT_3D ( 'NONE', #3019, #30934, #13532 ) ;
#24821=FACE_OUTER_BOUND ( 'NONE', #11750, .T. ) ;
#24823=AXIS2_PLACEMENT_3D ( 'NONE', #3966, #11510, #9052 ) ;
#24830=CARTESIAN_POINT ( 'NONE',  ( 33.46699938050304013, 28.46183152705961206, 47.04930799450051637 ) ) ;
#24835=EDGE_LOOP ( 'NONE', ( #15750, #21039, #24079, #21402 ) ) ;
#24838=CARTESIAN_POINT ( 'NONE',  ( 21.09992658989238734, 31.09164230456639544, 47.04930799450051637 ) ) ;
#24840=ORIENTED_EDGE ( 'NONE', *, *, #15444, .F. ) ;
#24843=CARTESIAN_POINT ( 'NONE',  ( 21.09992658989239089, 28.72145308207318237, 47.04930799450051637 ) ) ;
#24848=ADVANCED_FACE ( 'NONE', ( #14517 ), #10565, .T. ) ;
#24850=LINE ( 'NONE', #21560, #21533 ) ;
#24854=DIRECTION ( 'NONE',  ( -1.000000000000000000, 0.000000000000000000, 0.000000000000000000 ) ) ;
#24858=ORIENTED_EDGE ( 'NONE', *, *, #9950, .F. ) ;
#24859=CARTESIAN_POINT ( 'NONE',  ( 21.09992658989239089, 29.59164230456639899, 47.04930799450051637 ) ) ;
#24861=FACE_OUTER_BOUND ( 'NONE', #19659, .T. ) ;
#24862=AXIS2_PLACEMENT_3D ( 'NONE', #24483, #23556, #28495 ) ;
#24864=ORIENTED_EDGE ( 'NONE', *, *, #11243, .T. ) ;
#24867=DIRECTION ( 'NONE',  ( -1.101824276508909887E-16, 1.000000000000000000, -0.000000000000000000 ) ) ;
#24868=CARTESIAN_POINT ( 'NONE',  ( 33.72499318558949710, 25.59184655352419213, 47.04930799450051637 ) ) ;
#24870=ADVANCED_FACE ( 'NONE', ( #12053 ), #22610, .T. ) ;
#24875=ORIENTED_EDGE ( 'NONE', *, *, #26937, .F. ) ;
#24877=CARTESIAN_POINT ( 'NONE',  ( 21.09992658989239089, 26.34164230456639899, 47.04930799450051637 ) ) ;
#24879=CYLINDRICAL_SURFACE ( 'NONE', #28751, 12.36707279061065101 ) ;
#24881=DIRECTION ( 'NONE',  ( 1.000000000000000000, 0.000000000000000000, 0.000000000000000000 ) ) ;
#24886=CIRCLE ( 'NONE', #8654, 12.36707279061065101 ) ;
#24887=TOROIDAL_SURFACE ( 'NONE', #31190, 12.61792373059860495, 0.1250000000000008604 ) ;
#24888=AXIS2_PLACEMENT_3D ( 'NONE', #19306, #7339, #31798 ) ;
#24890=TOROIDAL_SURFACE ( 'NONE', #6548, 12.40141737965282509, 0.1249999999999980849 ) ;
#24894=ORIENTED_EDGE ( 'NONE', *, *, #387, .T. ) ;
#24900=CARTESIAN_POINT ( 'NONE',  ( 8.698509210239585343, 32.09164230456639899, 47.04930799450051637 ) ) ;
#24901=ORIENTED_EDGE ( 'NONE', *, *, #27161, .T. ) ;
#24902=DIRECTION ( 'NONE',  ( -1.101824276508909887E-16, 1.000000000000000000, -0.000000000000000000 ) ) ;
#24908=DIRECTION ( 'NONE',  ( -1.101824276508909887E-16, 1.000000000000000000, -0.000000000000000000 ) ) ;
#24912=DIRECTION ( 'NONE',  ( -1.000000000000000000, 0.000000000000000000, 0.000000000000000000 ) ) ;
#24915=CIRCLE ( 'NONE', #15485, 0.1250000000000001110 ) ;
#24922=AXIS2_PLACEMENT_3D ( 'NONE', #30448, #2859, #17795 ) ;
#24933=DIRECTION ( 'NONE',  ( -1.101824276508909887E-16, 1.000000000000000000, -0.000000000000000000 ) ) ;
#24939=DIRECTION ( 'NONE',  ( -1.000000000000000000, 0.000000000000000000, 0.000000000000000000 ) ) ;
#24945=ADVANCED_FACE ( 'NONE', ( #32212 ), #29952, .T. ) ;
#24949=DIRECTION ( 'NONE',  ( -1.101824276508909887E-16, 1.000000000000000000, -0.000000000000000000 ) ) ;
#24955=EDGE_LOOP ( 'NONE', ( #44, #21530, #15883, #3669 ) ) ;
#24965=ORIENTED_EDGE ( 'NONE', *, *, #14388, .T. ) ;
#24971=DIRECTION ( 'NONE',  ( -1.000000000000000000, 0.000000000000000000, 0.000000000000000000 ) ) ;
#24978=DIRECTION ( 'NONE',  ( -1.000000000000000000, 0.000000000000000000, 0.000000000000000000 ) ) ;
#24981=CARTESIAN_POINT ( 'NONE',  ( 21.09992658989238734, 38.56284415653841791, 47.04930799450051637 ) ) ;
#24982=ADVANCED_FACE ( 'NONE', ( #24485 ), #26791, .T. ) ;
#24985=DIRECTION ( 'NONE',  ( -1.000000000000000000, 0.000000000000000000, 0.000000000000000000 ) ) ;
#24988=ORIENTED_EDGE ( 'NONE', *, *, #11198, .F. ) ;
#24990=CARTESIAN_POINT ( 'NONE',  ( 33.37634396954526750, 24.84164230456639544, 47.04930799450051637 ) ) ;
#24994=TOROIDAL_SURFACE ( 'NONE', #22902, 12.40141737965288193, 0.1250000000000005829 ) ;
#24997=DIRECTION ( 'NONE',  ( 0.000000000000000000, -0.000000000000000000, -1.000000000000000000 ) ) ;
#24998=CARTESIAN_POINT ( 'NONE',  ( 33.72499318558949710, 31.84143805560860940, 47.04930799450051637 ) ) ;
#25007=EDGE_LOOP ( 'NONE', ( #22570, #16941, #11340, #19351 ) ) ;
#25009=ORIENTED_EDGE ( 'NONE', *, *, #3799, .T. ) ;
#25010=DIRECTION ( 'NONE',  ( 1.000000000000000000, 0.000000000000000000, 0.000000000000000000 ) ) ;
#25012=TOROIDAL_SURFACE ( 'NONE', #10873, 12.61792373059899219, 0.1249999999999961003 ) ;
#25013=ORIENTED_EDGE ( 'NONE', *, *, #32119, .T. ) ;
#25015=EDGE_LOOP ( 'NONE', ( #6529, #3633, #15672, #14880 ) ) ;
#25018=CYLINDRICAL_SURFACE ( 'NONE', #19377, 12.62506659569710443 ) ;
#25019=DIRECTION ( 'NONE',  ( -1.101824276508909887E-16, 1.000000000000000000, -0.000000000000000000 ) ) ;
#25021=DIRECTION ( 'NONE',  ( -1.000000000000000000, 0.000000000000000000, 0.000000000000000000 ) ) ;
#25023=DIRECTION ( 'NONE',  ( -1.101824276508909887E-16, 1.000000000000000000, -0.000000000000000000 ) ) ;
#25025=DIRECTION ( 'NONE',  ( -1.000000000000000000, 0.000000000000000000, 0.000000000000000000 ) ) ;
#25026=VECTOR ( 'NONE', #28114, 1000.000000000000000 ) ;
#25029=LINE ( 'NONE', #28303, #24508 ) ;
#25034=AXIS2_PLACEMENT_3D ( 'NONE', #19071, #13376, #1361 ) ;
#25035=ORIENTED_EDGE ( 'NONE', *, *, #4334, .F. ) ;
#25037=CYLINDRICAL_SURFACE ( 'NONE', #14069, 12.62506659569710266 ) ;
#25038=DIRECTION ( 'NONE',  ( -1.101824276508909887E-16, 1.000000000000000000, -0.000000000000000000 ) ) ;
#25039=EDGE_LOOP ( 'NONE', ( #27097, #8241, #7962, #18532 ) ) ;
#25043=ADVANCED_FACE ( 'NONE', ( #24821 ), #30081, .T. ) ;
#25044=ORIENTED_EDGE ( 'NONE', *, *, #27158, .T. ) ;
#25046=VECTOR ( 'NONE', #10780, 1000.000000000000000 ) ;
#25048=AXIS2_PLACEMENT_3D ( 'NONE', #21923, #16518, #24232 ) ;
#25050=DIRECTION ( 'NONE',  ( -1.000000000000000000, -1.101824276508909887E-16, 0.000000000000000000 ) ) ;
#25051=EDGE_LOOP ( 'NONE', ( #22302, #16832, #4531, #22697 ) ) ;
#25058=DIRECTION ( 'NONE',  ( -1.000000000000000000, 0.000000000000000000, 0.000000000000000000 ) ) ;
#25059=EDGE_CURVE ( 'NONE', #30824, #21924, #3725, .T. ) ;
#25061=DIRECTION ( 'NONE',  ( -1.101824276508909887E-16, 1.000000000000000000, -0.000000000000000000 ) ) ;
#25064=CARTESIAN_POINT ( 'NONE',  ( 21.09992658989238734, 30.84164230456639544, 47.04930799450051637 ) ) ;
#25065=EDGE_LOOP ( 'NONE', ( #14911, #23705, #29866, #14137 ) ) ;
#25066=CYLINDRICAL_SURFACE ( 'NONE', #22623, 12.36707279061065101 ) ;
#25073=DIRECTION ( 'NONE',  ( -1.000000000000000000, 0.000000000000000000, 0.000000000000000000 ) ) ;
#25083=AXIS2_PLACEMENT_3D ( 'NONE', #9783, #17486, #19774 ) ;
#25086=DIRECTION ( 'NONE',  ( -1.101824276508909887E-16, 1.000000000000000000, -0.000000000000000000 ) ) ;
#25094=DIRECTION ( 'NONE',  ( -1.000000000000000000, -1.101824276508910010E-16, 0.000000000000000000 ) ) ;
#25095=TOROIDAL_SURFACE ( 'NONE', #5157, 12.40141737965279667, 0.1249999999999991951 ) ;
#25097=AXIS2_PLACEMENT_3D ( 'NONE', #25634, #13178, #10716 ) ;
#25102=VERTEX_POINT ( 'NONE', #8678 ) ;
#25104=DIRECTION ( 'NONE',  ( -1.101824276508909887E-16, 1.000000000000000000, -0.000000000000000000 ) ) ;
#25105=EDGE_LOOP ( 'NONE', ( #30223, #4201, #9549, #26459 ) ) ;
#25107=DIRECTION ( 'NONE',  ( -1.000000000000000000, 0.000000000000000000, 0.000000000000000000 ) ) ;
#25114=ORIENTED_EDGE ( 'NONE', *, *, #11352, .F. ) ;
#25116=DIRECTION ( 'NONE',  ( -1.000000000000000000, -1.101824276508909764E-16, 0.000000000000000000 ) ) ;
#25117=DIRECTION ( 'NONE',  ( -1.101824276508909887E-16, 1.000000000000000000, -0.000000000000000000 ) ) ;
#25123=DIRECTION ( 'NONE',  ( -1.101824276508909887E-16, 1.000000000000000000, -0.000000000000000000 ) ) ;
#25125=AXIS2_PLACEMENT_3D ( 'NONE', #23385, #30943, #10437 ) ;
#25126=ADVANCED_FACE ( 'NONE', ( #29176 ), #23666, .T. ) ;
#25127=CARTESIAN_POINT ( 'NONE',  ( 21.09992658989238734, 32.59164230456639899, 47.04930799450051637 ) ) ;
#25134=CARTESIAN_POINT ( 'NONE',  ( 33.71785032049137953, 24.71664230456639899, 47.04930799450051637 ) ) ;
#25137=DIRECTION ( 'NONE',  ( -1.000000000000000000, 0.000000000000000000, 0.000000000000000000 ) ) ;
#25140=AXIS2_PLACEMENT_3D ( 'NONE', #27829, #3024, #10604 ) ;
#25142=DIRECTION ( 'NONE',  ( -1.000000000000000000, 0.000000000000000000, 0.000000000000000000 ) ) ;
#25148=EDGE_LOOP ( 'NONE', ( #18573, #3061, #26056, #29332 ) ) ;
#25151=DIRECTION ( 'NONE',  ( -1.000000000000000000, 0.000000000000000000, 0.000000000000000000 ) ) ;
#25152=DIRECTION ( 'NONE',  ( -1.101824276508909887E-16, 1.000000000000000000, -0.000000000000000000 ) ) ;
#25156=VERTEX_POINT ( 'NONE', #8991 ) ;
#25158=AXIS2_PLACEMENT_3D ( 'NONE', #30506, #18015, #5555 ) ;
#25168=CARTESIAN_POINT ( 'NONE',  ( 21.09992658989239089, 29.84164230456639899, 47.04930799450051637 ) ) ;
#25171=ORIENTED_EDGE ( 'NONE', *, *, #81, .T. ) ;
#25176=EDGE_LOOP ( 'NONE', ( #16519, #23921, #9321, #29117 ) ) ;
#25177=CIRCLE ( 'NONE', #13626, 12.62506659569710443 ) ;
#25178=DIRECTION ( 'NONE',  ( -1.000000000000000000, -1.101824276508909887E-16, 0.000000000000000000 ) ) ;
#25181=CIRCLE ( 'NONE', #13665, 12.62506659569710266 ) ;
#25182=ORIENTED_EDGE ( 'NONE', *, *, #17573, .F. ) ;
#25185=DIRECTION ( 'NONE',  ( -1.000000000000000000, 0.000000000000000000, 0.000000000000000000 ) ) ;
#25189=FACE_OUTER_BOUND ( 'NONE', #16060, .T. ) ;
#25193=AXIS2_PLACEMENT_3D ( 'NONE', #18737, #1679, #11702 ) ;
#25194=CARTESIAN_POINT ( 'NONE',  ( 33.46699938050304013, 31.46183152705961561, 47.04930799450051637 ) ) ;
#25195=CARTESIAN_POINT ( 'NONE',  ( 21.09992658989239089, 23.96664230456639899, 47.04930799450051637 ) ) ;
#25196=CARTESIAN_POINT ( 'NONE',  ( 33.72499318558949710, 29.09184655352418858, 47.04930799450051637 ) ) ;
#25197=VERTEX_POINT ( 'NONE', #680 ) ;
#25199=DIRECTION ( 'NONE',  ( -1.101824276508909887E-16, 1.000000000000000000, -0.000000000000000000 ) ) ;
#25203=CIRCLE ( 'NONE', #13673, 0.1250000000000001110 ) ;
#25208=EDGE_LOOP ( 'NONE', ( #2097, #18411, #18508, #7371 ) ) ;
#25210=CIRCLE ( 'NONE', #30437, 0.1250000000000001110 ) ;
#25212=EDGE_CURVE ( 'NONE', #29229, #2570, #23682, .T. ) ;
#25213=EDGE_CURVE ( 'NONE', #24404, #17879, #24721, .T. ) ;
#25215=EDGE_CURVE ( 'NONE', #31644, #25156, #22103, .T. ) ;
#25216=AXIS2_PLACEMENT_3D ( 'NONE', #6691, #16686, #4235 ) ;
#25219=ORIENTED_EDGE ( 'NONE', *, *, #23635, .T. ) ;
#25222=CARTESIAN_POINT ( 'NONE',  ( 21.09992658989238734, 31.59164230456639544, 47.04930799450051637 ) ) ;
#25224=DIRECTION ( 'NONE',  ( 0.000000000000000000, -0.000000000000000000, -1.000000000000000000 ) ) ;
#25232=AXIS2_PLACEMENT_3D ( 'NONE', #9244, #3829, #16458 ) ;
#25237=DIRECTION ( 'NONE',  ( -1.101824276508909887E-16, 1.000000000000000000, -0.000000000000000000 ) ) ;
#25242=VERTEX_POINT ( 'NONE', #11450 ) ;
#25244=EDGE_CURVE ( 'NONE', #28626, #31841, #26302, .T. ) ;
#25247=EDGE_CURVE ( 'NONE', #2027, #27575, #10065, .T. ) ;
#25250=VERTEX_POINT ( 'NONE', #19639 ) ;
#25254=CIRCLE ( 'NONE', #19994, 12.36707279061065101 ) ;
#25255=EDGE_CURVE ( 'NONE', #1311, #21016, #10578, .T. ) ;
#25258=ORIENTED_EDGE ( 'NONE', *, *, #31685, .T. ) ;
#25265=ORIENTED_EDGE ( 'NONE', *, *, #1338, .F. ) ;
#25268=ADVANCED_FACE ( 'NONE', ( #22268 ), #25066, .F. ) ;
#25270=CONICAL_SURFACE ( 'NONE', #14191, 12.52247886585643499, 0.6248499269447925775 ) ;
#25273=AXIS2_PLACEMENT_3D ( 'NONE', #21539, #26321, #11228 ) ;
#25277=ORIENTED_EDGE ( 'NONE', *, *, #14034, .T. ) ;
#25279=DIRECTION ( 'NONE',  ( -1.000000000000000000, 0.000000000000000000, 0.000000000000000000 ) ) ;
#25289=CARTESIAN_POINT ( 'NONE',  ( 21.09992658989238734, 38.56284415653841791, 47.04930799450051637 ) ) ;
#25290=AXIS2_PLACEMENT_3D ( 'NONE', #562, #20098, #2705 ) ;
#25291=AXIS2_PLACEMENT_3D ( 'NONE', #6731, #24125, #6900 ) ;
#25292=EDGE_CURVE ( 'NONE', #23085, #28525, #12698, .T. ) ;
#25293=AXIS2_PLACEMENT_3D ( 'NONE', #7054, #16566, #32003 ) ;
#25294=ORIENTED_EDGE ( 'NONE', *, *, #15239, .F. ) ;
#25296=VERTEX_POINT ( 'NONE', #117 ) ;
#25308=DIRECTION ( 'NONE',  ( -1.101824276508909887E-16, 1.000000000000000000, -0.000000000000000000 ) ) ;
#25309=DIRECTION ( 'NONE',  ( -1.101824276508909887E-16, 1.000000000000000000, -0.000000000000000000 ) ) ;
#25311=CARTESIAN_POINT ( 'NONE',  ( 21.09992658989238734, 38.56284415653841791, 47.04930799450051637 ) ) ;
#25312=CIRCLE ( 'NONE', #10642, 0.1250000000000001110 ) ;
#25315=ORIENTED_EDGE ( 'NONE', *, *, #29199, .F. ) ;
#25319=CARTESIAN_POINT ( 'NONE',  ( 21.09992658989239089, 24.72145308207319303, 47.04930799450051637 ) ) ;
#25323=TOROIDAL_SURFACE ( 'NONE', #30551, 12.40141737965286772, 0.1250000000000003331 ) ;
#25325=CARTESIAN_POINT ( 'NONE',  ( 21.09992658989239089, 28.59164230456639544, 47.04930799450051637 ) ) ;
#25326=LINE ( 'NONE', #2829, #7323 ) ;
#25333=FACE_OUTER_BOUND ( 'NONE', #6856, .T. ) ;
#25334=ORIENTED_EDGE ( 'NONE', *, *, #9964, .T. ) ;
#25335=CIRCLE ( 'NONE', #6959, 0.1250000000000001110 ) ;
#25340=AXIS2_PLACEMENT_3D ( 'NONE', #21133, #3749, #30849 ) ;
#25346=CARTESIAN_POINT ( 'NONE',  ( 21.09992658989239089, 25.84164230456639899, 47.04930799450051637 ) ) ;
#25362=DIRECTION ( 'NONE',  ( 1.000000000000000000, 0.000000000000000000, 0.000000000000000000 ) ) ;
#25366=CARTESIAN_POINT ( 'NONE',  ( 33.46699938050304013, 24.96183152705960140, 47.04930799450051637 ) ) ;
#25376=EDGE_LOOP ( 'NONE', ( #30355, #28589, #6299, #29542 ) ) ;
#25384=ORIENTED_EDGE ( 'NONE', *, *, #860, .F. ) ;
#25386=LINE ( 'NONE', #17513, #25820 ) ;
#25390=DIRECTION ( 'NONE',  ( -1.101824276508909887E-16, 1.000000000000000000, -0.000000000000000000 ) ) ;
#25394=EDGE_CURVE ( 'NONE', #23085, #7990, #15538, .T. ) ;
#25400=CARTESIAN_POINT ( 'NONE',  ( 8.577447724035948795, 32.54735957529758394, 47.04930799450051637 ) ) ;
#25404=AXIS2_PLACEMENT_3D ( 'NONE', #16119, #30598, #23357 ) ;
#25407=CARTESIAN_POINT ( 'NONE',  ( 21.09992658989238734, 31.96664230456639544, 47.04930799450051637 ) ) ;
#25409=CIRCLE ( 'NONE', #11249, 12.62506659569710443 ) ;
#25414=CARTESIAN_POINT ( 'NONE',  ( 21.09992658989239089, 28.84164230456639544, 47.04930799450051637 ) ) ;
#25416=ORIENTED_EDGE ( 'NONE', *, *, #32207, .F. ) ;
#25417=VECTOR ( 'NONE', #26747, 1000.000000000000000 ) ;
#25418=DIRECTION ( 'NONE',  ( -1.000000000000000000, 0.000000000000000000, 0.000000000000000000 ) ) ;
#25421=TOROIDAL_SURFACE ( 'NONE', #21726, 12.61792373059858896, 0.1250000000000002220 ) ;
#25423=VERTEX_POINT ( 'NONE', #10792 ) ;
#25424=ORIENTED_EDGE ( 'NONE', *, *, #19205, .F. ) ;
#25426=DIRECTION ( 'NONE',  ( -1.000000000000000000, 0.000000000000000000, 0.000000000000000000 ) ) ;
#25430=TOROIDAL_SURFACE ( 'NONE', #11283, 12.40141737965283397, 0.1249999999999992922 ) ;
#25434=CARTESIAN_POINT ( 'NONE',  ( 8.732853799281738105, 27.96183152705961206, 47.04930799450051637 ) ) ;
#25435=EDGE_CURVE ( 'NONE', #28743, #31649, #11619, .T. ) ;
#25442=CARTESIAN_POINT ( 'NONE',  ( 21.09992658989238734, 38.56284415653841791, 47.04930799450051637 ) ) ;
#25456=DIRECTION ( 'NONE',  ( -1.101824276508909887E-16, 1.000000000000000000, -0.000000000000000000 ) ) ;
#25459=TOROIDAL_SURFACE ( 'NONE', #29653, 12.40141737965287128, 0.1249999999999993477 ) ;
#25460=ORIENTED_EDGE ( 'NONE', *, *, #20157, .F. ) ;
#25468=CARTESIAN_POINT ( 'NONE',  ( 21.09992658989238734, 38.56284415653841791, 47.04930799450051637 ) ) ;
#25469=DIRECTION ( 'NONE',  ( -1.101824276508909887E-16, 1.000000000000000000, -0.000000000000000000 ) ) ;
#25472=ORIENTED_EDGE ( 'NONE', *, *, #23971, .T. ) ;
#25475=CIRCLE ( 'NONE', #21278, 0.1250000000000001110 ) ;
#25478=CARTESIAN_POINT ( 'NONE',  ( 8.474859994195282908, 38.56284415653841791, 47.04930799450051637 ) ) ;
#25489=AXIS2_PLACEMENT_3D ( 'NONE', #11889, #26824, #12225 ) ;
#25491=EDGE_CURVE ( 'NONE', #13589, #25773, #1660, .T. ) ;
#25494=CYLINDRICAL_SURFACE ( 'NONE', #24546, 12.62506659569710443 ) ;
#25495=AXIS2_PLACEMENT_3D ( 'NONE', #19195, #16905, #6418 ) ;
#25500=ADVANCED_FACE ( 'NONE', ( #11414 ), #13566, .T. ) ;
#25502=CARTESIAN_POINT ( 'NONE',  ( 8.732853799281734553, 30.22145308207317527, 47.04930799450051637 ) ) ;
#25503=CIRCLE ( 'NONE', #11354, 12.62506659569710266 ) ;
#25506=CARTESIAN_POINT ( 'NONE',  ( 8.482002859293423569, 26.71664230456639899, 47.04930799450051637 ) ) ;
#25508=CARTESIAN_POINT ( 'NONE',  ( 33.46699938050304013, 30.72145308207317882, 47.04930799450050927 ) ) ;
#25517=DIRECTION ( 'NONE',  ( -1.101824276508909887E-16, 1.000000000000000000, -0.000000000000000000 ) ) ;
#25521=DIRECTION ( 'NONE',  ( -1.000000000000000000, 0.000000000000000000, 0.000000000000000000 ) ) ;
#25522=AXIS2_PLACEMENT_3D ( 'NONE', #8360, #10680, #20668 ) ;
#25523=CYLINDRICAL_SURFACE ( 'NONE', #11509, 12.36707279061065101 ) ;
#25524=DIRECTION ( 'NONE',  ( -1.000000000000000000, -1.101824276508909887E-16, 0.000000000000000000 ) ) ;
#25527=ORIENTED_EDGE ( 'NONE', *, *, #5035, .T. ) ;
#25529=VECTOR ( 'NONE', #5279, 1000.000000000000000 ) ;
#25531=ORIENTED_EDGE ( 'NONE', *, *, #17297, .T. ) ;
#25533=DIRECTION ( 'NONE',  ( -1.000000000000000000, -1.101824276508909887E-16, 0.000000000000000000 ) ) ;
#25553=CARTESIAN_POINT ( 'NONE',  ( 33.46699938050303302, 38.56284415653841791, 47.04930799450051637 ) ) ;
#25555=CARTESIAN_POINT ( 'NONE',  ( 21.09992658989239089, 25.59143805560860940, 47.04930799450051637 ) ) ;
#25556=EDGE_LOOP ( 'NONE', ( #24737, #18172, #30321, #25384 ) ) ;
#25559=EDGE_LOOP ( 'NONE', ( #2044, #17768, #29652, #22621 ) ) ;
#25561=FACE_OUTER_BOUND ( 'NONE', #19516, .T. ) ;
#25562=AXIS2_PLACEMENT_3D ( 'NONE', #8722, #30740, #16263 ) ;
#25569=EDGE_CURVE ( 'NONE', #4539, #11837, #28934, .T. ) ;
#25581=ORIENTED_EDGE ( 'NONE', *, *, #20403, .T. ) ;
#25582=CARTESIAN_POINT ( 'NONE',  ( 8.732853799281732776, 25.72145308207319303, 47.04930799450051637 ) ) ;
#25588=AXIS2_PLACEMENT_3D ( 'NONE', #15307, #7755, #10066 ) ;
#25597=CYLINDRICAL_SURFACE ( 'NONE', #5671, 12.36707279061065101 ) ;
#25599=DIRECTION ( 'NONE',  ( -1.000000000000000000, 0.000000000000000000, 0.000000000000000000 ) ) ;
#25604=CIRCLE ( 'NONE', #19832, 12.36707279061065101 ) ;
#25608=ADVANCED_FACE ( 'NONE', ( #17138 ), #5887, .T. ) ;
#25611=AXIS2_PLACEMENT_3D ( 'NONE', #21588, #31618, #16345 ) ;
#25615=CARTESIAN_POINT ( 'NONE',  ( 21.09992658989238734, 30.72145308207317882, 47.04930799450051637 ) ) ;
#25618=EDGE_LOOP ( 'NONE', ( #13879, #21274, #1364, #6178 ) ) ;
#25622=CYLINDRICAL_SURFACE ( 'NONE', #14549, 12.36707279061065279 ) ;
#25625=DIRECTION ( 'NONE',  ( -1.000000000000000000, -1.101824276508909887E-16, 0.000000000000000000 ) ) ;
#25631=VERTEX_POINT ( 'NONE', #26841 ) ;
#25633=CIRCLE ( 'NONE', #14628, 12.36707279061065101 ) ;
#25634=CARTESIAN_POINT ( 'NONE',  ( 21.09992658989239089, 24.09164230456639544, 47.04930799450051637 ) ) ;
#25636=DIRECTION ( 'NONE',  ( -1.101824276508909887E-16, 1.000000000000000000, -0.000000000000000000 ) ) ;
#25638=CARTESIAN_POINT ( 'NONE',  ( 21.09992658989238734, 32.34164230456639899, 47.04930799450051637 ) ) ;
#25641=ORIENTED_EDGE ( 'NONE', *, *, #24054, .F. ) ;
#25645=EDGE_CURVE ( 'NONE', #25156, #24129, #6392, .T. ) ;
#25650=EDGE_CURVE ( 'NONE', #3723, #25296, #16880, .T. ) ;
#25652=CARTESIAN_POINT ( 'NONE',  ( 8.482002859293434227, 27.71664230456639899, 47.04930799450051637 ) ) ;
#25654=TOROIDAL_SURFACE ( 'NONE', #30910, 12.40141737965282154, 0.1250000000000006939 ) ;
#25656=FACE_OUTER_BOUND ( 'NONE', #13624, .T. ) ;
#25668=CARTESIAN_POINT ( 'NONE',  ( 21.09992658989238734, 38.56284415653841791, 47.04930799450051637 ) ) ;
#25669=CARTESIAN_POINT ( 'NONE',  ( 8.482002859293475083, 32.21664230456639899, 47.04930799450051637 ) ) ;
#25670=FACE_OUTER_BOUND ( 'NONE', #2738, .T. ) ;
#25678=ORIENTED_EDGE ( 'NONE', *, *, #23311, .T. ) ;
#25679=DIRECTION ( 'NONE',  ( -1.101824276508909887E-16, 1.000000000000000000, -0.000000000000000000 ) ) ;
#25685=DIRECTION ( 'NONE',  ( 0.000000000000000000, -0.000000000000000000, -1.000000000000000000 ) ) ;
#25691=AXIS2_PLACEMENT_3D ( 'NONE', #7516, #32462, #1923 ) ;
#25694=CIRCLE ( 'NONE', #9979, 12.62506659569710266 ) ;
#25702=ORIENTED_EDGE ( 'NONE', *, *, #30706, .T. ) ;
#25705=DIRECTION ( 'NONE',  ( -1.000000000000000000, 0.000000000000000000, 0.000000000000000000 ) ) ;
#25707=DIRECTION ( 'NONE',  ( -1.101824276508909887E-16, 1.000000000000000000, -0.000000000000000000 ) ) ;
#25708=ADVANCED_FACE ( 'NONE', ( #14701 ), #7461, .T. ) ;
#25710=DIRECTION ( 'NONE',  ( -1.000000000000000000, 0.000000000000000000, 0.000000000000000000 ) ) ;
#25712=CARTESIAN_POINT ( 'NONE',  ( 33.50134396954528171, 23.59164230456639544, 47.04930799450051637 ) ) ;
#25714=ORIENTED_EDGE ( 'NONE', *, *, #3569, .F. ) ;
#25717=VECTOR ( 'NONE', #15202, 1000.000000000000000 ) ;
#25719=DIRECTION ( 'NONE',  ( -1.101824276508909887E-16, 1.000000000000000000, -0.000000000000000000 ) ) ;
#25720=CARTESIAN_POINT ( 'NONE',  ( 8.474859994195282908, 38.56284415653841791, 47.04930799450051637 ) ) ;
#25721=CARTESIAN_POINT ( 'NONE',  ( 8.732853799281738105, 27.46183152705960850, 47.04930799450051637 ) ) ;
#25722=DIRECTION ( 'NONE',  ( -1.000000000000000000, 0.000000000000000000, 0.000000000000000000 ) ) ;
#25724=VERTEX_POINT ( 'NONE', #25194 ) ;
#25725=CIRCLE ( 'NONE', #5271, 0.1250000000000001110 ) ;
#25729=AXIS2_PLACEMENT_3D ( 'NONE', #21261, #16978, #11588 ) ;
#25735=AXIS2_PLACEMENT_3D ( 'NONE', #7345, #24743, #7679 ) ;
#25745=FACE_OUTER_BOUND ( 'NONE', #15413, .T. ) ;
#25747=ORIENTED_EDGE ( 'NONE', *, *, #1766, .F. ) ;
#25748=ORIENTED_EDGE ( 'NONE', *, *, #8740, .F. ) ;
#25749=DIRECTION ( 'NONE',  ( -1.101824276508909887E-16, 1.000000000000000000, -0.000000000000000000 ) ) ;
#25754=DIRECTION ( 'NONE',  ( -1.101824276508909887E-16, 1.000000000000000000, -0.000000000000000000 ) ) ;
#25755=CYLINDRICAL_SURFACE ( 'NONE', #25340, 12.36707279061065101 ) ;
#25758=EDGE_CURVE ( 'NONE', #27623, #13790, #6925, .T. ) ;
#25759=CIRCLE ( 'NONE', #1128, 0.1250000000000001110 ) ;
#25762=FACE_OUTER_BOUND ( 'NONE', #15949, .T. ) ;
#25763=AXIS2_PLACEMENT_3D ( 'NONE', #2711, #20103, #19770 ) ;
#25766=VERTEX_POINT ( 'NONE', #3014 ) ;
#25773=VERTEX_POINT ( 'NONE', #13051 ) ;
#25774=AXIS2_PLACEMENT_3D ( 'NONE', #22957, #7882, #2786 ) ;
#25777=AXIS2_PLACEMENT_3D ( 'NONE', #18276, #18441, #13057 ) ;
#25779=DIRECTION ( 'NONE',  ( -1.000000000000000000, 0.000000000000000000, 0.000000000000000000 ) ) ;
#25782=CARTESIAN_POINT ( 'NONE',  ( 8.474859994195281132, 30.84184655352422411, 47.04930799450051637 ) ) ;
#25783=CARTESIAN_POINT ( 'NONE',  ( 21.09992658989239089, 29.34164230456639899, 47.04930799450051637 ) ) ;
#25784=DIRECTION ( 'NONE',  ( -1.000000000000000000, -1.101824276508909764E-16, 0.000000000000000000 ) ) ;
#25787=SURFACE_STYLE_FILL_AREA ( #23802 ) ;
#25793=EDGE_CURVE ( 'NONE', #18578, #4682, #15118, .T. ) ;
#25794=DIRECTION ( 'NONE',  ( -1.101824276508909887E-16, 1.000000000000000000, -0.000000000000000000 ) ) ;
#25795=AXIS2_PLACEMENT_3D ( 'NONE', #29827, #20126, #17661 ) ;
#25797=ORIENTED_EDGE ( 'NONE', *, *, #21617, .F. ) ;
#25802=CARTESIAN_POINT ( 'NONE',  ( 33.72499318558949710, 25.84143805560860940, 47.04930799450051637 ) ) ;
#25806=CIRCLE ( 'NONE', #13240, 12.62506659569710266 ) ;
#25810=DIRECTION ( 'NONE',  ( -1.101824276508909887E-16, 1.000000000000000000, -0.000000000000000000 ) ) ;
#25815=AXIS2_PLACEMENT_3D ( 'NONE', #12146, #12304, #17698 ) ;
#25817=EDGE_CURVE ( 'NONE', #12300, #23862, #28221, .T. ) ;
#25818=DIRECTION ( 'NONE',  ( -1.224646799147353207E-16, -1.349345573449484691E-32, 1.000000000000000000 ) ) ;
#25820=VECTOR ( 'NONE', #20456, 1000.000000000000000 ) ;
#25831=FACE_OUTER_BOUND ( 'NONE', #26932, .T. ) ;
#25835=DIRECTION ( 'NONE',  ( -1.000000000000000000, -1.101824276508909887E-16, 0.000000000000000000 ) ) ;
#25838=ADVANCED_FACE ( 'NONE', ( #25670 ), #21918, .T. ) ;
#25840=CARTESIAN_POINT ( 'NONE',  ( 8.698509210239503631, 23.84164230456639544, 47.04930799450051637 ) ) ;
#25843=EDGE_LOOP ( 'NONE', ( #25990, #24499, #1740, #16274 ) ) ;
#25853=DIRECTION ( 'NONE',  ( -1.101824276508909887E-16, 1.000000000000000000, -0.000000000000000000 ) ) ;
#25861=CARTESIAN_POINT ( 'NONE',  ( 8.474859994195282908, 38.56284415653841791, 47.04930799450051637 ) ) ;
#25864=CYLINDRICAL_SURFACE ( 'NONE', #18368, 12.36707279061065279 ) ;
#25867=DIRECTION ( 'NONE',  ( -1.000000000000000000, 0.000000000000000000, 0.000000000000000000 ) ) ;
#25870=DIRECTION ( 'NONE',  ( 0.000000000000000000, -0.000000000000000000, -1.000000000000000000 ) ) ;
#25874=DIRECTION ( 'NONE',  ( -1.101824276508909887E-16, 1.000000000000000000, -0.000000000000000000 ) ) ;
#25876=AXIS2_PLACEMENT_3D ( 'NONE', #12035, #16944, #3995 ) ;
#25879=ORIENTED_EDGE ( 'NONE', *, *, #15239, .T. ) ;
#25880=CIRCLE ( 'NONE', #713, 12.62506659569710443 ) ;
#25888=ORIENTED_EDGE ( 'NONE', *, *, #23351, .F. ) ;
#25895=VERTEX_POINT ( 'NONE', #8598 ) ;
#25902=CARTESIAN_POINT ( 'NONE',  ( 21.09992658989238734, 38.56284415653841791, 47.04930799450051637 ) ) ;
#25905=ORIENTED_EDGE ( 'NONE', *, *, #3569, .T. ) ;
#25906=VERTEX_POINT ( 'NONE', #18911 ) ;
#25909=AXIS2_PLACEMENT_3D ( 'NONE', #12681, #30230, #2329 ) ;
#25914=CARTESIAN_POINT ( 'NONE',  ( 8.732853799281732776, 38.56284415653841791, 47.04930799450051637 ) ) ;
#25917=CYLINDRICAL_SURFACE ( 'NONE', #5221, 12.62506659569710266 ) ;
#25919=ORIENTED_EDGE ( 'NONE', *, *, #371, .F. ) ;
#25923=ADVANCED_FACE ( 'NONE', ( #11541 ), #7789, .T. ) ;
#25932=EDGE_CURVE ( 'NONE', #1400, #11991, #13527, .T. ) ;
#25935=CARTESIAN_POINT ( 'NONE',  ( 21.09992658989239089, 23.84164230456639544, 47.04930799450051637 ) ) ;
#25943=DIRECTION ( 'NONE',  ( -1.101824276508909887E-16, 1.000000000000000000, -0.000000000000000000 ) ) ;
#25944=DIRECTION ( 'NONE',  ( -1.101824276508909887E-16, 1.000000000000000000, -0.000000000000000000 ) ) ;
#25946=ORIENTED_EDGE ( 'NONE', *, *, #18874, .T. ) ;
#25949=DIRECTION ( 'NONE',  ( -1.000000000000000000, 0.000000000000000000, 0.000000000000000000 ) ) ;
#25951=ORIENTED_EDGE ( 'NONE', *, *, #16881, .F. ) ;
#25956=CARTESIAN_POINT ( 'NONE',  ( 8.732853799281738105, 30.47145308207317882, 47.04930799450051637 ) ) ;
#25959=AXIS2_PLACEMENT_3D ( 'NONE', #13561, #18306, #3217 ) ;
#25967=EDGE_CURVE ( 'NONE', #22254, #32203, #30302, .T. ) ;
#25970=ADVANCED_FACE ( 'NONE', ( #18432 ), #23845, .T. ) ;
#25971=ADVANCED_FACE ( 'NONE', ( #3827 ), #1465, .T. ) ;
#25975=CIRCLE ( 'NONE', #17596, 12.62506659569710266 ) ;
#25978=ORIENTED_EDGE ( 'NONE', *, *, #2349, .T. ) ;
#25982=CYLINDRICAL_SURFACE ( 'NONE', #10570, 12.36707279061065101 ) ;
#25984=DIRECTION ( 'NONE',  ( -1.000000000000000000, 0.000000000000000000, 0.000000000000000000 ) ) ;
#25987=DIRECTION ( 'NONE',  ( -1.101824276508909887E-16, 1.000000000000000000, -0.000000000000000000 ) ) ;
#25990=ORIENTED_EDGE ( 'NONE', *, *, #21145, .T. ) ;
#25993=DIRECTION ( 'NONE',  ( 0.000000000000000000, -0.000000000000000000, -1.000000000000000000 ) ) ;
#25998=FACE_OUTER_BOUND ( 'NONE', #27354, .T. ) ;
#26003=AXIS2_PLACEMENT_3D ( 'NONE', #5614, #18549, #3135 ) ;
#26006=AXIS2_PLACEMENT_3D ( 'NONE', #22540, #10090, #20086 ) ;
#26012=ORIENTED_EDGE ( 'NONE', *, *, #12985, .F. ) ;
#26014=EDGE_LOOP ( 'NONE', ( #6734, #19037, #27078, #20599 ) ) ;
#26015=CARTESIAN_POINT ( 'NONE',  ( 21.09992658989239089, 24.09184655352419213, 47.04930799450051637 ) ) ;
#26019=ORIENTED_EDGE ( 'NONE', *, *, #23480, .T. ) ;
#26020=CARTESIAN_POINT ( 'NONE',  ( 21.09992658989239089, 27.96183152705961206, 47.04930799450051637 ) ) ;
#26023=TOROIDAL_SURFACE ( 'NONE', #8731, 12.40141737965287305, 0.1250000000000000833 ) ;
#26024=LINE ( 'NONE', #13564, #15287 ) ;
#26033=DIRECTION ( 'NONE',  ( -1.000000000000000000, -1.101824276508909887E-16, 0.000000000000000000 ) ) ;
#26037=TOROIDAL_SURFACE ( 'NONE', #17123, 12.61792373059894068, 0.1249999999999991118 ) ;
#26042=FACE_OUTER_BOUND ( 'NONE', #4384, .T. ) ;
#26043=ADVANCED_FACE ( 'NONE', ( #24326 ), #10396, .T. ) ;
#26045=ORIENTED_EDGE ( 'NONE', *, *, #31985, .F. ) ;
#26051=CARTESIAN_POINT ( 'NONE',  ( 33.50134396954525329, 26.09164230456639899, 47.04930799450051637 ) ) ;
#26055=ORIENTED_EDGE ( 'NONE', *, *, #28029, .F. ) ;
#26056=ORIENTED_EDGE ( 'NONE', *, *, #17488, .T. ) ;
#26058=ORIENTED_EDGE ( 'NONE', *, *, #4157, .T. ) ;
#26059=DIRECTION ( 'NONE',  ( -1.101824276508909887E-16, 1.000000000000000000, -0.000000000000000000 ) ) ;
#26061=CIRCLE ( 'NONE', #11916, 12.36707279061065101 ) ;
#26070=DIRECTION ( 'NONE',  ( -1.000000000000000000, 0.000000000000000000, 0.000000000000000000 ) ) ;
#26072=EDGE_CURVE ( 'NONE', #27014, #28135, #4612, .T. ) ;
#26076=AXIS2_PLACEMENT_3D ( 'NONE', #1687, #11709, #9571 ) ;
#26078=DIRECTION ( 'NONE',  ( -1.000000000000000000, 0.000000000000000000, 0.000000000000000000 ) ) ;
#26080=ADVANCED_FACE ( 'NONE', ( #5133 ), #27457, .F. ) ;
#26081=EDGE_CURVE ( 'NONE', #12497, #17250, #3036, .T. ) ;
#26082=AXIS2_PLACEMENT_3D ( 'NONE', #28968, #29286, #4012 ) ;
#26085=VERTEX_POINT ( 'NONE', #20061 ) ;
#26086=DIRECTION ( 'NONE',  ( -1.224646799147353207E-16, -1.349345573449484691E-32, 1.000000000000000000 ) ) ;
#26090=AXIS2_PLACEMENT_3D ( 'NONE', #17500, #27516, #7162 ) ;
#26092=AXIS2_PLACEMENT_3D ( 'NONE', #12735, #20255, #28302 ) ;
#26094=VECTOR ( 'NONE', #2101, 1000.000000000000000 ) ;
#26099=ORIENTED_EDGE ( 'NONE', *, *, #27050, .T. ) ;
#26102=DIRECTION ( 'NONE',  ( -1.101824276508909887E-16, 1.000000000000000000, -0.000000000000000000 ) ) ;
#26105=ADVANCED_FACE ( 'NONE', ( #15463 ), #19821, .T. ) ;
#26106=( LENGTH_UNIT ( ) NAMED_UNIT ( * ) SI_UNIT ( .MILLI., .METRE. ) );
#26107=ORIENTED_EDGE ( 'NONE', *, *, #913, .F. ) ;
#26109=DIRECTION ( 'NONE',  ( -1.101824276508909887E-16, 1.000000000000000000, -0.000000000000000000 ) ) ;
#26110=CARTESIAN_POINT ( 'NONE',  ( 21.09992658989238734, 31.84184655352418503, 47.04930799450051637 ) ) ;
#26117=CARTESIAN_POINT ( 'NONE',  ( 33.72499318558949710, 27.59143805560860940, 47.04930799450051637 ) ) ;
#26119=AXIS2_PLACEMENT_3D ( 'NONE', #6107, #1177, #18248 ) ;
#26121=ADVANCED_FACE ( 'NONE', ( #22845 ), #16668, .T. ) ;
#26128=TOROIDAL_SURFACE ( 'NONE', #29289, 12.61792373059895134, 0.1249999999999985151 ) ;
#26130=DIRECTION ( 'NONE',  ( 0.000000000000000000, -0.000000000000000000, -1.000000000000000000 ) ) ;
#26136=AXIS2_PLACEMENT_3D ( 'NONE', #26746, #19673, #29702 ) ;
#26139=FACE_OUTER_BOUND ( 'NONE', #30942, .T. ) ;
#26140=TOROIDAL_SURFACE ( 'NONE', #4122, 12.40141737965288193, 0.1250000000000005829 ) ;
#26147=CARTESIAN_POINT ( 'NONE',  ( 33.46699938050304013, 32.21183152705962272, 47.04930799450051637 ) ) ;
#26152=ORIENTED_EDGE ( 'NONE', *, *, #5837, .F. ) ;
#26160=ADVANCED_FACE ( 'NONE', ( #689 ), #6210, .T. ) ;
#26164=ADVANCED_FACE ( 'NONE', ( #8088 ), #31915, .T. ) ;
#26167=CIRCLE ( 'NONE', #12574, 12.36707279061065101 ) ;
#26172=CARTESIAN_POINT ( 'NONE',  ( 21.09992658989239089, 23.72145308207319658, 47.04930799450051637 ) ) ;
#26174=ORIENTED_EDGE ( 'NONE', *, *, #20482, .F. ) ;
#26177=DIRECTION ( 'NONE',  ( -1.101824276508909887E-16, 1.000000000000000000, -0.000000000000000000 ) ) ;
#26178=FACE_OUTER_BOUND ( 'NONE', #31455, .T. ) ;
#26182=FACE_OUTER_BOUND ( 'NONE', #12051, .T. ) ;
#26183=DIRECTION ( 'NONE',  ( -1.101824276508909887E-16, 1.000000000000000000, -0.000000000000000000 ) ) ;
#26184=CYLINDRICAL_SURFACE ( 'NONE', #4864, 12.36707279061065279 ) ;
#26189=CARTESIAN_POINT ( 'NONE',  ( 33.46699938050302592, 31.97145308207317882, 47.04930799450050927 ) ) ;
#26193=ORIENTED_EDGE ( 'NONE', *, *, #6439, .F. ) ;
#26198=AXIS2_PLACEMENT_3D ( 'NONE', #14668, #17274, #17108 ) ;
#26201=ADVANCED_FACE ( 'NONE', ( #11188 ), #26140, .T. ) ;
#26215=AXIS2_PLACEMENT_3D ( 'NONE', #30870, #3447, #3608 ) ;
#26218=TOROIDAL_SURFACE ( 'NONE', #12089, 12.40141737965280200, 0.1249999999999999445 ) ;
#26223=EDGE_CURVE ( 'NONE', #12384, #15696, #4641, .T. ) ;
#26225=EDGE_LOOP ( 'NONE', ( #16845, #6726, #21885, #18663 ) ) ;
#26226=DIRECTION ( 'NONE',  ( -1.000000000000000000, 0.000000000000000000, 0.000000000000000000 ) ) ;
#26227=EDGE_CURVE ( 'NONE', #13441, #116, #30349, .T. ) ;
#26229=ORIENTED_EDGE ( 'NONE', *, *, #7233, .F. ) ;
#26232=LINE ( 'NONE', #13605, #10253 ) ;
#26236=DIRECTION ( 'NONE',  ( -1.101824276508909887E-16, 1.000000000000000000, -0.000000000000000000 ) ) ;
#26237=ORIENTED_EDGE ( 'NONE', *, *, #13279, .F. ) ;
#26239=CARTESIAN_POINT ( 'NONE',  ( 33.50134396954518934, 32.09164230456639899, 47.04930799450051637 ) ) ;
#26243=DIRECTION ( 'NONE',  ( -1.101824276508909887E-16, 1.000000000000000000, -0.000000000000000000 ) ) ;
#26247=LINE ( 'NONE', #19169, #16214 ) ;
#26252=CIRCLE ( 'NONE', #12103, 12.36707279061065101 ) ;
#26259=CARTESIAN_POINT ( 'NONE',  ( 33.72499318558949000, 38.56284415653841791, 47.04930799450051637 ) ) ;
#26261=EDGE_CURVE ( 'NONE', #1392, #11505, #23658, .T. ) ;
#26268=CARTESIAN_POINT ( 'NONE',  ( 33.72499318558949710, 25.09184655352419213, 47.04930799450051637 ) ) ;
#26269=ADVANCED_FACE ( 'NONE', ( #1161 ), #3467, .F. ) ;
#26274=CIRCLE ( 'NONE', #32038, 0.1250000000000001110 ) ;
#26275=FACE_OUTER_BOUND ( 'NONE', #7012, .T. ) ;
#26278=ORIENTED_EDGE ( 'NONE', *, *, #3782, .F. ) ;
#26280=AXIS2_PLACEMENT_3D ( 'NONE', #29145, #18950, #28823 ) ;
#26282=FACE_OUTER_BOUND ( 'NONE', #22632, .T. ) ;
#26283=VERTEX_POINT ( 'NONE', #5942 ) ;
#26287=LINE ( 'NONE', #6427, #29368 ) ;
#26293=DIRECTION ( 'NONE',  ( -1.101824276508909887E-16, 1.000000000000000000, -0.000000000000000000 ) ) ;
#26302=CIRCLE ( 'NONE', #13742, 12.62506659569710443 ) ;
#26304=ADVANCED_FACE ( 'NONE', ( #28739 ), #23966, .T. ) ;
#26317=DIRECTION ( 'NONE',  ( -1.101824276508909887E-16, 1.000000000000000000, -0.000000000000000000 ) ) ;
#26320=CARTESIAN_POINT ( 'NONE',  ( 8.698509210239560474, 29.34164230456639899, 47.04930799450051637 ) ) ;
#26321=DIRECTION ( 'NONE',  ( -1.101824276508909887E-16, 1.000000000000000000, -0.000000000000000000 ) ) ;
#26322=CARTESIAN_POINT ( 'NONE',  ( 21.09992658989238734, 38.56284415653841791, 47.04930799450051637 ) ) ;
#26330=VERTEX_POINT ( 'NONE', #14297 ) ;
#26332=VECTOR ( 'NONE', #12801, 1000.000000000000000 ) ;
#26337=CARTESIAN_POINT ( 'NONE',  ( 21.09992658989239089, 23.96183152705959785, 47.04930799450051637 ) ) ;
#26340=ORIENTED_EDGE ( 'NONE', *, *, #21358, .T. ) ;
#26342=CARTESIAN_POINT ( 'NONE',  ( 33.50134396954528171, 23.84164230456639544, 47.04930799450051637 ) ) ;
#26348=CARTESIAN_POINT ( 'NONE',  ( 8.823509210239521394, 25.59164230456639899, 47.04930799450051637 ) ) ;
#26349=DIRECTION ( 'NONE',  ( -1.101824276508909887E-16, 1.000000000000000000, -0.000000000000000000 ) ) ;
#26356=DIRECTION ( 'NONE',  ( -1.000000000000000000, 0.000000000000000000, 0.000000000000000000 ) ) ;
#26362=CYLINDRICAL_SURFACE ( 'NONE', #5675, 12.62506659569710266 ) ;
#26363=DIRECTION ( 'NONE',  ( -1.101824276508909887E-16, 1.000000000000000000, -0.000000000000000000 ) ) ;
#26365=AXIS2_PLACEMENT_3D ( 'NONE', #28995, #32108, #29154 ) ;
#26372=AXIS2_PLACEMENT_3D ( 'NONE', #29169, #26869, #6197 ) ;
#26376=DIRECTION ( 'NONE',  ( -1.000000000000000000, 0.000000000000000000, 0.000000000000000000 ) ) ;
#26377=TOROIDAL_SURFACE ( 'NONE', #7536, 12.61792373059859962, 0.1250000000000011380 ) ;
#26382=AXIS2_PLACEMENT_3D ( 'NONE', #30778, #23383, #15992 ) ;
#26393=DIRECTION ( 'NONE',  ( -1.224646799147353207E-16, -1.349345573449484691E-32, 1.000000000000000000 ) ) ;
#26394=DIRECTION ( 'NONE',  ( -1.000000000000000000, 0.000000000000000000, 0.000000000000000000 ) ) ;
#26395=LINE ( 'NONE', #1769, #23063 ) ;
#26406=CARTESIAN_POINT ( 'NONE',  ( 21.09992658989239089, 23.96183152705959785, 47.04930799450051637 ) ) ;
#26407=ORIENTED_EDGE ( 'NONE', *, *, #7757, .F. ) ;
#26423=DIRECTION ( 'NONE',  ( 1.000000000000000000, 0.000000000000000000, 0.000000000000000000 ) ) ;
#26424=CARTESIAN_POINT ( 'NONE',  ( 21.09992658989238734, 38.56284415653841791, 47.04930799450051637 ) ) ;
#26428=ORIENTED_EDGE ( 'NONE', *, *, #18551, .T. ) ;
#26429=CIRCLE ( 'NONE', #12295, 12.27641737965286772 ) ;
#26431=CARTESIAN_POINT ( 'NONE',  ( 21.09992658989239089, 28.59184655352419213, 47.04930799450051637 ) ) ;
#26432=DIRECTION ( 'NONE',  ( -1.224646799147353207E-16, -1.349345573449484691E-32, 1.000000000000000000 ) ) ;
#26433=SHAPE_REPRESENTATION_RELATIONSHIP ( 'NONE' , 'NONE' ,  #14743, #12811 ) ;
#26437=CARTESIAN_POINT ( 'NONE',  ( 21.09992658989238734, 38.56284415653841791, 47.04930799450051637 ) ) ;
#26441=DIRECTION ( 'NONE',  ( -1.101824276508909887E-16, 1.000000000000000000, -0.000000000000000000 ) ) ;
#26446=CYLINDRICAL_SURFACE ( 'NONE', #24823, 12.62506659569710266 ) ;
#26450=CIRCLE ( 'NONE', #31705, 12.62506659569710266 ) ;
#26459=ORIENTED_EDGE ( 'NONE', *, *, #3221, .F. ) ;
#26460=CARTESIAN_POINT ( 'NONE',  ( 33.46699938050303302, 38.56284415653841791, 47.04930799450051637 ) ) ;
#26461=DIRECTION ( 'NONE',  ( -1.101824276508909887E-16, 1.000000000000000000, -0.000000000000000000 ) ) ;
#26462=EDGE_CURVE ( 'NONE', #21567, #19469, #30368, .T. ) ;
#26464=DIRECTION ( 'NONE',  ( -1.101824276508909887E-16, 1.000000000000000000, -0.000000000000000000 ) ) ;
#26475=AXIS2_PLACEMENT_3D ( 'NONE', #30966, #11107, #28650 ) ;
#26484=ORIENTED_EDGE ( 'NONE', *, *, #29684, .T. ) ;
#26488=DIRECTION ( 'NONE',  ( 1.000000000000000000, 0.000000000000000000, 0.000000000000000000 ) ) ;
#26489=ADVANCED_FACE ( 'NONE', ( #22321 ), #22961, .F. ) ;
#26496=ADVANCED_FACE ( 'NONE', ( #28067 ), #15267, .F. ) ;
#26497=AXIS2_PLACEMENT_3D ( 'NONE', #12527, #22513, #46 ) ;
#26501=CARTESIAN_POINT ( 'NONE',  ( 21.09992658989239089, 25.84143805560860940, 47.04930799450051637 ) ) ;
#26503=TOROIDAL_SURFACE ( 'NONE', #27023, 12.40141737965282509, 0.1249999999999980849 ) ;
#26506=EDGE_LOOP ( 'NONE', ( #24735, #20001, #29278, #2875 ) ) ;
#26509=ORIENTED_EDGE ( 'NONE', *, *, #29543, .F. ) ;
#26511=LINE ( 'NONE', #28976, #21552 ) ;
#26516=CARTESIAN_POINT ( 'NONE',  ( 21.09992658989238734, 38.56284415653841791, 47.04930799450051637 ) ) ;
#26518=LINE ( 'NONE', #31289, #1064 ) ;
#26520=CYLINDRICAL_SURFACE ( 'NONE', #22575, 12.36707279061065101 ) ;
#26523=LINE ( 'NONE', #21750, #740 ) ;
#26530=DIRECTION ( 'NONE',  ( -1.101824276508909887E-16, 1.000000000000000000, -0.000000000000000000 ) ) ;
#26531=VERTEX_POINT ( 'NONE', #22475 ) ;
#26537=CIRCLE ( 'NONE', #9784, 12.62506659569710266 ) ;
#26549=DIRECTION ( 'NONE',  ( -1.101824276508909887E-16, 1.000000000000000000, -0.000000000000000000 ) ) ;
#26550=CARTESIAN_POINT ( 'NONE',  ( 8.732853799281729223, 26.72145308207318948, 47.04930799450051637 ) ) ;
#26551=TOROIDAL_SURFACE ( 'NONE', #10325, 12.61792373059898331, 0.1249999999999965583 ) ;
#26557=CARTESIAN_POINT ( 'NONE',  ( 33.37634396954523908, 27.09164230456639899, 47.04930799450051637 ) ) ;
#26559=FACE_OUTER_BOUND ( 'NONE', #23333, .T. ) ;
#26560=CARTESIAN_POINT ( 'NONE',  ( 21.09992658989239089, 29.71664230456640254, 47.04930799450051637 ) ) ;
#26561=CARTESIAN_POINT ( 'NONE',  ( 8.732853799281732776, 28.47145308207318237, 47.04930799450051637 ) ) ;
#26567=DIRECTION ( 'NONE',  ( -1.101824276508909887E-16, 1.000000000000000000, -0.000000000000000000 ) ) ;
#26568=CIRCLE ( 'NONE', #1397, 12.62506659569710266 ) ;
#26571=ADVANCED_FACE ( 'NONE', ( #5580 ), #9844, .T. ) ;
#26572=EDGE_CURVE ( 'NONE', #27727, #27500, #10025, .T. ) ;
#26573=ADVANCED_FACE ( 'NONE', ( #14946 ), #31333, .T. ) ;
#26574=ORIENTED_EDGE ( 'NONE', *, *, #28617, .F. ) ;
#26577=DIRECTION ( 'NONE',  ( 1.000000000000000000, 0.000000000000000000, 0.000000000000000000 ) ) ;
#26578=EDGE_LOOP ( 'NONE', ( #14182, #5161, #23057, #10815 ) ) ;
#26579=CARTESIAN_POINT ( 'NONE',  ( 21.09992658989239089, 25.97145308207318593, 47.04930799450051637 ) ) ;
#26582=AXIS2_PLACEMENT_3D ( 'NONE', #13657, #6099, #3634 ) ;
#26596=LINE ( 'NONE', #23659, #20356 ) ;
#26598=CARTESIAN_POINT ( 'NONE',  ( 21.09992658989239089, 27.59164230456639544, 47.04930799450051637 ) ) ;
#26600=ORIENTED_EDGE ( 'NONE', *, *, #21617, .T. ) ;
#26601=CARTESIAN_POINT ( 'NONE',  ( 33.72499318558949710, 30.59143805560860585, 47.04930799450051637 ) ) ;
#26602=DIRECTION ( 'NONE',  ( -1.000000000000000000, 0.000000000000000000, 0.000000000000000000 ) ) ;
#26604=ADVANCED_FACE ( 'NONE', ( #13460 ), #31332, .F. ) ;
#26605=ADVANCED_FACE ( 'NONE', ( #23458 ), #19787, .T. ) ;
#26608=ADVANCED_FACE ( 'NONE', ( #28552 ), #28195, .T. ) ;
#26612=DIRECTION ( 'NONE',  ( -1.101824276508909887E-16, 1.000000000000000000, -0.000000000000000000 ) ) ;
#26616=AXIS2_PLACEMENT_3D ( 'NONE', #6967, #16963, #14851 ) ;
#26619=DIRECTION ( 'NONE',  ( -1.000000000000000000, 0.000000000000000000, 0.000000000000000000 ) ) ;
#26627=EDGE_CURVE ( 'NONE', #25250, #19596, #12993, .T. ) ;
#26628=DIRECTION ( 'NONE',  ( 0.000000000000000000, -0.000000000000000000, -1.000000000000000000 ) ) ;
#26642=FACE_OUTER_BOUND ( 'NONE', #11392, .T. ) ;
#26645=AXIS2_PLACEMENT_3D ( 'NONE', #1836, #29088, #1347 ) ;
#26650=EDGE_CURVE ( 'NONE', #17679, #30342, #27197, .T. ) ;
#26652=CARTESIAN_POINT ( 'NONE',  ( 21.09992658989238734, 32.21664230456639899, 47.04930799450051637 ) ) ;
#26654=AXIS2_PLACEMENT_3D ( 'NONE', #11911, #14543, #12572 ) ;
#26657=FACE_OUTER_BOUND ( 'NONE', #26999, .T. ) ;
#26664=DIRECTION ( 'NONE',  ( -1.101824276508909887E-16, 1.000000000000000000, -0.000000000000000000 ) ) ;
#26666=ORIENTED_EDGE ( 'NONE', *, *, #1320, .F. ) ;
#26669=CARTESIAN_POINT ( 'NONE',  ( 8.732853799281738105, 30.21183152705961561, 47.04930799450051637 ) ) ;
#26671=EDGE_CURVE ( 'NONE', #3483, #154, #22407, .T. ) ;
#26672=ORIENTED_EDGE ( 'NONE', *, *, #14233, .F. ) ;
#26673=CARTESIAN_POINT ( 'NONE',  ( 8.698509210239587119, 32.34164230456639899, 47.04930799450051637 ) ) ;
#26677=EDGE_CURVE ( 'NONE', #17732, #27591, #4663, .T. ) ;
#26682=EDGE_LOOP ( 'NONE', ( #3068, #9824, #30264, #24696 ) ) ;
#26685=AXIS2_PLACEMENT_3D ( 'NONE', #6555, #11806, #19333 ) ;
#26687=ORIENTED_EDGE ( 'NONE', *, *, #29691, .T. ) ;
#26694=AXIS2_PLACEMENT_3D ( 'NONE', #16010, #8630, #3695 ) ;
#26695=AXIS2_PLACEMENT_3D ( 'NONE', #21712, #14509, #11877 ) ;
#26697=ORIENTED_EDGE ( 'NONE', *, *, #19661, .T. ) ;
#26711=AXIS2_PLACEMENT_3D ( 'NONE', #15313, #4812, #14834 ) ;
#26716=EDGE_CURVE ( 'NONE', #24189, #31962, #21421, .T. ) ;
#26718=AXIS2_PLACEMENT_3D ( 'NONE', #2917, #22932, #20307 ) ;
#26723=CIRCLE ( 'NONE', #31438, 12.50967055512594150 ) ;
#26728=VERTEX_POINT ( 'NONE', #14262 ) ;
#26731=DIRECTION ( 'NONE',  ( -1.101824276508909887E-16, 1.000000000000000000, -0.000000000000000000 ) ) ;
#26732=DIRECTION ( 'NONE',  ( -1.000000000000000000, -1.101824276508909887E-16, 0.000000000000000000 ) ) ;
#26734=CIRCLE ( 'NONE', #17284, 12.62506659569710266 ) ;
#26736=AXIS2_PLACEMENT_3D ( 'NONE', #13129, #23126, #643 ) ;
#26739=ORIENTED_EDGE ( 'NONE', *, *, #29684, .F. ) ;
#26740=CIRCLE ( 'NONE', #9983, 12.62506659569710266 ) ;
#26746=CARTESIAN_POINT ( 'NONE',  ( 21.09992658989239089, 28.09164230456639544, 47.04930799450051637 ) ) ;
#26747=DIRECTION ( 'NONE',  ( -1.101824276508909887E-16, 1.000000000000000000, -0.000000000000000000 ) ) ;
#26750=EDGE_LOOP ( 'NONE', ( #29267, #12411, #2931, #12090 ) ) ;
#26752=AXIS2_PLACEMENT_3D ( 'NONE', #2175, #20051, #26952 ) ;
#26753=ADVANCED_FACE ( 'NONE', ( #24094 ), #19653, .F. ) ;
#26754=ORIENTED_EDGE ( 'NONE', *, *, #28861, .F. ) ;
#26758=ORIENTED_EDGE ( 'NONE', *, *, #22972, .F. ) ;
#26766=TOROIDAL_SURFACE ( 'NONE', #31990, 12.61792373059860850, 0.1249999999999999445 ) ;
#26768=EDGE_LOOP ( 'NONE', ( #24875, #6072, #18889, #29800 ) ) ;
#26770=AXIS2_PLACEMENT_3D ( 'NONE', #27523, #30158, #4711 ) ;
#26773=CIRCLE ( 'NONE', #12634, 12.62506659569710266 ) ;
#26774=DIRECTION ( 'NONE',  ( -1.101824276508909887E-16, 1.000000000000000000, -0.000000000000000000 ) ) ;
#26779=DIRECTION ( 'NONE',  ( -1.224646799147353207E-16, -1.349345573449484691E-32, 1.000000000000000000 ) ) ;
#26788=DIRECTION ( 'NONE',  ( -1.000000000000000000, -1.101824276508909887E-16, 0.000000000000000000 ) ) ;
#26790=ADVANCED_FACE ( 'NONE', ( #21793 ), #20309, .T. ) ;
#26791=CYLINDRICAL_SURFACE ( 'NONE', #15798, 12.62506659569710266 ) ;
#26799=DIRECTION ( 'NONE',  ( -1.101824276508909887E-16, 1.000000000000000000, -0.000000000000000000 ) ) ;
#26804=VERTEX_POINT ( 'NONE', #26561 ) ;
#26806=CARTESIAN_POINT ( 'NONE',  ( 8.823509210239503631, 23.84164230456639544, 47.04930799450051637 ) ) ;
#26814=CIRCLE ( 'NONE', #5342, 0.1249999999999983763 ) ;
#26817=AXIS2_PLACEMENT_3D ( 'NONE', #27334, #12569, #22558 ) ;
#26823=AXIS2_PLACEMENT_3D ( 'NONE', #12440, #7177, #22424 ) ;
#26824=DIRECTION ( 'NONE',  ( -1.101824276508909887E-16, 1.000000000000000000, -0.000000000000000000 ) ) ;
#26826=CARTESIAN_POINT ( 'NONE',  ( 33.50134396954518934, 32.09164230456639899, 47.04930799450051637 ) ) ;
#26830=CIRCLE ( 'NONE', #24131, 0.1250000000000001110 ) ;
#26831=CIRCLE ( 'NONE', #12714, 0.1250000000000001110 ) ;
#26833=AXIS2_PLACEMENT_3D ( 'NONE', #28307, #26962, #19409 ) ;
#26837=EDGE_LOOP ( 'NONE', ( #1917, #31525, #5886, #810 ) ) ;
#26841=CARTESIAN_POINT ( 'NONE',  ( 33.37634396954522487, 28.84164230456639544, 47.04930799450051637 ) ) ;
#26843=DIRECTION ( 'NONE',  ( -1.000000000000000000, -1.101824276508909887E-16, 0.000000000000000000 ) ) ;
#26857=ORIENTED_EDGE ( 'NONE', *, *, #17149, .F. ) ;
#26862=CARTESIAN_POINT ( 'NONE',  ( 33.72499318558949000, 38.56284415653841791, 47.04930799450051637 ) ) ;
#26865=FACE_OUTER_BOUND ( 'NONE', #31020, .T. ) ;
#26866=CIRCLE ( 'NONE', #32109, 12.62506659569710443 ) ;
#26868=CYLINDRICAL_SURFACE ( 'NONE', #6584, 12.62506659569710266 ) ;
#26869=DIRECTION ( 'NONE',  ( 0.000000000000000000, -0.000000000000000000, -1.000000000000000000 ) ) ;
#26873=CARTESIAN_POINT ( 'NONE',  ( 33.50134396954519644, 31.59164230456639544, 47.04930799450051637 ) ) ;
#26878=DIRECTION ( 'NONE',  ( 0.000000000000000000, -0.000000000000000000, -1.000000000000000000 ) ) ;
#26880=DIRECTION ( 'NONE',  ( -1.101824276508909887E-16, 1.000000000000000000, -0.000000000000000000 ) ) ;
#26882=AXIS2_PLACEMENT_3D ( 'NONE', #22240, #29975, #410 ) ;
#26885=ORIENTED_EDGE ( 'NONE', *, *, #2452, .F. ) ;
#26888=CARTESIAN_POINT ( 'NONE',  ( 8.698509210239588896, 32.59164230456639899, 47.04930799450051637 ) ) ;
#26889=DIRECTION ( 'NONE',  ( -1.101824276508909887E-16, 1.000000000000000000, -0.000000000000000000 ) ) ;
#26891=EDGE_LOOP ( 'NONE', ( #30109, #12562, #18525, #9818 ) ) ;
#26895=DIRECTION ( 'NONE',  ( -1.101824276508909887E-16, 1.000000000000000000, -0.000000000000000000 ) ) ;
#26901=EDGE_CURVE ( 'NONE', #5223, #32221, #26723, .T. ) ;
#26905=VECTOR ( 'NONE', #31973, 1000.000000000000000 ) ;
#26908=CARTESIAN_POINT ( 'NONE',  ( 33.46699938050304013, 29.22145308207318237, 47.04930799450050927 ) ) ;
#26909=CARTESIAN_POINT ( 'NONE',  ( 21.09992658989239089, 27.21664230456639899, 47.04930799450051637 ) ) ;
#26914=ORIENTED_EDGE ( 'NONE', *, *, #2721, .F. ) ;
#26918=CARTESIAN_POINT ( 'NONE',  ( 33.46699938050304013, 25.46183152705960140, 47.04930799450051637 ) ) ;
#26919=CIRCLE ( 'NONE', #19029, 12.62506659569710266 ) ;
#26928=ORIENTED_EDGE ( 'NONE', *, *, #4971, .F. ) ;
#26931=EDGE_CURVE ( 'NONE', #12816, #12417, #27230, .T. ) ;
#26932=EDGE_LOOP ( 'NONE', ( #19773, #11177, #26960, #22853 ) ) ;
#26935=DIRECTION ( 'NONE',  ( -1.101824276508909887E-16, 1.000000000000000000, -0.000000000000000000 ) ) ;
#26937=EDGE_CURVE ( 'NONE', #22536, #32221, #10483, .T. ) ;
#26939=AXIS2_PLACEMENT_3D ( 'NONE', #3090, #7879, #15418 ) ;
#26948=DIRECTION ( 'NONE',  ( 1.000000000000000000, 0.000000000000000000, 0.000000000000000000 ) ) ;
#26952=DIRECTION ( 'NONE',  ( -1.000000000000000000, 0.000000000000000000, 0.000000000000000000 ) ) ;
#26960=ORIENTED_EDGE ( 'NONE', *, *, #28144, .T. ) ;
#26962=DIRECTION ( 'NONE',  ( 0.000000000000000000, -0.000000000000000000, -1.000000000000000000 ) ) ;
#26966=ORIENTED_EDGE ( 'NONE', *, *, #16149, .F. ) ;
#26968=AXIS2_PLACEMENT_3D ( 'NONE', #2001, #11256, #12020 ) ;
#26971=CIRCLE ( 'NONE', #1282, 0.1250000000000001110 ) ;
#26972=DIRECTION ( 'NONE',  ( 1.000000000000000000, 0.000000000000000000, 0.000000000000000000 ) ) ;
#26979=ORIENTED_EDGE ( 'NONE', *, *, #6304, .F. ) ;
#26981=EDGE_CURVE ( 'NONE', #31427, #2267, #4175, .T. ) ;
#26982=EDGE_CURVE ( 'NONE', #4576, #593, #30421, .T. ) ;
#26986=LINE ( 'NONE', #14520, #27590 ) ;
#26989=CARTESIAN_POINT ( 'NONE',  ( 33.72499318558949710, 24.09184655352419213, 47.04930799450051637 ) ) ;
#26991=CIRCLE ( 'NONE', #12867, 12.36707279061065101 ) ;
#26995=CIRCLE ( 'NONE', #9711, 12.36707279061065101 ) ;
#26996=CARTESIAN_POINT ( 'NONE',  ( 21.09992658989238734, 38.56284415653841791, 47.04930799450051637 ) ) ;
#26999=EDGE_LOOP ( 'NONE', ( #934, #15253, #24965, #23101 ) ) ;
#27001=DIRECTION ( 'NONE',  ( -1.101824276508909887E-16, 1.000000000000000000, -0.000000000000000000 ) ) ;
#27006=ORIENTED_EDGE ( 'NONE', *, *, #18887, .F. ) ;
#27011=LINE ( 'NONE', #19120, #18993 ) ;
#27014=VERTEX_POINT ( 'NONE', #12905 ) ;
#27016=CIRCLE ( 'NONE', #25959, 12.62506659569710266 ) ;
#27018=AXIS2_PLACEMENT_3D ( 'NONE', #19099, #8943, #4507 ) ;
#27023=AXIS2_PLACEMENT_3D ( 'NONE', #16885, #12299, #24279 ) ;
#27024=CARTESIAN_POINT ( 'NONE',  ( 33.72499318558949710, 28.59184655352419213, 47.04930799450051637 ) ) ;
#27025=ORIENTED_EDGE ( 'NONE', *, *, #22662, .F. ) ;
#27028=DIRECTION ( 'NONE',  ( -1.101824276508909887E-16, 1.000000000000000000, -0.000000000000000000 ) ) ;
#27031=CARTESIAN_POINT ( 'NONE',  ( 21.09992658989239089, 24.59164230456639544, 47.04930799450051637 ) ) ;
#27035=CIRCLE ( 'NONE', #31751, 0.1250000000000001110 ) ;
#27038=CARTESIAN_POINT ( 'NONE',  ( 21.09992658989239089, 24.09143805560860940, 47.04930799450051637 ) ) ;
#27039=CARTESIAN_POINT ( 'NONE',  ( 21.09992658989239089, 28.96183152705961206, 47.04930799450051637 ) ) ;
#27047=CARTESIAN_POINT ( 'NONE',  ( 21.09992658989239089, 28.97145308207318237, 47.04930799450051637 ) ) ;
#27050=EDGE_CURVE ( 'NONE', #28202, #16423, #22528, .T. ) ;
#27058=VECTOR ( 'NONE', #15943, 1000.000000000000000 ) ;
#27060=DIRECTION ( 'NONE',  ( -1.000000000000000000, 0.000000000000000000, 0.000000000000000000 ) ) ;
#27063=AXIS2_PLACEMENT_3D ( 'NONE', #17707, #14612, #1963 ) ;
#27064=ORIENTED_EDGE ( 'NONE', *, *, #1706, .F. ) ;
#27065=LINE ( 'NONE', #1954, #20887 ) ;
#27069=ORIENTED_EDGE ( 'NONE', *, *, #19045, .T. ) ;
#27077=CARTESIAN_POINT ( 'NONE',  ( 21.09992658989239089, 28.09184655352419213, 47.04930799450051637 ) ) ;
#27078=ORIENTED_EDGE ( 'NONE', *, *, #15759, .T. ) ;
#27079=ORIENTED_EDGE ( 'NONE', *, *, #11937, .T. ) ;
#27080=DIRECTION ( 'NONE',  ( 1.000000000000000000, 0.000000000000000000, 0.000000000000000000 ) ) ;
#27081=ADVANCED_FACE ( 'NONE', ( #13700 ), #5244, .T. ) ;
#27085=EDGE_CURVE ( 'NONE', #14523, #11099, #13630, .T. ) ;
#27086=DIRECTION ( 'NONE',  ( -1.101824276508909887E-16, 1.000000000000000000, -0.000000000000000000 ) ) ;
#27092=DIRECTION ( 'NONE',  ( -1.000000000000000000, -1.101824276508909764E-16, 0.000000000000000000 ) ) ;
#27093=AXIS2_PLACEMENT_3D ( 'NONE', #21974, #20174, #25107 ) ;
#27097=ORIENTED_EDGE ( 'NONE', *, *, #19102, .F. ) ;
#27105=DIRECTION ( 'NONE',  ( -1.000000000000000000, 0.000000000000000000, 0.000000000000000000 ) ) ;
#27110=DIRECTION ( 'NONE',  ( 1.000000000000000000, 0.000000000000000000, 0.000000000000000000 ) ) ;
#27111=DIRECTION ( 'NONE',  ( -1.000000000000000000, 0.000000000000000000, 0.000000000000000000 ) ) ;
#27126=DIRECTION ( 'NONE',  ( -1.000000000000000000, 0.000000000000000000, 0.000000000000000000 ) ) ;
#27128=DIRECTION ( 'NONE',  ( -1.000000000000000000, -1.101824276508909887E-16, 0.000000000000000000 ) ) ;
#27131=DIRECTION ( 'NONE',  ( -1.101824276508909887E-16, 1.000000000000000000, -0.000000000000000000 ) ) ;
#27133=CIRCLE ( 'NONE', #6675, 12.27641737965281266 ) ;
#27134=DIRECTION ( 'NONE',  ( -1.000000000000000000, 0.000000000000000000, 0.000000000000000000 ) ) ;
#27138=AXIS2_PLACEMENT_3D ( 'NONE', #23044, #15656, #15504 ) ;
#27149=ORIENTED_EDGE ( 'NONE', *, *, #13988, .T. ) ;
#27158=EDGE_CURVE ( 'NONE', #32103, #27500, #6269, .T. ) ;
#27159=DIRECTION ( 'NONE',  ( -1.101824276508909887E-16, 1.000000000000000000, -0.000000000000000000 ) ) ;
#27160=CIRCLE ( 'NONE', #1474, 0.1249999999999983763 ) ;
#27161=EDGE_CURVE ( 'NONE', #3559, #3723, #23038, .T. ) ;
#27164=DIRECTION ( 'NONE',  ( -1.224646799147353207E-16, -1.349345573449484691E-32, 1.000000000000000000 ) ) ;
#27176=CIRCLE ( 'NONE', #20902, 12.36707279061065101 ) ;
#27182=CARTESIAN_POINT ( 'NONE',  ( 8.482002859293427122, 26.96664230456639899, 47.04930799450051637 ) ) ;
#27184=CYLINDRICAL_SURFACE ( 'NONE', #26770, 12.62506659569710266 ) ;
#27188=DIRECTION ( 'NONE',  ( -1.101824276508909887E-16, 1.000000000000000000, -0.000000000000000000 ) ) ;
#27191=EDGE_LOOP ( 'NONE', ( #12665, #6904, #3376, #13726 ) ) ;
#27197=CIRCLE ( 'NONE', #11400, 12.27641737965283042 ) ;
#27201=EDGE_CURVE ( 'NONE', #27623, #30099, #11079, .T. ) ;
#27204=ADVANCED_FACE ( 'NONE', ( #26642 ), #18444, .T. ) ;
#27209=VECTOR ( 'NONE', #1448, 1000.000000000000000 ) ;
#27214=EDGE_LOOP ( 'NONE', ( #15108, #30682, #31138, #15376 ) ) ;
#27215=AXIS2_PLACEMENT_3D ( 'NONE', #13251, #30641, #28334 ) ;
#27216=AXIS2_PLACEMENT_3D ( 'NONE', #15837, #3354, #405 ) ;
#27217=ORIENTED_EDGE ( 'NONE', *, *, #23688, .F. ) ;
#27221=ADVANCED_FACE ( 'NONE', ( #9747 ), #2122, .T. ) ;
#27222=AXIS2_PLACEMENT_3D ( 'NONE', #31856, #13980, #21832 ) ;
#27223=CIRCLE ( 'NONE', #15710, 0.1250000000000001110 ) ;
#27230=CIRCLE ( 'NONE', #13111, 12.36707279061065101 ) ;
#27233=CYLINDRICAL_SURFACE ( 'NONE', #29599, 12.36707279061065101 ) ;
#27234=ORIENTED_EDGE ( 'NONE', *, *, #14633, .T. ) ;
#27236=DIRECTION ( 'NONE',  ( -1.000000000000000000, -1.101824276508909887E-16, 0.000000000000000000 ) ) ;
#27237=DIRECTION ( 'NONE',  ( -1.000000000000000000, -1.101824276508909764E-16, 0.000000000000000000 ) ) ;
#27242=CARTESIAN_POINT ( 'NONE',  ( 33.50134396954524618, 26.59164230456639899, 47.04930799450051637 ) ) ;
#27244=CARTESIAN_POINT ( 'NONE',  ( 21.09992658989239089, 25.22145308207319303, 47.04930799450051637 ) ) ;
#27247=CARTESIAN_POINT ( 'NONE',  ( 21.09992658989238734, 31.34143805560860585, 47.04930799450051637 ) ) ;
#27249=FACE_OUTER_BOUND ( 'NONE', #14040, .T. ) ;
#27257=TOROIDAL_SURFACE ( 'NONE', #31464, 12.40141737965282687, 0.1250000000000004718 ) ;
#27264=DIRECTION ( 'NONE',  ( -1.101824276508909887E-16, 1.000000000000000000, -0.000000000000000000 ) ) ;
#27266=CONICAL_SURFACE ( 'NONE', #31468, 12.52247886585643499, 0.6248499269447925775 ) ;
#27270=CARTESIAN_POINT ( 'NONE',  ( 8.698509210239555145, 28.84164230456639544, 47.04930799450051637 ) ) ;
#27273=AXIS2_PLACEMENT_3D ( 'NONE', #7311, #24705, #9281 ) ;
#27275=DIRECTION ( 'NONE',  ( -1.101824276508909887E-16, 1.000000000000000000, -0.000000000000000000 ) ) ;
#27278=DIRECTION ( 'NONE',  ( -1.000000000000000000, 0.000000000000000000, 0.000000000000000000 ) ) ;
#27286=CIRCLE ( 'NONE', #22490, 12.36707279061065279 ) ;
#27292=ORIENTED_EDGE ( 'NONE', *, *, #4213, .F. ) ;
#27295=FACE_OUTER_BOUND ( 'NONE', #6325, .T. ) ;
#27296=DIRECTION ( 'NONE',  ( -1.101824276508909887E-16, 1.000000000000000000, -0.000000000000000000 ) ) ;
#27298=EDGE_LOOP ( 'NONE', ( #22113, #31389, #15053, #11972 ) ) ;
#27301=CARTESIAN_POINT ( 'NONE',  ( 8.732853799281732776, 23.72145308207319303, 47.04930799450051637 ) ) ;
#27311=CIRCLE ( 'NONE', #24158, 0.1249999999999983763 ) ;
#27318=DIRECTION ( 'NONE',  ( 1.000000000000000000, 0.000000000000000000, 0.000000000000000000 ) ) ;
#27326=CARTESIAN_POINT ( 'NONE',  ( 21.09992658989238734, 38.56284415653841791, 47.04930799450051637 ) ) ;
#27328=CARTESIAN_POINT ( 'NONE',  ( 33.50134396954524618, 26.84164230456639899, 47.04930799450051637 ) ) ;
#27330=DIRECTION ( 'NONE',  ( -1.101824276508909887E-16, 1.000000000000000000, -0.000000000000000000 ) ) ;
#27334=CARTESIAN_POINT ( 'NONE',  ( 21.09992658989239089, 25.71183152705960140, 47.04930799450051637 ) ) ;
#27339=TOROIDAL_SURFACE ( 'NONE', #27853, 12.40141737965282509, 0.1249999999999980849 ) ;
#27343=VERTEX_POINT ( 'NONE', #215 ) ;
#27344=VERTEX_POINT ( 'NONE', #20714 ) ;
#27354=EDGE_LOOP ( 'NONE', ( #30270, #30911, #30763, #9825 ) ) ;
#27359=CARTESIAN_POINT ( 'NONE',  ( 21.09992658989239089, 24.59184655352419213, 47.04930799450051637 ) ) ;
#27362=ORIENTED_EDGE ( 'NONE', *, *, #8574, .F. ) ;
#27365=AXIS2_PLACEMENT_3D ( 'NONE', #22390, #12240, #32422 ) ;
#27367=CARTESIAN_POINT ( 'NONE',  ( 21.09992658989239089, 24.84143805560860940, 47.04930799450051637 ) ) ;
#27368=FACE_OUTER_BOUND ( 'NONE', #16231, .T. ) ;
#27369=CARTESIAN_POINT ( 'NONE',  ( 8.482002859293418240, 26.21664230456639899, 47.04930799450051637 ) ) ;
#27370=CARTESIAN_POINT ( 'NONE',  ( 21.09992658989239089, 29.46664230456640254, 47.04930799450051637 ) ) ;
#27371=DIRECTION ( 'NONE',  ( -1.101824276508909887E-16, 1.000000000000000000, -0.000000000000000000 ) ) ;
#27379=ORIENTED_EDGE ( 'NONE', *, *, #20154, .T. ) ;
#27381=DIRECTION ( 'NONE',  ( 0.000000000000000000, -0.000000000000000000, -1.000000000000000000 ) ) ;
#27386=VERTEX_POINT ( 'NONE', #25802 ) ;
#27391=EDGE_CURVE ( 'NONE', #28369, #15187, #25181, .T. ) ;
#27392=ORIENTED_EDGE ( 'NONE', *, *, #14827, .T. ) ;
#27397=DIRECTION ( 'NONE',  ( -1.101824276508909887E-16, 1.000000000000000000, -0.000000000000000000 ) ) ;
#27400=CIRCLE ( 'NONE', #18492, 12.36707279061065101 ) ;
#27406=DIRECTION ( 'NONE',  ( -1.101824276508909887E-16, 1.000000000000000000, -0.000000000000000000 ) ) ;
#27420=EDGE_LOOP ( 'NONE', ( #27608, #6559, #12987, #6234 ) ) ;
#27422=CIRCLE ( 'NONE', #7507, 12.62506659569710266 ) ;
#27427=FACE_OUTER_BOUND ( 'NONE', #9407, .T. ) ;
#27433=ADVANCED_FACE ( 'NONE', ( #8250 ), #10498, .T. ) ;
#27439=CYLINDRICAL_SURFACE ( 'NONE', #19645, 12.36707279061065101 ) ;
#27443=DIRECTION ( 'NONE',  ( -1.000000000000000000, 0.000000000000000000, 0.000000000000000000 ) ) ;
#27446=DIRECTION ( 'NONE',  ( -1.000000000000000000, 0.000000000000000000, 0.000000000000000000 ) ) ;
#27450=TOROIDAL_SURFACE ( 'NONE', #31640, 12.61792373059894778, 0.1249999999999986539 ) ;
#27454=ORIENTED_EDGE ( 'NONE', *, *, #4109, .F. ) ;
#27457=CYLINDRICAL_SURFACE ( 'NONE', #13026, 12.36707279061065101 ) ;
#27468=EDGE_CURVE ( 'NONE', #3119, #1392, #19400, .T. ) ;
#27471=DIRECTION ( 'NONE',  ( -1.101824276508909887E-16, 1.000000000000000000, -0.000000000000000000 ) ) ;
#27472=VECTOR ( 'NONE', #27001, 1000.000000000000000 ) ;
#27477=DIRECTION ( 'NONE',  ( -1.101824276508909887E-16, 1.000000000000000000, -0.000000000000000000 ) ) ;
#27485=FACE_OUTER_BOUND ( 'NONE', #24097, .T. ) ;
#27486=AXIS2_PLACEMENT_3D ( 'NONE', #29741, #7584, #19548 ) ;
#27493=DIRECTION ( 'NONE',  ( -1.000000000000000000, 0.000000000000000000, 0.000000000000000000 ) ) ;
#27494=FACE_OUTER_BOUND ( 'NONE', #3166, .T. ) ;
#27498=DIRECTION ( 'NONE',  ( -1.000000000000000000, 0.000000000000000000, 0.000000000000000000 ) ) ;
#27500=VERTEX_POINT ( 'NONE', #28920 ) ;
#27502=DIRECTION ( 'NONE',  ( -1.224646799147353207E-16, -1.349345573449484691E-32, 1.000000000000000000 ) ) ;
#27505=EDGE_CURVE ( 'NONE', #17800, #19067, #26287, .T. ) ;
#27511=ORIENTED_EDGE ( 'NONE', *, *, #11315, .T. ) ;
#27516=DIRECTION ( 'NONE',  ( 0.000000000000000000, -0.000000000000000000, -1.000000000000000000 ) ) ;
#27517=ORIENTED_EDGE ( 'NONE', *, *, #29577, .T. ) ;
#27521=DIRECTION ( 'NONE',  ( -1.000000000000000000, 0.000000000000000000, 0.000000000000000000 ) ) ;
#27523=CARTESIAN_POINT ( 'NONE',  ( 21.09992658989238734, 38.56284415653841791, 47.04930799450051637 ) ) ;
#27531=DIRECTION ( 'NONE',  ( -1.101824276508909887E-16, 1.000000000000000000, -0.000000000000000000 ) ) ;
#27532=ADVANCED_FACE ( 'NONE', ( #11039 ), #27257, .T. ) ;
#27533=DIRECTION ( 'NONE',  ( -1.101824276508909887E-16, 1.000000000000000000, -0.000000000000000000 ) ) ;
#27534=DIRECTION ( 'NONE',  ( -1.000000000000000000, 0.000000000000000000, 0.000000000000000000 ) ) ;
#27540=AXIS2_PLACEMENT_3D ( 'NONE', #19521, #2461, #22314 ) ;
#27550=VERTEX_POINT ( 'NONE', #26117 ) ;
#27552=DIRECTION ( 'NONE',  ( -1.224646799147353207E-16, -1.349345573449484691E-32, 1.000000000000000000 ) ) ;
#27559=ORIENTED_EDGE ( 'NONE', *, *, #16373, .F. ) ;
#27561=DIRECTION ( 'NONE',  ( -1.000000000000000000, 0.000000000000000000, 0.000000000000000000 ) ) ;
#27566=CARTESIAN_POINT ( 'NONE',  ( 21.09992658989239089, 29.34184655352418858, 47.04930799450051637 ) ) ;
#27567=ORIENTED_EDGE ( 'NONE', *, *, #3782, .T. ) ;
#27568=VECTOR ( 'NONE', #28162, 1000.000000000000000 ) ;
#27570=DIRECTION ( 'NONE',  ( -1.000000000000000000, -1.101824276508909887E-16, 0.000000000000000000 ) ) ;
#27574=PRODUCT_CONTEXT ( 'NONE', #705, 'mechanical' ) ;
#27575=VERTEX_POINT ( 'NONE', #25956 ) ;
#27577=CARTESIAN_POINT ( 'NONE',  ( 8.732853799281738105, 26.71183152705960495, 47.04930799450051637 ) ) ;
#27578=CARTESIAN_POINT ( 'NONE',  ( 21.09992658989238734, 38.56284415653841791, 47.04930799450051637 ) ) ;
#27580=FACE_OUTER_BOUND ( 'NONE', #17715, .T. ) ;
#27582=EDGE_LOOP ( 'NONE', ( #12479, #31959, #7496, #13296 ) ) ;
#27586=DIRECTION ( 'NONE',  ( -1.101824276508909887E-16, 1.000000000000000000, -0.000000000000000000 ) ) ;
#27588=COLOUR_RGB ( '',0.7921568627450980005, 0.8196078431372548767, 0.9333333333333333481 ) ;
#27590=VECTOR ( 'NONE', #31753, 1000.000000000000000 ) ;
#27591=VERTEX_POINT ( 'NONE', #26601 ) ;
#27592=ORIENTED_EDGE ( 'NONE', *, *, #14572, .F. ) ;
#27600=LINE ( 'NONE', #12999, #20485 ) ;
#27608=ORIENTED_EDGE ( 'NONE', *, *, #9459, .T. ) ;
#27610=CARTESIAN_POINT ( 'NONE',  ( 21.09992658989239089, 30.09184655352422411, 47.04930799450051637 ) ) ;
#27621=DIRECTION ( 'NONE',  ( -1.101824276508909887E-16, 1.000000000000000000, -0.000000000000000000 ) ) ;
#27623=VERTEX_POINT ( 'NONE', #24630 ) ;
#27624=CARTESIAN_POINT ( 'NONE',  ( 33.71785032049132269, 29.71664230456640254, 47.04930799450051637 ) ) ;
#27625=ADVANCED_FACE ( 'NONE', ( #27249 ), #12332, .T. ) ;
#27628=FACE_OUTER_BOUND ( 'NONE', #23074, .T. ) ;
#27629=CARTESIAN_POINT ( 'NONE',  ( 8.474859994195282908, 38.56284415653841791, 47.04930799450051637 ) ) ;
#27631=ORIENTED_EDGE ( 'NONE', *, *, #2349, .F. ) ;
#27632=DIRECTION ( 'NONE',  ( -1.224646799147353207E-16, -1.349345573449484691E-32, 1.000000000000000000 ) ) ;
#27633=ORIENTED_EDGE ( 'NONE', *, *, #14424, .T. ) ;
#27638=ORIENTED_EDGE ( 'NONE', *, *, #19219, .F. ) ;
#27639=CARTESIAN_POINT ( 'NONE',  ( 8.482002859293789498, 30.46664230456641675, 47.04930799450051637 ) ) ;
#27641=AXIS2_PLACEMENT_3D ( 'NONE', #15930, #6407, #8708 ) ;
#27643=CARTESIAN_POINT ( 'NONE',  ( 33.50134396954521065, 30.09164230456639544, 47.04930799450051637 ) ) ;
#27646=DIRECTION ( 'NONE',  ( -1.000000000000000000, 0.000000000000000000, 0.000000000000000000 ) ) ;
#27647=VERTEX_POINT ( 'NONE', #4605 ) ;
#27650=CARTESIAN_POINT ( 'NONE',  ( 8.823509210239548040, 28.09164230456639544, 47.04930799450051637 ) ) ;
#27652=FACE_OUTER_BOUND ( 'NONE', #16217, .T. ) ;
#27655=FACE_OUTER_BOUND ( 'NONE', #23734, .T. ) ;
#27657=ORIENTED_EDGE ( 'NONE', *, *, #21747, .F. ) ;
#27665=DIRECTION ( 'NONE',  ( -1.101824276508909887E-16, 1.000000000000000000, -0.000000000000000000 ) ) ;
#27671=AXIS2_PLACEMENT_3D ( 'NONE', #29683, #7188, #22434 ) ;
#27676=EDGE_LOOP ( 'NONE', ( #16951, #6720, #15554, #31839 ) ) ;
#27677=AXIS2_PLACEMENT_3D ( 'NONE', #14811, #10209, #19714 ) ;
#27682=DIRECTION ( 'NONE',  ( -1.101824276508909887E-16, 1.000000000000000000, -0.000000000000000000 ) ) ;
#27684=DIRECTION ( 'NONE',  ( -1.000000000000000000, 0.000000000000000000, 0.000000000000000000 ) ) ;
#27689=DIRECTION ( 'NONE',  ( 0.000000000000000000, -0.000000000000000000, -1.000000000000000000 ) ) ;
#27691=CARTESIAN_POINT ( 'NONE',  ( 21.09992658989239089, 29.46183152705961206, 47.04930799450051637 ) ) ;
#27695=LINE ( 'NONE', #14744, #7407 ) ;
#27697=VERTEX_POINT ( 'NONE', #24306 ) ;
#27700=AXIS2_PLACEMENT_3D ( 'NONE', #3803, #8577, #704 ) ;
#27701=VERTEX_POINT ( 'NONE', #21677 ) ;
#27703=CIRCLE ( 'NONE', #19292, 12.36707279061065101 ) ;
#27706=ORIENTED_EDGE ( 'NONE', *, *, #2119, .F. ) ;
#27710=TOROIDAL_SURFACE ( 'NONE', #13552, 12.40141737965283220, 0.1250000000000002498 ) ;
#27713=ADVANCED_FACE ( 'NONE', ( #21834 ), #12559, .T. ) ;
#27714=EDGE_LOOP ( 'NONE', ( #28397, #25641, #10791, #708 ) ) ;
#27719=ORIENTED_EDGE ( 'NONE', *, *, #19134, .F. ) ;
#27722=FACE_OUTER_BOUND ( 'NONE', #8283, .T. ) ;
#27727=VERTEX_POINT ( 'NONE', #12823 ) ;
#27730=AXIS2_PLACEMENT_3D ( 'NONE', #29433, #14988, #17270 ) ;
#27731=DIRECTION ( 'NONE',  ( -1.101824276508909887E-16, 1.000000000000000000, -0.000000000000000000 ) ) ;
#27732=FACE_OUTER_BOUND ( 'NONE', #222, .T. ) ;
#27734=FACE_OUTER_BOUND ( 'NONE', #9502, .T. ) ;
#27738=VERTEX_POINT ( 'NONE', #327 ) ;
#27744=ORIENTED_EDGE ( 'NONE', *, *, #29871, .T. ) ;
#27748=CIRCLE ( 'NONE', #29321, 0.1250000000000018319 ) ;
#27750=AXIS2_PLACEMENT_3D ( 'NONE', #28877, #26243, #6067 ) ;
#27756=DIRECTION ( 'NONE',  ( -1.101824276508909887E-16, 1.000000000000000000, -0.000000000000000000 ) ) ;
#27757=EDGE_CURVE ( 'NONE', #63, #12709, #4228, .T. ) ;
#27759=EDGE_CURVE ( 'NONE', #11910, #4901, #20920, .T. ) ;
#27761=DIRECTION ( 'NONE',  ( -1.224646799147353207E-16, -1.349345573449484691E-32, 1.000000000000000000 ) ) ;
#27762=DIRECTION ( 'NONE',  ( 0.000000000000000000, -0.000000000000000000, -1.000000000000000000 ) ) ;
#27770=DIRECTION ( 'NONE',  ( -1.000000000000000000, 0.000000000000000000, 0.000000000000000000 ) ) ;
#27774=VERTEX_POINT ( 'NONE', #20512 ) ;
#27777=DIRECTION ( 'NONE',  ( -1.224646799147353207E-16, -1.349345573449484691E-32, 1.000000000000000000 ) ) ;
#27778=VECTOR ( 'NONE', #1694, 1000.000000000000000 ) ;
#27785=FACE_OUTER_BOUND ( 'NONE', #22686, .T. ) ;
#27792=DIRECTION ( 'NONE',  ( -1.000000000000000000, -1.101824276508910010E-16, 0.000000000000000000 ) ) ;
#27793=DIRECTION ( 'NONE',  ( -1.000000000000000000, 0.000000000000000000, 0.000000000000000000 ) ) ;
#27798=CIRCLE ( 'NONE', #6308, 12.36707279061065101 ) ;
#27799=AXIS2_PLACEMENT_3D ( 'NONE', #2959, #10530, #5596 ) ;
#27802=EDGE_CURVE ( 'NONE', #9593, #7848, #8211, .T. ) ;
#27803=AXIS2_PLACEMENT_3D ( 'NONE', #3460, #26432, #13488 ) ;
#27804=ADVANCED_FACE ( 'NONE', ( #10031 ), #15429, .T. ) ;
#27808=CIRCLE ( 'NONE', #30435, 0.1250000000000001110 ) ;
#27811=ORIENTED_EDGE ( 'NONE', *, *, #17618, .T. ) ;
#27814=CYLINDRICAL_SURFACE ( 'NONE', #4725, 12.36707279061065279 ) ;
#27820=AXIS2_PLACEMENT_3D ( 'NONE', #7959, #13043, #20576 ) ;
#27822=CARTESIAN_POINT ( 'NONE',  ( 33.37634396954522487, 28.59164230456639544, 47.04930799450051637 ) ) ;
#27825=DIRECTION ( 'NONE',  ( -1.000000000000000000, 0.000000000000000000, 0.000000000000000000 ) ) ;
#27828=CARTESIAN_POINT ( 'NONE',  ( 21.09992658989239089, 23.65414230456639544, 47.04930799450051637 ) ) ;
#27829=CARTESIAN_POINT ( 'NONE',  ( 21.09992658989239089, 29.96664230456641675, 47.04930799450051637 ) ) ;
#27837=AXIS2_PLACEMENT_3D ( 'NONE', #24734, #27682, #2249 ) ;
#27840=VERTEX_POINT ( 'NONE', #12979 ) ;
#27842=DIRECTION ( 'NONE',  ( -1.000000000000000000, 0.000000000000000000, 0.000000000000000000 ) ) ;
#27843=EDGE_CURVE ( 'NONE', #19672, #15022, #8428, .T. ) ;
#27846=DIRECTION ( 'NONE',  ( -1.101824276508909887E-16, 1.000000000000000000, -0.000000000000000000 ) ) ;
#27847=CIRCLE ( 'NONE', #3714, 12.27641737965280555 ) ;
#27849=LINE ( 'NONE', #30643, #703 ) ;
#27850=CARTESIAN_POINT ( 'NONE',  ( 21.09992658989238734, 38.56284415653841791, 47.04930799450051637 ) ) ;
#27853=AXIS2_PLACEMENT_3D ( 'NONE', #6015, #10458, #20454 ) ;
#27859=EDGE_LOOP ( 'NONE', ( #3535, #26697, #16549, #22480 ) ) ;
#27862=CARTESIAN_POINT ( 'NONE',  ( 8.732853799281734553, 38.56284415653841791, 47.04930799450051637 ) ) ;
#27866=DIRECTION ( 'NONE',  ( -1.101824276508909887E-16, 1.000000000000000000, -0.000000000000000000 ) ) ;
#27867=EDGE_CURVE ( 'NONE', #17879, #11837, #27286, .T. ) ;
#27872=AXIS2_PLACEMENT_3D ( 'NONE', #3128, #26549, #21290 ) ;
#27877=FACE_OUTER_BOUND ( 'NONE', #27888, .T. ) ;
#27879=ADVANCED_FACE ( 'NONE', ( #2475 ), #7302, .T. ) ;
#27882=AXIS2_PLACEMENT_3D ( 'NONE', #1733, #21749, #28826 ) ;
#27883=AXIS2_PLACEMENT_3D ( 'NONE', #24488, #22349, #14821 ) ;
#27888=EDGE_LOOP ( 'NONE', ( #19109, #9624, #26174, #1100 ) ) ;
#27900=CARTESIAN_POINT ( 'NONE',  ( 8.732853799281734553, 38.56284415653841791, 47.04930799450051637 ) ) ;
#27903=ORIENTED_EDGE ( 'NONE', *, *, #32080, .T. ) ;
#27906=EDGE_CURVE ( 'NONE', #27774, #414, #6388, .T. ) ;
#27910=DIRECTION ( 'NONE',  ( -1.000000000000000000, 0.000000000000000000, 0.000000000000000000 ) ) ;
#27911=CARTESIAN_POINT ( 'NONE',  ( 21.09992658989239089, 26.84184655352419568, 47.04930799450051637 ) ) ;
#27916=VECTOR ( 'NONE', #434, 1000.000000000000000 ) ;
#27917=EDGE_LOOP ( 'NONE', ( #16162, #12263, #11620, #23586 ) ) ;
#27923=VERTEX_POINT ( 'NONE', #18362 ) ;
#27929=CARTESIAN_POINT ( 'NONE',  ( 21.09992658989239089, 24.46664230456639899, 47.04930799450051637 ) ) ;
#27936=EDGE_CURVE ( 'NONE', #6910, #27923, #21507, .T. ) ;
#27940=CARTESIAN_POINT ( 'NONE',  ( 21.09992658989239089, 27.34164230456639544, 47.04930799450051637 ) ) ;
#27941=CARTESIAN_POINT ( 'NONE',  ( 21.09992658989238734, 31.22145308207317171, 47.04930799450051637 ) ) ;
#27943=CARTESIAN_POINT ( 'NONE',  ( 21.09992658989239089, 25.96183152705960140, 47.04930799450051637 ) ) ;
#27944=ORIENTED_EDGE ( 'NONE', *, *, #6002, .T. ) ;
#27947=CARTESIAN_POINT ( 'NONE',  ( 33.72499318558949000, 38.56284415653841791, 47.04930799450051637 ) ) ;
#27956=DIRECTION ( 'NONE',  ( -1.101824276508909887E-16, 1.000000000000000000, -0.000000000000000000 ) ) ;
#27958=AXIS2_PLACEMENT_3D ( 'NONE', #4031, #29146, #18951 ) ;
#27964=AXIS2_PLACEMENT_3D ( 'NONE', #22532, #27471, #5146 ) ;
#27972=FACE_OUTER_BOUND ( 'NONE', #10475, .T. ) ;
#27981=AXIS2_PLACEMENT_3D ( 'NONE', #31771, #6335, #16337 ) ;
#27984=FACE_OUTER_BOUND ( 'NONE', #6475, .T. ) ;
#27985=DIRECTION ( 'NONE',  ( -1.101824276508909887E-16, 1.000000000000000000, -0.000000000000000000 ) ) ;
#27988=CARTESIAN_POINT ( 'NONE',  ( 8.698509210239580014, 31.59164230456639544, 47.04930799450051637 ) ) ;
#27994=EDGE_CURVE ( 'NONE', #7860, #15433, #1594, .T. ) ;
#27998=ORIENTED_EDGE ( 'NONE', *, *, #19291, .F. ) ;
#28000=ORIENTED_EDGE ( 'NONE', *, *, #28710, .T. ) ;
#28002=CARTESIAN_POINT ( 'NONE',  ( 21.09992658989239089, 30.34164230456639544, 47.04930799450051637 ) ) ;
#28009=DIRECTION ( 'NONE',  ( -1.101824276508909887E-16, 1.000000000000000000, -0.000000000000000000 ) ) ;
#28015=ORIENTED_EDGE ( 'NONE', *, *, #18727, .T. ) ;
#28018=ORIENTED_EDGE ( 'NONE', *, *, #13182, .F. ) ;
#28022=CARTESIAN_POINT ( 'NONE',  ( 21.09992658989239089, 25.59184655352419213, 47.04930799450051637 ) ) ;
#28023=CYLINDRICAL_SURFACE ( 'NONE', #8937, 12.62506659569710266 ) ;
#28029=EDGE_CURVE ( 'NONE', #7677, #11017, #20410, .T. ) ;
#28031=ORIENTED_EDGE ( 'NONE', *, *, #1207, .F. ) ;
#28035=ORIENTED_EDGE ( 'NONE', *, *, #16334, .T. ) ;
#28043=CARTESIAN_POINT ( 'NONE',  ( 8.732853799281729223, 24.22145308207319303, 47.04930799450051637 ) ) ;
#28045=CIRCLE ( 'NONE', #1324, 12.36707279061065279 ) ;
#28047=FACE_OUTER_BOUND ( 'NONE', #6182, .T. ) ;
#28049=AXIS2_PLACEMENT_3D ( 'NONE', #23648, #1153, #20857 ) ;
#28051=EDGE_CURVE ( 'NONE', #272, #9936, #26247, .T. ) ;
#28056=ADVANCED_FACE ( 'NONE', ( #1619 ), #9177, .F. ) ;
#28058=EDGE_LOOP ( 'NONE', ( #4759, #2416, #12420, #31189 ) ) ;
#28060=CIRCLE ( 'NONE', #22801, 0.1250000000000001110 ) ;
#28066=DIRECTION ( 'NONE',  ( -1.000000000000000000, -1.101824276508909887E-16, 0.000000000000000000 ) ) ;
#28067=FACE_OUTER_BOUND ( 'NONE', #7051, .T. ) ;
#28075=CARTESIAN_POINT ( 'NONE',  ( 8.482002859293411134, 25.46664230456640254, 47.04930799450051637 ) ) ;
#28078=AXIS2_PLACEMENT_3D ( 'NONE', #14291, #20012, #5250 ) ;
#28088=EDGE_CURVE ( 'NONE', #22382, #3968, #1541, .T. ) ;
#28094=ADVANCED_FACE ( 'NONE', ( #4079 ), #4171, .T. ) ;
#28096=ADVANCED_FACE ( 'NONE', ( #24426 ), #10480, .T. ) ;
#28109=AXIS2_PLACEMENT_3D ( 'NONE', #15104, #24786, #22474 ) ;
#28114=DIRECTION ( 'NONE',  ( -1.101824276508909887E-16, 1.000000000000000000, -0.000000000000000000 ) ) ;
#28115=ORIENTED_EDGE ( 'NONE', *, *, #17860, .F. ) ;
#28116=ORIENTED_EDGE ( 'NONE', *, *, #13241, .F. ) ;
#28117=CARTESIAN_POINT ( 'NONE',  ( 21.09992658989239089, 26.34143805560860940, 47.04930799450051637 ) ) ;
#28119=EDGE_CURVE ( 'NONE', #31932, #28443, #15175, .T. ) ;
#28121=AXIS2_PLACEMENT_3D ( 'NONE', #7295, #32247, #25178 ) ;
#28123=ORIENTED_EDGE ( 'NONE', *, *, #16340, .T. ) ;
#28125=FACE_OUTER_BOUND ( 'NONE', #18418, .T. ) ;
#28126=TOROIDAL_SURFACE ( 'NONE', #1418, 12.40141737965286595, 0.1249999999999979183 ) ;
#28128=ADVANCED_FACE ( 'NONE', ( #16876 ), #11961, .F. ) ;
#28129=VERTEX_POINT ( 'NONE', #14589 ) ;
#28132=DIRECTION ( 'NONE',  ( -1.101824276508909887E-16, 1.000000000000000000, -0.000000000000000000 ) ) ;
#28134=CIRCLE ( 'NONE', #13984, 12.36707279061065101 ) ;
#28135=VERTEX_POINT ( 'NONE', #14755 ) ;
#28137=EDGE_CURVE ( 'NONE', #2041, #17732, #12033, .T. ) ;
#28140=LINE ( 'NONE', #15337, #20513 ) ;
#28143=CYLINDRICAL_SURFACE ( 'NONE', #19147, 12.62506659569710266 ) ;
#28144=EDGE_CURVE ( 'NONE', #11753, #25296, #19347, .T. ) ;
#28159=ORIENTED_EDGE ( 'NONE', *, *, #29500, .T. ) ;
#28162=DIRECTION ( 'NONE',  ( -1.101824276508909887E-16, 1.000000000000000000, -0.000000000000000000 ) ) ;
#28165=CIRCLE ( 'NONE', #4581, 0.1250000000000001110 ) ;
#28168=DIRECTION ( 'NONE',  ( -1.000000000000000000, 0.000000000000000000, 0.000000000000000000 ) ) ;
#28170=CARTESIAN_POINT ( 'NONE',  ( 21.09992658989239089, 29.96183152705961206, 47.04930799450051637 ) ) ;
#28171=CARTESIAN_POINT ( 'NONE',  ( 21.09992658989238734, 31.09143805560860585, 47.04930799450051637 ) ) ;
#28176=CARTESIAN_POINT ( 'NONE',  ( 21.09992658989239089, 26.84164230456639899, 47.04930799450051637 ) ) ;
#28181=CARTESIAN_POINT ( 'NONE',  ( 33.46699938050303302, 38.56284415653841791, 47.04930799450051637 ) ) ;
#28183=DIRECTION ( 'NONE',  ( -1.101824276508909887E-16, 1.000000000000000000, -0.000000000000000000 ) ) ;
#28190=CARTESIAN_POINT ( 'NONE',  ( 21.09992658989238734, 38.56284415653841791, 47.04930799450051637 ) ) ;
#28194=CIRCLE ( 'NONE', #7243, 12.62506659569710266 ) ;
#28195=TOROIDAL_SURFACE ( 'NONE', #17240, 12.40141737965283042, 0.1249999999999995420 ) ;
#28202=VERTEX_POINT ( 'NONE', #4737 ) ;
#28203=ADVANCED_FACE ( 'NONE', ( #6554 ), #18327, .T. ) ;
#28213=TOROIDAL_SURFACE ( 'NONE', #28746, 12.61792373059891048, 0.1250000000000026368 ) ;
#28214=VERTEX_POINT ( 'NONE', #15238 ) ;
#28215=FACE_OUTER_BOUND ( 'NONE', #27859, .T. ) ;
#28216=AXIS2_PLACEMENT_3D ( 'NONE', #10969, #14395, #1421 ) ;
#28218=DIRECTION ( 'NONE',  ( -1.224646799147353207E-16, -1.349345573449484691E-32, 1.000000000000000000 ) ) ;
#28221=CIRCLE ( 'NONE', #20330, 0.1250000000000001110 ) ;
#28222=TOROIDAL_SURFACE ( 'NONE', #15120, 12.40141737965281976, 0.1249999999999999722 ) ;
#28224=CARTESIAN_POINT ( 'NONE',  ( 33.72499318558949000, 38.56284415653841791, 47.04930799450051637 ) ) ;
#28225=EDGE_LOOP ( 'NONE', ( #5098, #7463, #1258, #18052 ) ) ;
#28236=ADVANCED_FACE ( 'NONE', ( #27877 ), #5394, .T. ) ;
#28237=CIRCLE ( 'NONE', #7270, 12.36707279061065101 ) ;
#28240=AXIS2_PLACEMENT_3D ( 'NONE', #2470, #12819, #7719 ) ;
#28241=CIRCLE ( 'NONE', #18264, 12.62506659569710266 ) ;
#28246=TOROIDAL_SURFACE ( 'NONE', #24551, 12.40141737965288193, 0.1250000000000005829 ) ;
#28250=DIRECTION ( 'NONE',  ( 1.000000000000000000, 0.000000000000000000, 0.000000000000000000 ) ) ;
#28251=ADVANCED_FACE ( 'NONE', ( #12946 ), #28296, .T. ) ;
#28253=DIRECTION ( 'NONE',  ( -1.000000000000000000, 0.000000000000000000, 0.000000000000000000 ) ) ;
#28256=DIRECTION ( 'NONE',  ( 1.101824276508909887E-16, -1.000000000000000000, 0.000000000000000000 ) ) ;
#28267=CYLINDRICAL_SURFACE ( 'NONE', #5647, 12.62506659569710266 ) ;
#28269=EDGE_CURVE ( 'NONE', #9505, #24311, #12587, .T. ) ;
#28274=ADVANCED_FACE ( 'NONE', ( #12625 ), #15551, .F. ) ;
#28275=AXIS2_PLACEMENT_3D ( 'NONE', #8841, #21139, #3757 ) ;
#28278=ADVANCED_FACE ( 'NONE', ( #25561 ), #6268, .T. ) ;
#28279=EDGE_CURVE ( 'NONE', #12476, #8369, #18826, .T. ) ;
#28281=CARTESIAN_POINT ( 'NONE',  ( 21.09992658989239089, 25.59143805560860940, 47.04930799450051637 ) ) ;
#28284=TOROIDAL_SURFACE ( 'NONE', #1536, 12.61792373059860850, 0.1249999999999999445 ) ;
#28291=ORIENTED_EDGE ( 'NONE', *, *, #22572, .F. ) ;
#28293=DIRECTION ( 'NONE',  ( -1.224646799147353207E-16, -1.349345573449484691E-32, 1.000000000000000000 ) ) ;
#28296=TOROIDAL_SURFACE ( 'NONE', #14146, 12.40141737965287128, 0.1249999999999993477 ) ;
#28297=CARTESIAN_POINT ( 'NONE',  ( 8.732853799281734553, 38.56284415653841791, 47.04930799450051637 ) ) ;
#28302=DIRECTION ( 'NONE',  ( 1.000000000000000000, 0.000000000000000000, 0.000000000000000000 ) ) ;
#28303=CARTESIAN_POINT ( 'NONE',  ( 8.577447724035948795, 32.54735957529758394, 47.04930799450051637 ) ) ;
#28307=CARTESIAN_POINT ( 'NONE',  ( 8.698509210239532052, 26.59164230456639899, 47.04930799450051637 ) ) ;
#28313=AXIS2_PLACEMENT_3D ( 'NONE', #24859, #25019, #2382 ) ;
#28315=DIRECTION ( 'NONE',  ( -1.000000000000000000, 0.000000000000000000, 0.000000000000000000 ) ) ;
#28321=CIRCLE ( 'NONE', #18848, 12.36707279061065101 ) ;
#28323=ORIENTED_EDGE ( 'NONE', *, *, #9064, .F. ) ;
#28324=ADVANCED_FACE ( 'NONE', ( #26042 ), #13431, .F. ) ;
#28326=CIRCLE ( 'NONE', #20973, 0.1250000000000001110 ) ;
#28328=DIRECTION ( 'NONE',  ( -1.000000000000000000, 0.000000000000000000, 0.000000000000000000 ) ) ;
#28332=DIRECTION ( 'NONE',  ( -1.000000000000000000, 0.000000000000000000, 0.000000000000000000 ) ) ;
#28334=DIRECTION ( 'NONE',  ( -1.000000000000000000, 0.000000000000000000, 0.000000000000000000 ) ) ;
#28337=DIRECTION ( 'NONE',  ( -1.101824276508909887E-16, 1.000000000000000000, -0.000000000000000000 ) ) ;
#28338=EDGE_LOOP ( 'NONE', ( #20457, #2923, #19253, #19532 ) ) ;
#28340=ORIENTED_EDGE ( 'NONE', *, *, #2006, .T. ) ;
#28344=ORIENTED_EDGE ( 'NONE', *, *, #2395, .F. ) ;
#28352=TOROIDAL_SURFACE ( 'NONE', #3683, 12.40141737965285529, 0.1250000000000000555 ) ;
#28353=DIRECTION ( 'NONE',  ( -1.101824276508909887E-16, 1.000000000000000000, -0.000000000000000000 ) ) ;
#28359=DIRECTION ( 'NONE',  ( -1.101824276508909887E-16, 1.000000000000000000, -0.000000000000000000 ) ) ;
#28361=VERTEX_POINT ( 'NONE', #7790 ) ;
#28362=ORIENTED_EDGE ( 'NONE', *, *, #12849, .F. ) ;
#28365=AXIS2_PLACEMENT_3D ( 'NONE', #27038, #1921, #22106 ) ;
#28367=ORIENTED_EDGE ( 'NONE', *, *, #16076, .T. ) ;
#28368=AXIS2_PLACEMENT_3D ( 'NONE', #15741, #25754, #8357 ) ;
#28369=VERTEX_POINT ( 'NONE', #7633 ) ;
#28370=MECHANICAL_DESIGN_GEOMETRIC_PRESENTATION_REPRESENTATION('',(#23140),#8457);
#28372=ORIENTED_EDGE ( 'NONE', *, *, #10985, .F. ) ;
#28378=ORIENTED_EDGE ( 'NONE', *, *, #28861, .T. ) ;
#28383=CARTESIAN_POINT ( 'NONE',  ( 33.46699938050304013, 31.21183152705961206, 47.04930799450051637 ) ) ;
#28384=LINE ( 'NONE', #5903, #24687 ) ;
#28387=DIRECTION ( 'NONE',  ( 0.000000000000000000, -0.000000000000000000, -1.000000000000000000 ) ) ;
#28389=AXIS2_PLACEMENT_3D ( 'NONE', #7308, #7795, #79 ) ;
#28392=AXIS2_PLACEMENT_3D ( 'NONE', #3547, #13572, #13099 ) ;
#28396=ADVANCED_FACE ( 'NONE', ( #554 ), #29957, .T. ) ;
#28397=ORIENTED_EDGE ( 'NONE', *, *, #15042, .F. ) ;
#28398=EDGE_CURVE ( 'NONE', #2267, #1400, #21475, .T. ) ;
#28404=ORIENTED_EDGE ( 'NONE', *, *, #16478, .T. ) ;
#28407=DIRECTION ( 'NONE',  ( -1.101824276508909887E-16, 1.000000000000000000, -0.000000000000000000 ) ) ;
#28415=ORIENTED_EDGE ( 'NONE', *, *, #6149, .F. ) ;
#28417=ORIENTED_EDGE ( 'NONE', *, *, #894, .T. ) ;
#28418=CARTESIAN_POINT ( 'NONE',  ( 8.698509210239508960, 24.34164230456639544, 47.04930799450051637 ) ) ;
#28419=FACE_OUTER_BOUND ( 'NONE', #27582, .T. ) ;
#28422=CARTESIAN_POINT ( 'NONE',  ( 33.46699938050304013, 29.46183152705961206, 47.04930799450051637 ) ) ;
#28429=CARTESIAN_POINT ( 'NONE',  ( 21.09992658989239089, 24.34164230456639544, 47.04930799450051637 ) ) ;
#28434=VERTEX_POINT ( 'NONE', #17950 ) ;
#28443=VERTEX_POINT ( 'NONE', #3167 ) ;
#28446=EDGE_LOOP ( 'NONE', ( #2910, #21083, #15863, #22730 ) ) ;
#28449=AXIS2_PLACEMENT_3D ( 'NONE', #26424, #4267, #23795 ) ;
#28452=ADVANCED_FACE ( 'NONE', ( #10098 ), #19397, .T. ) ;
#28453=ORIENTED_EDGE ( 'NONE', *, *, #15558, .T. ) ;
#28454=CARTESIAN_POINT ( 'NONE',  ( 21.09992658989238734, 38.56284415653841791, 47.04930799450051637 ) ) ;
#28456=CARTESIAN_POINT ( 'NONE',  ( 33.50134396954518223, 32.59164230456639899, 47.04930799450051637 ) ) ;
#28457=CIRCLE ( 'NONE', #21110, 0.1250000000000001110 ) ;
#28458=DIRECTION ( 'NONE',  ( -1.101824276508909887E-16, 1.000000000000000000, -0.000000000000000000 ) ) ;
#28461=EDGE_CURVE ( 'NONE', #16025, #23957, #25694, .T. ) ;
#28463=DIRECTION ( 'NONE',  ( 1.000000000000000000, 0.000000000000000000, 0.000000000000000000 ) ) ;
#28466=DIRECTION ( 'NONE',  ( -1.000000000000000000, 0.000000000000000000, 0.000000000000000000 ) ) ;
#28473=CARTESIAN_POINT ( 'NONE',  ( 21.09992658989238734, 38.56284415653841791, 47.04930799450051637 ) ) ;
#28474=DIRECTION ( 'NONE',  ( -1.101824276508909887E-16, 1.000000000000000000, -0.000000000000000000 ) ) ;
#28477=ORIENTED_EDGE ( 'NONE', *, *, #7576, .T. ) ;
#28479=ORIENTED_EDGE ( 'NONE', *, *, #23439, .T. ) ;
#28481=ADVANCED_FACE ( 'NONE', ( #15018 ), #25018, .T. ) ;
#28482=EDGE_LOOP ( 'NONE', ( #25678, #18348, #11034, #7803 ) ) ;
#28483=AXIS2_PLACEMENT_3D ( 'NONE', #15002, #2363, #27792 ) ;
#28485=ADVANCED_FACE ( 'NONE', ( #27972 ), #27814, .F. ) ;
#28495=DIRECTION ( 'NONE',  ( -1.000000000000000000, 0.000000000000000000, 0.000000000000000000 ) ) ;
#28499=EDGE_CURVE ( 'NONE', #32221, #6908, #18343, .T. ) ;
#28504=EDGE_CURVE ( 'NONE', #3840, #1375, #21200, .T. ) ;
#28508=LINE ( 'NONE', #3226, #15911 ) ;
#28512=AXIS2_PLACEMENT_3D ( 'NONE', #31227, #26935, #31547 ) ;
#28513=ORIENTED_EDGE ( 'NONE', *, *, #6527, .T. ) ;
#28514=AXIS2_PLACEMENT_3D ( 'NONE', #10148, #20467, #7844 ) ;
#28515=DIRECTION ( 'NONE',  ( -1.000000000000000000, 0.000000000000000000, 0.000000000000000000 ) ) ;
#28525=VERTEX_POINT ( 'NONE', #8271 ) ;
#28532=DIRECTION ( 'NONE',  ( -1.000000000000000000, -1.101824276508909887E-16, 0.000000000000000000 ) ) ;
#28540=CARTESIAN_POINT ( 'NONE',  ( 21.09992658989239089, 25.21183152705960140, 47.04930799450051637 ) ) ;
#28545=DIRECTION ( 'NONE',  ( -1.101824276508909887E-16, 1.000000000000000000, -0.000000000000000000 ) ) ;
#28550=CARTESIAN_POINT ( 'NONE',  ( 21.09992658989239089, 24.09143805560860940, 47.04930799450051637 ) ) ;
#28552=FACE_OUTER_BOUND ( 'NONE', #73, .T. ) ;
#28559=CARTESIAN_POINT ( 'NONE',  ( 21.09992658989239089, 24.22145308207319303, 47.04930799450051637 ) ) ;
#28566=CIRCLE ( 'NONE', #24888, 0.1250000000000001110 ) ;
#28575=ORIENTED_EDGE ( 'NONE', *, *, #711, .F. ) ;
#28578=EDGE_CURVE ( 'NONE', #13978, #1940, #20435, .T. ) ;
#28582=EDGE_LOOP ( 'NONE', ( #13008, #8179, #32365, #9733 ) ) ;
#28585=DIRECTION ( 'NONE',  ( -1.000000000000000000, 0.000000000000000000, 0.000000000000000000 ) ) ;
#28586=AXIS2_PLACEMENT_3D ( 'NONE', #4425, #1956, #31999 ) ;
#28587=VERTEX_POINT ( 'NONE', #23686 ) ;
#28588=DIRECTION ( 'NONE',  ( -1.101824276508909887E-16, 1.000000000000000000, -0.000000000000000000 ) ) ;
#28589=ORIENTED_EDGE ( 'NONE', *, *, #521, .F. ) ;
#28594=CIRCLE ( 'NONE', #291, 0.1250000000000001110 ) ;
#28600=CARTESIAN_POINT ( 'NONE',  ( 8.474859994195286461, 29.84184655352422411, 47.04930799450051637 ) ) ;
#28601=VECTOR ( 'NONE', #7925, 1000.000000000000000 ) ;
#28602=FACE_OUTER_BOUND ( 'NONE', #2082, .T. ) ;
#28608=DIRECTION ( 'NONE',  ( -1.000000000000000000, 0.000000000000000000, 0.000000000000000000 ) ) ;
#28611=CARTESIAN_POINT ( 'NONE',  ( 8.474859994195286461, 26.84184655352419568, 47.04930799450051637 ) ) ;
#28612=ADVANCED_FACE ( 'NONE', ( #10059 ), #10711, .T. ) ;
#28614=EDGE_LOOP ( 'NONE', ( #31515, #15791, #31208, #11693 ) ) ;
#28617=EDGE_CURVE ( 'NONE', #1121, #32103, #25177, .T. ) ;
#28619=DIRECTION ( 'NONE',  ( -1.000000000000000000, -1.101824276508909887E-16, 0.000000000000000000 ) ) ;
#28623=CARTESIAN_POINT ( 'NONE',  ( 21.09992658989239089, 23.84143805560861296, 47.04930799450051637 ) ) ;
#28626=VERTEX_POINT ( 'NONE', #5294 ) ;
#28628=DIRECTION ( 'NONE',  ( -1.101824276508909887E-16, 1.000000000000000000, -0.000000000000000000 ) ) ;
#28631=ORIENTED_EDGE ( 'NONE', *, *, #16744, .F. ) ;
#28632=ORIENTED_EDGE ( 'NONE', *, *, #9538, .F. ) ;
#28635=ORIENTED_EDGE ( 'NONE', *, *, #9064, .T. ) ;
#28642=ORIENTED_EDGE ( 'NONE', *, *, #20637, .F. ) ;
#28646=CARTESIAN_POINT ( 'NONE',  ( 21.09992658989238734, 30.84164230456639544, 47.04930799450051637 ) ) ;
#28647=DIRECTION ( 'NONE',  ( -1.224646799147353207E-16, -1.349345573449484691E-32, 1.000000000000000000 ) ) ;
#28649=ORIENTED_EDGE ( 'NONE', *, *, #10730, .T. ) ;
#28650=DIRECTION ( 'NONE',  ( -1.000000000000000000, 0.000000000000000000, 0.000000000000000000 ) ) ;
#28653=CIRCLE ( 'NONE', #22341, 12.36707279061065279 ) ;
#28657=DIRECTION ( 'NONE',  ( -1.000000000000000000, 0.000000000000000000, 0.000000000000000000 ) ) ;
#28662=CARTESIAN_POINT ( 'NONE',  ( 21.09992658989239089, 23.65414230456639544, 47.04930799450051637 ) ) ;
#28680=DIRECTION ( 'NONE',  ( -1.224646799147353207E-16, -1.349345573449484691E-32, 1.000000000000000000 ) ) ;
#28681=DIRECTION ( 'NONE',  ( -1.224646799147353207E-16, -1.349345573449484691E-32, 1.000000000000000000 ) ) ;
#28688=ORIENTED_EDGE ( 'NONE', *, *, #15526, .T. ) ;
#28689=CARTESIAN_POINT ( 'NONE',  ( 8.698509210239581790, 31.84164230456639544, 47.04930799450051637 ) ) ;
#28691=DIRECTION ( 'NONE',  ( -1.101824276508909887E-16, 1.000000000000000000, -0.000000000000000000 ) ) ;
#28694=FACE_OUTER_BOUND ( 'NONE', #31201, .T. ) ;
#28695=ORIENTED_EDGE ( 'NONE', *, *, #23612, .T. ) ;
#28698=CIRCLE ( 'NONE', #32362, 0.1250000000000001110 ) ;
#28702=DIRECTION ( 'NONE',  ( -1.101824276508909887E-16, 1.000000000000000000, -0.000000000000000000 ) ) ;
#28705=AXIS2_PLACEMENT_3D ( 'NONE', #29105, #32381, #6618 ) ;
#28706=ADVANCED_FACE ( 'NONE', ( #20054 ), #31971, .T. ) ;
#28710=EDGE_CURVE ( 'NONE', #4802, #1140, #3657, .T. ) ;
#28715=ORIENTED_EDGE ( 'NONE', *, *, #1294, .T. ) ;
#28718=CARTESIAN_POINT ( 'NONE',  ( 21.09992658989239089, 26.96664230456639899, 47.04930799450051637 ) ) ;
#28720=AXIS2_PLACEMENT_3D ( 'NONE', #16006, #31116, #27842 ) ;
#28722=AXIS2_PLACEMENT_3D ( 'NONE', #19891, #29430, #11866 ) ;
#28725=CIRCLE ( 'NONE', #22955, 0.1250000000000001110 ) ;
#28726=CARTESIAN_POINT ( 'NONE',  ( 21.09992658989239089, 23.59164230456639544, 47.04930799450051637 ) ) ;
#28729=DIRECTION ( 'NONE',  ( -1.101824276508909887E-16, 1.000000000000000000, -0.000000000000000000 ) ) ;
#28735=SURFACE_SIDE_STYLE ('',( #25787 ) ) ;
#28737=EDGE_LOOP ( 'NONE', ( #28323, #21676, #21980, #7541 ) ) ;
#28738=LINE ( 'NONE', #11029, #27058 ) ;
#28739=FACE_OUTER_BOUND ( 'NONE', #9425, .T. ) ;
#28741=CARTESIAN_POINT ( 'NONE',  ( 33.71785032049137243, 25.21664230456640254, 47.04930799450051637 ) ) ;
#28742=FACE_OUTER_BOUND ( 'NONE', #4003, .T. ) ;
#28743=VERTEX_POINT ( 'NONE', #1477 ) ;
#28746=AXIS2_PLACEMENT_3D ( 'NONE', #13032, #7460, #15006 ) ;
#28749=CARTESIAN_POINT ( 'NONE',  ( 33.50134396954523908, 27.84164230456639544, 47.04930799450051637 ) ) ;
#28751=AXIS2_PLACEMENT_3D ( 'NONE', #2396, #10112, #32107 ) ;
#28753=TOROIDAL_SURFACE ( 'NONE', #8839, 12.40141737965287305, 0.1250000000000000833 ) ;
#28755=ADVANCED_FACE ( 'NONE', ( #1002 ), #16092, .F. ) ;
#28757=DIRECTION ( 'NONE',  ( -1.101824276508909887E-16, 1.000000000000000000, -0.000000000000000000 ) ) ;
#28761=CYLINDRICAL_SURFACE ( 'NONE', #4097, 12.36707279061065101 ) ;
#28762=AXIS2_PLACEMENT_3D ( 'NONE', #26051, #28680, #3733 ) ;
#28775=DIRECTION ( 'NONE',  ( -1.000000000000000000, -1.101824276508909887E-16, 0.000000000000000000 ) ) ;
#28782=CARTESIAN_POINT ( 'NONE',  ( 21.09992658989239089, 30.46664230456641675, 47.04930799450051637 ) ) ;
#28790=ORIENTED_EDGE ( 'NONE', *, *, #23114, .F. ) ;
#28791=CIRCLE ( 'NONE', #13591, 0.1249999999999931721 ) ;
#28796=ADVANCED_FACE ( 'NONE', ( #26275 ), #26766, .T. ) ;
#28803=CYLINDRICAL_SURFACE ( 'NONE', #8199, 12.62506659569710266 ) ;
#28817=CARTESIAN_POINT ( 'NONE',  ( 8.590256034766447613, 23.65414230456639544, 47.04930799450051637 ) ) ;
#28818=DIRECTION ( 'NONE',  ( -1.000000000000000000, 0.000000000000000000, 0.000000000000000000 ) ) ;
#28823=DIRECTION ( 'NONE',  ( -1.000000000000000000, -1.101824276508909887E-16, 0.000000000000000000 ) ) ;
#28826=DIRECTION ( 'NONE',  ( -1.000000000000000000, 0.000000000000000000, 0.000000000000000000 ) ) ;
#28828=VERTEX_POINT ( 'NONE', #28422 ) ;
#28831=AXIS2_PLACEMENT_3D ( 'NONE', #14569, #29339, #30003 ) ;
#28836=ORIENTED_EDGE ( 'NONE', *, *, #11365, .F. ) ;
#28839=EDGE_LOOP ( 'NONE', ( #21864, #12395, #13316, #951 ) ) ;
#28840=AXIS2_PLACEMENT_3D ( 'NONE', #11514, #22001, #19542 ) ;
#28841=EDGE_CURVE ( 'NONE', #27647, #20897, #5805, .T. ) ;
#28842=AXIS2_PLACEMENT_3D ( 'NONE', #15937, #25944, #22996 ) ;
#28843=ORIENTED_EDGE ( 'NONE', *, *, #10274, .F. ) ;
#28844=DIRECTION ( 'NONE',  ( -1.101824276508909887E-16, 1.000000000000000000, -0.000000000000000000 ) ) ;
#28845=AXIS2_PLACEMENT_3D ( 'NONE', #15699, #25719, #13261 ) ;
#28847=EDGE_LOOP ( 'NONE', ( #7645, #24775, #12025, #26672 ) ) ;
#28848=FACE_OUTER_BOUND ( 'NONE', #23384, .T. ) ;
#28849=DIRECTION ( 'NONE',  ( -1.000000000000000000, 0.000000000000000000, 0.000000000000000000 ) ) ;
#28854=AXIS2_PLACEMENT_3D ( 'NONE', #12269, #9963, #15211 ) ;
#28855=VECTOR ( 'NONE', #31340, 1000.000000000000000 ) ;
#28858=CARTESIAN_POINT ( 'NONE',  ( 21.09992658989238734, 30.96183152705961206, 47.04930799450051637 ) ) ;
#28860=DIRECTION ( 'NONE',  ( -1.000000000000000000, 0.000000000000000000, 0.000000000000000000 ) ) ;
#28861=EDGE_CURVE ( 'NONE', #21198, #28587, #544, .T. ) ;
#28867=DIRECTION ( 'NONE',  ( -1.101824276508909887E-16, 1.000000000000000000, -0.000000000000000000 ) ) ;
#28870=DIRECTION ( 'NONE',  ( -1.101824276508909887E-16, 1.000000000000000000, -0.000000000000000000 ) ) ;
#28872=ADVANCED_FACE ( 'NONE', ( #29555 ), #28352, .T. ) ;
#28873=CIRCLE ( 'NONE', #13156, 12.36707279061065101 ) ;
#28874=DIRECTION ( 'NONE',  ( -1.101824276508909887E-16, 1.000000000000000000, -0.000000000000000000 ) ) ;
#28876=DIRECTION ( 'NONE',  ( -1.101824276508909887E-16, 1.000000000000000000, -0.000000000000000000 ) ) ;
#28877=CARTESIAN_POINT ( 'NONE',  ( 21.09992658989238734, 38.56284415653841791, 47.04930799450051637 ) ) ;
#28883=AXIS2_PLACEMENT_3D ( 'NONE', #11415, #6333, #8642 ) ;
#28884=ORIENTED_EDGE ( 'NONE', *, *, #31023, .F. ) ;
#28889=EDGE_LOOP ( 'NONE', ( #28930, #3884, #1414, #21708 ) ) ;
#28890=DIRECTION ( 'NONE',  ( -1.101824276508909887E-16, 1.000000000000000000, -0.000000000000000000 ) ) ;
#28898=ADVANCED_FACE ( 'NONE', ( #29713 ), #15758, .T. ) ;
#28901=ORIENTED_EDGE ( 'NONE', *, *, #5121, .F. ) ;
#28905=DIRECTION ( 'NONE',  ( -1.000000000000000000, -1.101824276508909887E-16, 0.000000000000000000 ) ) ;
#28908=EDGE_LOOP ( 'NONE', ( #18465, #23013, #32419, #18014 ) ) ;
#28910=CIRCLE ( 'NONE', #1649, 12.62506659569710266 ) ;
#28913=EDGE_CURVE ( 'NONE', #15199, #31427, #9199, .T. ) ;
#28920=CARTESIAN_POINT ( 'NONE',  ( 33.62240545574881878, 32.54735957529758394, 47.04930799450051637 ) ) ;
#28923=FACE_OUTER_BOUND ( 'NONE', #21021, .T. ) ;
#28924=ORIENTED_EDGE ( 'NONE', *, *, #11629, .T. ) ;
#28926=DIRECTION ( 'NONE',  ( -1.000000000000000000, 0.000000000000000000, 0.000000000000000000 ) ) ;
#28930=ORIENTED_EDGE ( 'NONE', *, *, #12349, .F. ) ;
#28933=EDGE_CURVE ( 'NONE', #25766, #893, #15243, .T. ) ;
#28934=CIRCLE ( 'NONE', #23173, 0.1250000000000001110 ) ;
#28937=DIRECTION ( 'NONE',  ( -1.000000000000000000, 0.000000000000000000, 0.000000000000000000 ) ) ;
#28942=CARTESIAN_POINT ( 'NONE',  ( 21.09992658989238734, 32.09164230456639899, 47.04930799450051637 ) ) ;
#28948=ADVANCED_FACE ( 'NONE', ( #9034 ), #8932, .T. ) ;
#28951=AXIS2_PLACEMENT_3D ( 'NONE', #17359, #27381, #20145 ) ;
#28956=CARTESIAN_POINT ( 'NONE',  ( 33.71785032049129427, 32.46664230456639899, 47.04930799450051637 ) ) ;
#28959=CARTESIAN_POINT ( 'NONE',  ( 21.09992658989239089, 28.22145308207318237, 47.04930799450051637 ) ) ;
#28967=DIRECTION ( 'NONE',  ( -1.101824276508909887E-16, 1.000000000000000000, -0.000000000000000000 ) ) ;
#28968=CARTESIAN_POINT ( 'NONE',  ( 21.09992658989238734, 38.56284415653841791, 47.04930799450051637 ) ) ;
#28975=CARTESIAN_POINT ( 'NONE',  ( 21.09992658989238734, 32.59164230456639899, 47.04930799450051637 ) ) ;
#28976=CARTESIAN_POINT ( 'NONE',  ( 33.72499318558949000, 38.56284415653841791, 47.04930799450051637 ) ) ;
#28982=CARTESIAN_POINT ( 'NONE',  ( 21.09992658989239089, 27.47145308207318593, 47.04930799450051637 ) ) ;
#28983=CARTESIAN_POINT ( 'NONE',  ( 21.09992658989239089, 28.34184655352419213, 47.04930799450051637 ) ) ;
#28986=VECTOR ( 'NONE', #12611, 1000.000000000000000 ) ;
#28987=FACE_OUTER_BOUND ( 'NONE', #13340, .T. ) ;
#28993=EDGE_LOOP ( 'NONE', ( #582, #1004, #28477, #27511 ) ) ;
#28995=CARTESIAN_POINT ( 'NONE',  ( 21.09992658989239089, 28.59143805560861296, 47.04930799450051637 ) ) ;
#28996=VERTEX_POINT ( 'NONE', #22316 ) ;
#29001=AXIS2_PLACEMENT_3D ( 'NONE', #28983, #14052, #6659 ) ;
#29004=EDGE_CURVE ( 'NONE', #31841, #16102, #2785, .T. ) ;
#29006=DIRECTION ( 'NONE',  ( -1.000000000000000000, -1.101824276508909764E-16, 0.000000000000000000 ) ) ;
#29007=CIRCLE ( 'NONE', #7005, 0.1249999999999983763 ) ;
#29014=LINE ( 'NONE', #11618, #13768 ) ;
#29015=ORIENTED_EDGE ( 'NONE', *, *, #2118, .T. ) ;
#29017=DIRECTION ( 'NONE',  ( -1.101824276508909887E-16, 1.000000000000000000, -0.000000000000000000 ) ) ;
#29018=DIRECTION ( 'NONE',  ( -1.101824276508909887E-16, 1.000000000000000000, -0.000000000000000000 ) ) ;
#29032=FACE_OUTER_BOUND ( 'NONE', #30485, .T. ) ;
#29033=CIRCLE ( 'NONE', #28216, 12.36707279061065101 ) ;
#29036=ORIENTED_EDGE ( 'NONE', *, *, #24308, .F. ) ;
#29039=CIRCLE ( 'NONE', #20123, 0.1250000000000001110 ) ;
#29043=EDGE_CURVE ( 'NONE', #593, #4576, #16798, .T. ) ;
#29044=CARTESIAN_POINT ( 'NONE',  ( 33.46699938050303302, 38.56284415653841791, 47.04930799450051637 ) ) ;
#29051=AXIS2_PLACEMENT_3D ( 'NONE', #27182, #9961, #14889 ) ;
#29053=LINE ( 'NONE', #14121, #14800 ) ;
#29057=DIRECTION ( 'NONE',  ( 1.000000000000000000, 0.000000000000000000, 0.000000000000000000 ) ) ;
#29061=ORIENTED_EDGE ( 'NONE', *, *, #4217, .F. ) ;
#29064=EDGE_LOOP ( 'NONE', ( #26754, #4333, #20866, #5263 ) ) ;
#29070=DIRECTION ( 'NONE',  ( -1.000000000000000000, 0.000000000000000000, 0.000000000000000000 ) ) ;
#29073=CIRCLE ( 'NONE', #781, 0.1250000000000001110 ) ;
#29074=CIRCLE ( 'NONE', #13875, 12.62506659569710266 ) ;
#29078=ORIENTED_EDGE ( 'NONE', *, *, #3807, .F. ) ;
#29079=CARTESIAN_POINT ( 'NONE',  ( 21.09992658989238734, 31.84164230456639544, 47.04930799450051637 ) ) ;
#29086=EDGE_CURVE ( 'NONE', #2250, #4802, #478, .T. ) ;
#29088=DIRECTION ( 'NONE',  ( -1.101824276508909887E-16, 1.000000000000000000, -0.000000000000000000 ) ) ;
#29089=CARTESIAN_POINT ( 'NONE',  ( 21.09992658989239089, 27.84164230456639544, 47.04930799450051637 ) ) ;
#29094=TOROIDAL_SURFACE ( 'NONE', #21755, 12.40141737965284641, 0.1249999999999995698 ) ;
#29105=CARTESIAN_POINT ( 'NONE',  ( 33.50134396954520355, 30.59164230456639544, 47.04930799450051637 ) ) ;
#29107=DIRECTION ( 'NONE',  ( -1.101824276508909887E-16, 1.000000000000000000, -0.000000000000000000 ) ) ;
#29108=ORIENTED_EDGE ( 'NONE', *, *, #2811, .T. ) ;
#29113=DIRECTION ( 'NONE',  ( -1.224646799147353207E-16, -1.349345573449484691E-32, 1.000000000000000000 ) ) ;
#29114=CARTESIAN_POINT ( 'NONE',  ( 21.09992658989239089, 30.09164230456639544, 47.04930799450051637 ) ) ;
#29117=ORIENTED_EDGE ( 'NONE', *, *, #5574, .F. ) ;
#29121=ADVANCED_FACE ( 'NONE', ( #27734 ), #26218, .T. ) ;
#29127=AXIS2_PLACEMENT_3D ( 'NONE', #19553, #7091, #27110 ) ;
#29131=DIRECTION ( 'NONE',  ( 1.000000000000000000, 0.000000000000000000, 0.000000000000000000 ) ) ;
#29132=AXIS2_PLACEMENT_3D ( 'NONE', #18059, #25456, #2958 ) ;
#29136=DIRECTION ( 'NONE',  ( -1.000000000000000000, 0.000000000000000000, 0.000000000000000000 ) ) ;
#29140=DIRECTION ( 'NONE',  ( -1.101824276508909887E-16, 1.000000000000000000, -0.000000000000000000 ) ) ;
#29142=ORIENTED_EDGE ( 'NONE', *, *, #14168, .T. ) ;
#29145=CARTESIAN_POINT ( 'NONE',  ( 21.09992658989238734, 32.34164230456639899, 47.04930799450051637 ) ) ;
#29146=DIRECTION ( 'NONE',  ( -1.224646799147353207E-16, -1.349345573449484691E-32, 1.000000000000000000 ) ) ;
#29147=CARTESIAN_POINT ( 'NONE',  ( 8.698509210239508960, 24.34164230456639544, 47.04930799450051637 ) ) ;
#29154=DIRECTION ( 'NONE',  ( -1.000000000000000000, 0.000000000000000000, 0.000000000000000000 ) ) ;
#29163=CIRCLE ( 'NONE', #3481, 12.27641737965281621 ) ;
#29167=CARTESIAN_POINT ( 'NONE',  ( 21.09992658989239089, 28.09184655352419213, 47.04930799450051637 ) ) ;
#29169=CARTESIAN_POINT ( 'NONE',  ( 8.698509210239587119, 32.34164230456639899, 47.04930799450051637 ) ) ;
#29172=DIRECTION ( 'NONE',  ( -1.224646799147353207E-16, -1.349345573449484691E-32, 1.000000000000000000 ) ) ;
#29176=FACE_OUTER_BOUND ( 'NONE', #32145, .T. ) ;
#29181=CARTESIAN_POINT ( 'NONE',  ( 33.71785032049135822, 26.71664230456639899, 47.04930799450051637 ) ) ;
#29193=VERTEX_POINT ( 'NONE', #18190 ) ;
#29194=CARTESIAN_POINT ( 'NONE',  ( 21.09992658989238734, 38.56284415653841791, 47.04930799450051637 ) ) ;
#29199=EDGE_CURVE ( 'NONE', #24404, #4539, #27847, .T. ) ;
#29207=CARTESIAN_POINT ( 'NONE',  ( 8.732853799281738105, 25.96183152705960140, 47.04930799450051637 ) ) ;
#29210=AXIS2_PLACEMENT_3D ( 'NONE', #1752, #21438, #1910 ) ;
#29212=DIRECTION ( 'NONE',  ( -1.000000000000000000, 0.000000000000000000, 0.000000000000000000 ) ) ;
#29216=CARTESIAN_POINT ( 'NONE',  ( 21.09992658989238734, 38.56284415653841791, 47.04930799450051637 ) ) ;
#29217=CARTESIAN_POINT ( 'NONE',  ( 21.09992658989238734, 38.56284415653841791, 47.04930799450051637 ) ) ;
#29220=VERTEX_POINT ( 'NONE', #807 ) ;
#29223=DIRECTION ( 'NONE',  ( -1.101824276508909887E-16, 1.000000000000000000, -0.000000000000000000 ) ) ;
#29229=VERTEX_POINT ( 'NONE', #10832 ) ;
#29236=EDGE_LOOP ( 'NONE', ( #4286, #17121, #31797, #27719 ) ) ;
#29238=DIRECTION ( 'NONE',  ( -1.000000000000000000, 0.000000000000000000, 0.000000000000000000 ) ) ;
#29242=ORIENTED_EDGE ( 'NONE', *, *, #22196, .F. ) ;
#29250=EDGE_CURVE ( 'NONE', #21573, #9948, #18392, .T. ) ;
#29256=AXIS2_PLACEMENT_3D ( 'NONE', #26826, #8940, #29131 ) ;
#29258=EDGE_CURVE ( 'NONE', #13589, #24454, #28384, .T. ) ;
#29267=ORIENTED_EDGE ( 'NONE', *, *, #16076, .F. ) ;
#29273=CARTESIAN_POINT ( 'NONE',  ( 33.72499318558949710, 25.09143805560860940, 47.04930799450051637 ) ) ;
#29274=CIRCLE ( 'NONE', #5680, 12.36707279061065101 ) ;
#29278=ORIENTED_EDGE ( 'NONE', *, *, #18289, .T. ) ;
#29279=EDGE_LOOP ( 'NONE', ( #13078, #20298, #14734, #17669 ) ) ;
#29283=AXIS2_PLACEMENT_3D ( 'NONE', #21307, #8212, #3763 ) ;
#29286=DIRECTION ( 'NONE',  ( -1.101824276508909887E-16, 1.000000000000000000, -0.000000000000000000 ) ) ;
#29288=ORIENTED_EDGE ( 'NONE', *, *, #12736, .F. ) ;
#29289=AXIS2_PLACEMENT_3D ( 'NONE', #10383, #25636, #20378 ) ;
#29294=CARTESIAN_POINT ( 'NONE',  ( 33.71785032049136532, 25.96664230456639899, 47.04930799450051637 ) ) ;
#29296=EDGE_LOOP ( 'NONE', ( #4776, #31747, #3189, #11828 ) ) ;
#29299=CARTESIAN_POINT ( 'NONE',  ( 21.09992658989238734, 38.56284415653841791, 47.04930799450051637 ) ) ;
#29301=DIRECTION ( 'NONE',  ( -1.224646799147353207E-16, -1.349345573449484691E-32, 1.000000000000000000 ) ) ;
#29303=CARTESIAN_POINT ( 'NONE',  ( 21.09992658989239089, 23.71183152705959429, 47.04930799450051637 ) ) ;
#29306=DIRECTION ( 'NONE',  ( -1.101824276508909887E-16, 1.000000000000000000, -0.000000000000000000 ) ) ;
#29308=DIRECTION ( 'NONE',  ( -1.000000000000000000, -1.101824276508909887E-16, 0.000000000000000000 ) ) ;
#29309=CIRCLE ( 'NONE', #22483, 12.36707279061065279 ) ;
#29314=ORIENTED_EDGE ( 'NONE', *, *, #2803, .T. ) ;
#29321=AXIS2_PLACEMENT_3D ( 'NONE', #27988, #15349, #23051 ) ;
#29330=VERTEX_POINT ( 'NONE', #18994 ) ;
#29332=ORIENTED_EDGE ( 'NONE', *, *, #19097, .F. ) ;
#29337=CIRCLE ( 'NONE', #31428, 12.27641737965281266 ) ;
#29339=DIRECTION ( 'NONE',  ( -1.101824276508909887E-16, 1.000000000000000000, -0.000000000000000000 ) ) ;
#29345=LINE ( 'NONE', #29679, #26905 ) ;
#29347=CARTESIAN_POINT ( 'NONE',  ( 8.732853799281734553, 38.56284415653841791, 47.04930799450051637 ) ) ;
#29353=EDGE_CURVE ( 'NONE', #20430, #21925, #27695, .T. ) ;
#29358=DIRECTION ( 'NONE',  ( -1.000000000000000000, 0.000000000000000000, 0.000000000000000000 ) ) ;
#29360=AXIS2_PLACEMENT_3D ( 'NONE', #28456, #5642, #5974 ) ;
#29364=AXIS2_PLACEMENT_3D ( 'NONE', #13366, #1037, #23996 ) ;
#29368=VECTOR ( 'NONE', #5954, 1000.000000000000000 ) ;
#29374=DIRECTION ( 'NONE',  ( -1.101824276508909887E-16, 1.000000000000000000, -0.000000000000000000 ) ) ;
#29375=CARTESIAN_POINT ( 'NONE',  ( 8.474859994195286461, 27.59143805560860940, 47.04930799450051637 ) ) ;
#29377=ORIENTED_EDGE ( 'NONE', *, *, #1420, .T. ) ;
#29378=CARTESIAN_POINT ( 'NONE',  ( 33.46699938050304013, 27.97145308207318237, 47.04930799450050927 ) ) ;
#29379=CIRCLE ( 'NONE', #26752, 0.1250000000000001110 ) ;
#29385=ORIENTED_EDGE ( 'NONE', *, *, #26627, .T. ) ;
#29392=CARTESIAN_POINT ( 'NONE',  ( 21.09992658989238734, 38.56284415653841791, 47.04930799450051637 ) ) ;
#29398=DIRECTION ( 'NONE',  ( -1.101824276508909887E-16, 1.000000000000000000, -0.000000000000000000 ) ) ;
#29400=ORIENTED_EDGE ( 'NONE', *, *, #24678, .F. ) ;
#29408=DIRECTION ( 'NONE',  ( -1.000000000000000000, -1.101824276508909887E-16, 0.000000000000000000 ) ) ;
#29414=DIRECTION ( 'NONE',  ( -1.000000000000000000, 0.000000000000000000, 0.000000000000000000 ) ) ;
#29415=DIRECTION ( 'NONE',  ( -1.101824276508909887E-16, 1.000000000000000000, -0.000000000000000000 ) ) ;
#29416=VECTOR ( 'NONE', #5488, 1000.000000000000000 ) ;
#29420=CARTESIAN_POINT ( 'NONE',  ( 8.474859994195286461, 29.59184655352418858, 47.04930799450051637 ) ) ;
#29422=DIRECTION ( 'NONE',  ( -1.101824276508909887E-16, 1.000000000000000000, -0.000000000000000000 ) ) ;
#29430=DIRECTION ( 'NONE',  ( -1.101824276508909887E-16, 1.000000000000000000, -0.000000000000000000 ) ) ;
#29433=CARTESIAN_POINT ( 'NONE',  ( 21.09992658989238734, 38.56284415653841791, 47.04930799450051637 ) ) ;
#29437=CYLINDRICAL_SURFACE ( 'NONE', #25273, 12.62506659569710266 ) ;
#29440=ORIENTED_EDGE ( 'NONE', *, *, #25932, .T. ) ;
#29447=ORIENTED_EDGE ( 'NONE', *, *, #23578, .T. ) ;
#29449=TOROIDAL_SURFACE ( 'NONE', #25763, 12.40141737965280200, 0.1249999999999999445 ) ;
#29454=AXIS2_PLACEMENT_3D ( 'NONE', #26673, #6019, #20940 ) ;
#29456=ORIENTED_EDGE ( 'NONE', *, *, #5, .T. ) ;
#29460=EDGE_CURVE ( 'NONE', #2537, #12300, #19451, .T. ) ;
#29465=CARTESIAN_POINT ( 'NONE',  ( 21.09992658989238734, 38.56284415653841791, 47.04930799450051637 ) ) ;
#29476=EDGE_LOOP ( 'NONE', ( #31622, #26340, #17300, #15785 ) ) ;
#29483=CARTESIAN_POINT ( 'NONE',  ( 33.71785032049136532, 25.71664230456640254, 47.04930799450051637 ) ) ;
#29490=AXIS2_PLACEMENT_3D ( 'NONE', #21949, #16701, #1781 ) ;
#29495=EDGE_CURVE ( 'NONE', #3554, #16793, #30464, .T. ) ;
#29496=ADVANCED_FACE ( 'NONE', ( #6025 ), #30655, .T. ) ;
#29500=EDGE_CURVE ( 'NONE', #22128, #30310, #26252, .T. ) ;
#29505=AXIS2_PLACEMENT_3D ( 'NONE', #22458, #5077, #24773 ) ;
#29514=CARTESIAN_POINT ( 'NONE',  ( 8.732853799281732776, 31.71183152705962272, 47.04930799450051637 ) ) ;
#29520=EDGE_LOOP ( 'NONE', ( #23012, #16077, #14871, #2029 ) ) ;
#29524=DIRECTION ( 'NONE',  ( -1.000000000000000000, 0.000000000000000000, 0.000000000000000000 ) ) ;
#29526=DIRECTION ( 'NONE',  ( 1.000000000000000000, 0.000000000000000000, 0.000000000000000000 ) ) ;
#29529=DIRECTION ( 'NONE',  ( -1.101824276508909887E-16, 1.000000000000000000, -0.000000000000000000 ) ) ;
#29531=AXIS2_PLACEMENT_3D ( 'NONE', #611, #22922, #20628 ) ;
#29541=EDGE_CURVE ( 'NONE', #12341, #7948, #5698, .T. ) ;
#29542=ORIENTED_EDGE ( 'NONE', *, *, #17249, .T. ) ;
#29543=EDGE_CURVE ( 'NONE', #13543, #22868, #10569, .T. ) ;
#29544=DIRECTION ( 'NONE',  ( -1.101824276508909887E-16, 1.000000000000000000, -0.000000000000000000 ) ) ;
#29548=ORIENTED_EDGE ( 'NONE', *, *, #10892, .F. ) ;
#29552=CARTESIAN_POINT ( 'NONE',  ( 8.474859994195282908, 38.56284415653841791, 47.04930799450051637 ) ) ;
#29553=FACE_OUTER_BOUND ( 'NONE', #4433, .T. ) ;
#29555=FACE_OUTER_BOUND ( 'NONE', #5238, .T. ) ;
#29557=EDGE_LOOP ( 'NONE', ( #22512, #20349, #27069, #14968 ) ) ;
#29558=EDGE_LOOP ( 'NONE', ( #6614, #31441, #7571, #9130 ) ) ;
#29559=DIRECTION ( 'NONE',  ( -1.000000000000000000, 0.000000000000000000, 0.000000000000000000 ) ) ;
#29561=CIRCLE ( 'NONE', #1753, 0.1249999999999966416 ) ;
#29562=DIRECTION ( 'NONE',  ( -1.101824276508909887E-16, 1.000000000000000000, -0.000000000000000000 ) ) ;
#29564=CIRCLE ( 'NONE', #15404, 0.1250000000000001110 ) ;
#29572=AXIS2_PLACEMENT_3D ( 'NONE', #21195, #31235, #29414 ) ;
#29577=EDGE_CURVE ( 'NONE', #32221, #5223, #22072, .T. ) ;
#29579=EDGE_CURVE ( 'NONE', #11099, #14523, #4274, .T. ) ;
#29581=DIRECTION ( 'NONE',  ( -1.000000000000000000, 0.000000000000000000, 0.000000000000000000 ) ) ;
#29588=CARTESIAN_POINT ( 'NONE',  ( 8.698509210239544487, 27.84164230456639544, 47.04930799450051637 ) ) ;
#29594=AXIS2_PLACEMENT_3D ( 'NONE', #23680, #31873, #6760 ) ;
#29599=AXIS2_PLACEMENT_3D ( 'NONE', #14289, #24612, #19352 ) ;
#29603=AXIS2_PLACEMENT_3D ( 'NONE', #28171, #13252, #20281 ) ;
#29610=DIRECTION ( 'NONE',  ( -1.000000000000000000, 0.000000000000000000, 0.000000000000000000 ) ) ;
#29619=CARTESIAN_POINT ( 'NONE',  ( 8.732853799281732776, 30.96183152705961206, 47.04930799450051637 ) ) ;
#29627=CIRCLE ( 'NONE', #32255, 12.62506659569710443 ) ;
#29628=FACE_OUTER_BOUND ( 'NONE', #25176, .T. ) ;
#29629=( NAMED_UNIT ( * ) PLANE_ANGLE_UNIT ( ) SI_UNIT ( $, .RADIAN. ) );
#29636=CARTESIAN_POINT ( 'NONE',  ( 33.72499318558949710, 27.84143805560860940, 47.04930799450051637 ) ) ;
#29642=CARTESIAN_POINT ( 'NONE',  ( 8.732853799281734553, 28.97145308207318237, 47.04930799450051637 ) ) ;
#29643=DIRECTION ( 'NONE',  ( -1.000000000000000000, 0.000000000000000000, 0.000000000000000000 ) ) ;
#29646=VERTEX_POINT ( 'NONE', #10953 ) ;
#29652=ORIENTED_EDGE ( 'NONE', *, *, #18212, .T. ) ;
#29653=AXIS2_PLACEMENT_3D ( 'NONE', #7380, #27397, #14923 ) ;
#29663=FACE_OUTER_BOUND ( 'NONE', #9531, .T. ) ;
#29675=CARTESIAN_POINT ( 'NONE',  ( 33.46699938050302592, 32.22145308207317527, 47.04930799450050927 ) ) ;
#29676=LINE ( 'NONE', #12774, #28986 ) ;
#29679=CARTESIAN_POINT ( 'NONE',  ( 33.46699938050303302, 38.56284415653841791, 47.04930799450051637 ) ) ;
#29681=ORIENTED_EDGE ( 'NONE', *, *, #31212, .F. ) ;
#29683=CARTESIAN_POINT ( 'NONE',  ( 33.71785032049097453, 31.21664230456641675, 47.04930799450051637 ) ) ;
#29684=EDGE_CURVE ( 'NONE', #17205, #17361, #5345, .T. ) ;
#29685=AXIS2_PLACEMENT_3D ( 'NONE', #1874, #14361, #6478 ) ;
#29688=ORIENTED_EDGE ( 'NONE', *, *, #11481, .F. ) ;
#29691=EDGE_CURVE ( 'NONE', #7282, #2007, #24184, .T. ) ;
#29696=ORIENTED_EDGE ( 'NONE', *, *, #32480, .T. ) ;
#29699=FACE_OUTER_BOUND ( 'NONE', #5074, .T. ) ;
#29700=AXIS2_PLACEMENT_3D ( 'NONE', #5476, #27956, #30424 ) ;
#29701=ORIENTED_EDGE ( 'NONE', *, *, #20379, .F. ) ;
#29702=DIRECTION ( 'NONE',  ( -1.000000000000000000, -1.101824276508910010E-16, 0.000000000000000000 ) ) ;
#29707=ORIENTED_EDGE ( 'NONE', *, *, #21170, .F. ) ;
#29713=FACE_OUTER_BOUND ( 'NONE', #19594, .T. ) ;
#29719=AXIS2_PLACEMENT_3D ( 'NONE', #18357, #28387, #5906 ) ;
#29720=DIRECTION ( 'NONE',  ( -1.000000000000000000, 0.000000000000000000, 0.000000000000000000 ) ) ;
#29721=ADVANCED_FACE ( 'NONE', ( #16980 ), #13196, .T. ) ;
#29732=EDGE_CURVE ( 'NONE', #9593, #30342, #26274, .T. ) ;
#29737=CARTESIAN_POINT ( 'NONE',  ( 21.09992658989239089, 29.59164230456639899, 47.04930799450051637 ) ) ;
#29741=CARTESIAN_POINT ( 'NONE',  ( 21.09992658989239089, 29.09143805560861296, 47.04930799450051637 ) ) ;
#29745=DIRECTION ( 'NONE',  ( -1.000000000000000000, -1.101824276508909887E-16, 0.000000000000000000 ) ) ;
#29750=DIRECTION ( 'NONE',  ( 0.000000000000000000, -0.000000000000000000, -1.000000000000000000 ) ) ;
#29752=ORIENTED_EDGE ( 'NONE', *, *, #12275, .T. ) ;
#29754=DIRECTION ( 'NONE',  ( -1.000000000000000000, 0.000000000000000000, 0.000000000000000000 ) ) ;
#29758=ORIENTED_EDGE ( 'NONE', *, *, #519, .F. ) ;
#29759=DIRECTION ( 'NONE',  ( -1.101824276508909887E-16, 1.000000000000000000, -0.000000000000000000 ) ) ;
#29767=AXIS2_PLACEMENT_3D ( 'NONE', #22116, #1612, #4402 ) ;
#29769=CARTESIAN_POINT ( 'NONE',  ( 33.46699938050304013, 27.46183152705960850, 47.04930799450051637 ) ) ;
#29771=DIRECTION ( 'NONE',  ( -1.000000000000000000, 0.000000000000000000, 0.000000000000000000 ) ) ;
#29780=DIRECTION ( 'NONE',  ( -1.101824276508909887E-16, 1.000000000000000000, -0.000000000000000000 ) ) ;
#29781=CIRCLE ( 'NONE', #15625, 12.62506659569710266 ) ;
#29783=ORIENTED_EDGE ( 'NONE', *, *, #30135, .F. ) ;
#29787=DIRECTION ( 'NONE',  ( 1.000000000000000000, 0.000000000000000000, 0.000000000000000000 ) ) ;
#29794=CARTESIAN_POINT ( 'NONE',  ( 33.46699938050304013, 38.56284415653841791, 47.04930799450051637 ) ) ;
#29795=DIRECTION ( 'NONE',  ( -1.000000000000000000, 0.000000000000000000, 0.000000000000000000 ) ) ;
#29796=CARTESIAN_POINT ( 'NONE',  ( 8.698509210239512512, 24.59164230456639544, 47.04930799450051637 ) ) ;
#29797=CARTESIAN_POINT ( 'NONE',  ( 21.09992658989238734, 38.56284415653841791, 47.04930799450051637 ) ) ;
#29800=ORIENTED_EDGE ( 'NONE', *, *, #29577, .F. ) ;
#29803=ORIENTED_EDGE ( 'NONE', *, *, #8269, .F. ) ;
#29806=LINE ( 'NONE', #19944, #31624 ) ;
#29808=EDGE_CURVE ( 'NONE', #13651, #9009, #25254, .T. ) ;
#29809=ORIENTED_EDGE ( 'NONE', *, *, #7611, .T. ) ;
#29812=EDGE_CURVE ( 'NONE', #32455, #2915, #30479, .T. ) ;
#29813=ADVANCED_FACE ( 'NONE', ( #27655 ), #29449, .T. ) ;
#29818=AXIS2_PLACEMENT_3D ( 'NONE', #287, #5549, #8492 ) ;
#29823=VERTEX_POINT ( 'NONE', #30133 ) ;
#29824=CARTESIAN_POINT ( 'NONE',  ( 21.09992658989238734, 38.56284415653841791, 47.04930799450051637 ) ) ;
#29825=DIRECTION ( 'NONE',  ( -1.000000000000000000, -1.101824276508909887E-16, 0.000000000000000000 ) ) ;
#29827=CARTESIAN_POINT ( 'NONE',  ( 21.09992658989238734, 31.84164230456639544, 47.04930799450051637 ) ) ;
#29832=VERTEX_POINT ( 'NONE', #15185 ) ;
#29835=EDGE_LOOP ( 'NONE', ( #21, #3718, #29934, #4611 ) ) ;
#29841=CARTESIAN_POINT ( 'NONE',  ( 8.474859994195281132, 38.56284415653841791, 47.04930799450051637 ) ) ;
#29844=DIRECTION ( 'NONE',  ( -1.000000000000000000, 0.000000000000000000, 0.000000000000000000 ) ) ;
#29845=VERTEX_POINT ( 'NONE', #17142 ) ;
#29851=DIRECTION ( 'NONE',  ( -1.101824276508909887E-16, 1.000000000000000000, -0.000000000000000000 ) ) ;
#29852=EDGE_LOOP ( 'NONE', ( #13710, #11777, #24596, #7044 ) ) ;
#29853=EDGE_CURVE ( 'NONE', #27647, #3840, #11605, .T. ) ;
#29858=VERTEX_POINT ( 'NONE', #17801 ) ;
#29859=TOROIDAL_SURFACE ( 'NONE', #17253, 12.61792373059896555, 0.1249999999999975853 ) ;
#29861=EDGE_LOOP ( 'NONE', ( #15675, #5730, #735, #741 ) ) ;
#29866=ORIENTED_EDGE ( 'NONE', *, *, #13757, .T. ) ;
#29869=DIRECTION ( 'NONE',  ( 1.000000000000000000, 0.000000000000000000, 0.000000000000000000 ) ) ;
#29871=EDGE_CURVE ( 'NONE', #30753, #19067, #31038, .T. ) ;
#29874=CARTESIAN_POINT ( 'NONE',  ( 21.09992658989239089, 25.71664230456640254, 47.04930799450051637 ) ) ;
#29884=CARTESIAN_POINT ( 'NONE',  ( 33.72499318558949710, 31.09184655352422411, 47.04930799450051637 ) ) ;
#29886=DIRECTION ( 'NONE',  ( -1.101824276508909887E-16, 1.000000000000000000, -0.000000000000000000 ) ) ;
#29887=AXIS2_PLACEMENT_3D ( 'NONE', #29824, #7333, #10126 ) ;
#29888=DIRECTION ( 'NONE',  ( -1.000000000000000000, 0.000000000000000000, 0.000000000000000000 ) ) ;
#29889=ORIENTED_EDGE ( 'NONE', *, *, #22787, .T. ) ;
#29893=CARTESIAN_POINT ( 'NONE',  ( 33.50134396954526039, 25.34164230456639899, 47.04930799450051637 ) ) ;
#29894=ADVANCED_FACE ( 'NONE', ( #20589 ), #6135, .F. ) ;
#29896=CIRCLE ( 'NONE', #1570, 12.62506659569710266 ) ;
#29905=DIRECTION ( 'NONE',  ( -1.000000000000000000, 0.000000000000000000, 0.000000000000000000 ) ) ;
#29907=AXIS2_PLACEMENT_3D ( 'NONE', #31880, #9397, #14326 ) ;
#29909=ORIENTED_EDGE ( 'NONE', *, *, #22445, .T. ) ;
#29915=CARTESIAN_POINT ( 'NONE',  ( 33.62634396954518223, 32.59164230456640610, 47.04930799450050927 ) ) ;
#29916=EDGE_CURVE ( 'NONE', #22169, #17679, #7970, .T. ) ;
#29918=DIRECTION ( 'NONE',  ( -1.101824276508909887E-16, 1.000000000000000000, -0.000000000000000000 ) ) ;
#29921=CARTESIAN_POINT ( 'NONE',  ( 8.732853799281738105, 29.96183152705961206, 47.04930799450051637 ) ) ;
#29925=VERTEX_POINT ( 'NONE', #10910 ) ;
#29929=DIRECTION ( 'NONE',  ( -1.000000000000000000, 0.000000000000000000, 0.000000000000000000 ) ) ;
#29931=VERTEX_POINT ( 'NONE', #23217 ) ;
#29934=ORIENTED_EDGE ( 'NONE', *, *, #4217, .T. ) ;
#29935=EDGE_LOOP ( 'NONE', ( #31982, #22581, #4242, #2633 ) ) ;
#29940=DIRECTION ( 'NONE',  ( -1.000000000000000000, 0.000000000000000000, 0.000000000000000000 ) ) ;
#29941=EDGE_LOOP ( 'NONE', ( #30704, #18626, #15803, #21718 ) ) ;
#29947=AXIS2_PLACEMENT_3D ( 'NONE', #18913, #29107, #4148 ) ;
#29949=EDGE_LOOP ( 'NONE', ( #30228, #552, #25702, #14964 ) ) ;
#29952=TOROIDAL_SURFACE ( 'NONE', #5328, 12.61792373059895134, 0.1249999999999985151 ) ;
#29953=ADVANCED_FACE ( 'NONE', ( #27984 ), #20015, .T. ) ;
#29954=ORIENTED_EDGE ( 'NONE', *, *, #23494, .F. ) ;
#29957=CYLINDRICAL_SURFACE ( 'NONE', #5240, 12.62506659569710266 ) ;
#29958=CARTESIAN_POINT ( 'NONE',  ( 21.09992658989239089, 26.84164230456639899, 47.04930799450051637 ) ) ;
#29959=FACE_OUTER_BOUND ( 'NONE', #30650, .T. ) ;
#29960=CARTESIAN_POINT ( 'NONE',  ( 33.37634396954521776, 29.34164230456639899, 47.04930799450051637 ) ) ;
#29966=TOROIDAL_SURFACE ( 'NONE', #17907, 12.40141737965281621, 0.1249999999999985428 ) ;
#29972=ORIENTED_EDGE ( 'NONE', *, *, #26677, .F. ) ;
#29973=CIRCLE ( 'NONE', #9507, 12.27641737965280200 ) ;
#29975=DIRECTION ( 'NONE',  ( 0.000000000000000000, -0.000000000000000000, -1.000000000000000000 ) ) ;
#29976=EDGE_LOOP ( 'NONE', ( #7383, #6895, #6728, #32428 ) ) ;
#29978=ORIENTED_EDGE ( 'NONE', *, *, #10838, .T. ) ;
#29983=ADVANCED_FACE ( 'NONE', ( #20421 ), #4823, .T. ) ;
#29988=EDGE_CURVE ( 'NONE', #6679, #19118, #10598, .T. ) ;
#29990=ADVANCED_FACE ( 'NONE', ( #21218 ), #29437, .T. ) ;
#29991=FACE_OUTER_BOUND ( 'NONE', #20723, .T. ) ;
#30003=DIRECTION ( 'NONE',  ( -1.000000000000000000, 0.000000000000000000, 0.000000000000000000 ) ) ;
#30013=AXIS2_PLACEMENT_3D ( 'NONE', #312, #27406, #25426 ) ;
#30015=ORIENTED_EDGE ( 'NONE', *, *, #20030, .T. ) ;
#30016=CIRCLE ( 'NONE', #10100, 0.1250000000000001110 ) ;
#30024=CIRCLE ( 'NONE', #1183, 12.36707279061065101 ) ;
#30032=AXIS2_PLACEMENT_3D ( 'NONE', #9619, #1739, #29643 ) ;
#30041=CARTESIAN_POINT ( 'NONE',  ( 21.09992658989239089, 26.34184655352419213, 47.04930799450051637 ) ) ;
#30043=CARTESIAN_POINT ( 'NONE',  ( 21.09992658989239089, 27.46664230456639899, 47.04930799450051637 ) ) ;
#30047=EDGE_LOOP ( 'NONE', ( #12256, #5348, #10384, #6101 ) ) ;
#30048=ORIENTED_EDGE ( 'NONE', *, *, #23247, .F. ) ;
#30050=CARTESIAN_POINT ( 'NONE',  ( 21.09992658989239089, 27.09164230456639899, 47.04930799450051637 ) ) ;
#30051=CARTESIAN_POINT ( 'NONE',  ( 8.732853799281732776, 38.56284415653841791, 47.04930799450051637 ) ) ;
#30052=AXIS2_PLACEMENT_3D ( 'NONE', #23764, #21621, #1770 ) ;
#30058=CARTESIAN_POINT ( 'NONE',  ( 21.09992658989239089, 25.46183152705960140, 47.04930799450051637 ) ) ;
#30061=CIRCLE ( 'NONE', #5951, 0.1250000000000001110 ) ;
#30064=ORIENTED_EDGE ( 'NONE', *, *, #1405, .T. ) ;
#30065=VERTEX_POINT ( 'NONE', #26806 ) ;
#30072=CARTESIAN_POINT ( 'NONE',  ( 21.09992658989239089, 29.46664230456640254, 47.04930799450051637 ) ) ;
#30074=DIRECTION ( 'NONE',  ( 0.000000000000000000, -0.000000000000000000, -1.000000000000000000 ) ) ;
#30078=CYLINDRICAL_SURFACE ( 'NONE', #6541, 12.62506659569710266 ) ;
#30081=CYLINDRICAL_SURFACE ( 'NONE', #20498, 12.62506659569710266 ) ;
#30083=AXIS2_PLACEMENT_3D ( 'NONE', #23979, #23816, #29070 ) ;
#30084=CIRCLE ( 'NONE', #8065, 12.62506659569710266 ) ;
#30087=( NAMED_UNIT ( * ) PLANE_ANGLE_UNIT ( ) SI_UNIT ( $, .RADIAN. ) );
#30091=CARTESIAN_POINT ( 'NONE',  ( 21.09992658989239089, 25.59164230456639899, 47.04930799450051637 ) ) ;
#30092=CARTESIAN_POINT ( 'NONE',  ( 21.09992658989238734, 32.46664230456639899, 47.04930799450051637 ) ) ;
#30097=DIRECTION ( 'NONE',  ( -1.101824276508909887E-16, 1.000000000000000000, -0.000000000000000000 ) ) ;
#30099=VERTEX_POINT ( 'NONE', #21373 ) ;
#30109=ORIENTED_EDGE ( 'NONE', *, *, #20665, .F. ) ;
#30111=VERTEX_POINT ( 'NONE', #24998 ) ;
#30115=EDGE_LOOP ( 'NONE', ( #16205, #29456, #22913, #30748 ) ) ;
#30116=FACE_OUTER_BOUND ( 'NONE', #17886, .T. ) ;
#30119=DIRECTION ( 'NONE',  ( -1.000000000000000000, -1.101824276508909764E-16, 0.000000000000000000 ) ) ;
#30127=AXIS2_PLACEMENT_3D ( 'NONE', #22343, #5288, #193 ) ;
#30133=CARTESIAN_POINT ( 'NONE',  ( 8.474859994195286461, 24.59184655352419213, 47.04930799450051637 ) ) ;
#30135=EDGE_CURVE ( 'NONE', #22536, #25197, #14269, .T. ) ;
#30142=ORIENTED_EDGE ( 'NONE', *, *, #30696, .T. ) ;
#30144=ORIENTED_EDGE ( 'NONE', *, *, #1837, .T. ) ;
#30152=ORIENTED_EDGE ( 'NONE', *, *, #29199, .T. ) ;
#30158=DIRECTION ( 'NONE',  ( -1.101824276508909887E-16, 1.000000000000000000, -0.000000000000000000 ) ) ;
#30159=ORIENTED_EDGE ( 'NONE', *, *, #10420, .F. ) ;
#30173=FACE_OUTER_BOUND ( 'NONE', #21285, .T. ) ;
#30176=CIRCLE ( 'NONE', #30683, 12.27641737965279845 ) ;
#30177=ORIENTED_EDGE ( 'NONE', *, *, #24071, .T. ) ;
#30178=AXIS2_PLACEMENT_3D ( 'NONE', #8588, #1035, #8432 ) ;
#30180=VERTEX_POINT ( 'NONE', #4978 ) ;
#30186=EDGE_LOOP ( 'NONE', ( #6542, #3599, #6518, #10740 ) ) ;
#30190=DIRECTION ( 'NONE',  ( -1.101824276508909887E-16, 1.000000000000000000, -0.000000000000000000 ) ) ;
#30196=FACE_OUTER_BOUND ( 'NONE', #20667, .T. ) ;
#30197=VERTEX_POINT ( 'NONE', #10229 ) ;
#30198=CIRCLE ( 'NONE', #19163, 12.62506659569710266 ) ;
#30216=( GEOMETRIC_REPRESENTATION_CONTEXT ( 3 ) GLOBAL_UNCERTAINTY_ASSIGNED_CONTEXT ( ( #16665 ) ) GLOBAL_UNIT_ASSIGNED_CONTEXT ( ( #26106, #6251, #6415 ) ) REPRESENTATION_CONTEXT ( 'NONE', 'WORKASPACE' ) );
#30217=DIRECTION ( 'NONE',  ( -1.101824276508909887E-16, 1.000000000000000000, -0.000000000000000000 ) ) ;
#30223=ORIENTED_EDGE ( 'NONE', *, *, #6664, .T. ) ;
#30224=ORIENTED_EDGE ( 'NONE', *, *, #25435, .F. ) ;
#30228=ORIENTED_EDGE ( 'NONE', *, *, #7464, .F. ) ;
#30230=DIRECTION ( 'NONE',  ( -1.101824276508909887E-16, 1.000000000000000000, -0.000000000000000000 ) ) ;
#30231=DIRECTION ( 'NONE',  ( -1.000000000000000000, 0.000000000000000000, 0.000000000000000000 ) ) ;
#30235=CYLINDRICAL_SURFACE ( 'NONE', #6035, 12.62506659569710443 ) ;
#30250=EDGE_LOOP ( 'NONE', ( #8468, #23982, #17354, #12901 ) ) ;
#30251=DIRECTION ( 'NONE',  ( -1.000000000000000000, 0.000000000000000000, 0.000000000000000000 ) ) ;
#30253=FACE_OUTER_BOUND ( 'NONE', #1463, .T. ) ;
#30258=CARTESIAN_POINT ( 'NONE',  ( 33.72499318558949710, 26.09184655352419213, 47.04930799450051637 ) ) ;
#30259=DIRECTION ( 'NONE',  ( 0.000000000000000000, -0.000000000000000000, -1.000000000000000000 ) ) ;
#30260=DIRECTION ( 'NONE',  ( 0.000000000000000000, -0.000000000000000000, -1.000000000000000000 ) ) ;
#30264=ORIENTED_EDGE ( 'NONE', *, *, #10439, .T. ) ;
#30266=ADVANCED_FACE ( 'NONE', ( #27295 ), #10616, .T. ) ;
#30269=EDGE_CURVE ( 'NONE', #10922, #7990, #1690, .T. ) ;
#30270=ORIENTED_EDGE ( 'NONE', *, *, #744, .F. ) ;
#30273=CIRCLE ( 'NONE', #27641, 12.62506659569710266 ) ;
#30278=ORIENTED_EDGE ( 'NONE', *, *, #22196, .T. ) ;
#30280=VECTOR ( 'NONE', #14992, 1000.000000000000000 ) ;
#30282=ADVANCED_FACE ( 'NONE', ( #1129 ), #21079, .T. ) ;
#30283=AXIS2_PLACEMENT_3D ( 'NONE', #15578, #29886, #12325 ) ;
#30291=DIRECTION ( 'NONE',  ( -1.000000000000000000, 0.000000000000000000, 0.000000000000000000 ) ) ;
#30292=AXIS2_PLACEMENT_3D ( 'NONE', #24693, #32248, #11569 ) ;
#30297=ORIENTED_EDGE ( 'NONE', *, *, #2623, .T. ) ;
#30298=EDGE_CURVE ( 'NONE', #12749, #14790, #2982, .T. ) ;
#30302=CIRCLE ( 'NONE', #20875, 12.36707279061065101 ) ;
#30307=ADVANCED_FACE ( 'NONE', ( #8840 ), #11658, .T. ) ;
#30309=TOROIDAL_SURFACE ( 'NONE', #26645, 12.40141737965282509, 0.1249999999999980849 ) ;
#30310=VERTEX_POINT ( 'NONE', #9007 ) ;
#30311=CARTESIAN_POINT ( 'NONE',  ( 21.09992658989239089, 29.46183152705961206, 47.04930799450051637 ) ) ;
#30321=ORIENTED_EDGE ( 'NONE', *, *, #15892, .T. ) ;
#30334=CIRCLE ( 'NONE', #17727, 0.1250000000000018319 ) ;
#30335=VECTOR ( 'NONE', #174, 1000.000000000000000 ) ;
#30338=CIRCLE ( 'NONE', #13548, 12.62506659569710266 ) ;
#30341=AXIS2_PLACEMENT_3D ( 'NONE', #6739, #6583, #9042 ) ;
#30342=VERTEX_POINT ( 'NONE', #5467 ) ;
#30348=ORIENTED_EDGE ( 'NONE', *, *, #22715, .F. ) ;
#30349=CIRCLE ( 'NONE', #18260, 0.1250000000000001110 ) ;
#30350=CARTESIAN_POINT ( 'NONE',  ( 21.09992658989239089, 25.84184655352419213, 47.04930799450051637 ) ) ;
#30355=ORIENTED_EDGE ( 'NONE', *, *, #3433, .F. ) ;
#30359=TOROIDAL_SURFACE ( 'NONE', #16191, 12.40141737965281976, 0.1249999999999999722 ) ;
#30361=DIRECTION ( 'NONE',  ( -1.000000000000000000, 0.000000000000000000, 0.000000000000000000 ) ) ;
#30362=FACE_OUTER_BOUND ( 'NONE', #29520, .T. ) ;
#30368=LINE ( 'NONE', #22647, #13579 ) ;
#30378=CIRCLE ( 'NONE', #18324, 12.62506659569710266 ) ;
#30385=ORIENTED_EDGE ( 'NONE', *, *, #19468, .F. ) ;
#30391=CIRCLE ( 'NONE', #13623, 0.1250000000000001110 ) ;
#30395=DIRECTION ( 'NONE',  ( -1.000000000000000000, 0.000000000000000000, 0.000000000000000000 ) ) ;
#30399=ADVANCED_FACE ( 'NONE', ( #6703 ), #24755, .F. ) ;
#30401=EDGE_CURVE ( 'NONE', #24621, #11017, #7029, .T. ) ;
#30402=DIRECTION ( 'NONE',  ( -1.101824276508909887E-16, 1.000000000000000000, -0.000000000000000000 ) ) ;
#30408=DIRECTION ( 'NONE',  ( -1.101824276508909887E-16, 1.000000000000000000, -0.000000000000000000 ) ) ;
#30409=AXIS2_PLACEMENT_3D ( 'NONE', #26322, #6464, #24012 ) ;
#30412=ORIENTED_EDGE ( 'NONE', *, *, #15196, .F. ) ;
#30418=ORIENTED_EDGE ( 'NONE', *, *, #18157, .T. ) ;
#30421=CIRCLE ( 'NONE', #12589, 12.62506659569710266 ) ;
#30424=DIRECTION ( 'NONE',  ( -1.000000000000000000, 0.000000000000000000, 0.000000000000000000 ) ) ;
#30426=ORIENTED_EDGE ( 'NONE', *, *, #23480, .F. ) ;
#30435=AXIS2_PLACEMENT_3D ( 'NONE', #14315, #26779, #1343 ) ;
#30437=AXIS2_PLACEMENT_3D ( 'NONE', #29147, #1406, #4197 ) ;
#30438=ORIENTED_EDGE ( 'NONE', *, *, #955, .F. ) ;
#30441=CARTESIAN_POINT ( 'NONE',  ( 21.09992658989239089, 25.34143805560860940, 47.04930799450051637 ) ) ;
#30445=ADVANCED_FACE ( 'NONE', ( #31662 ), #14285, .T. ) ;
#30448=CARTESIAN_POINT ( 'NONE',  ( 21.09992658989238734, 31.22145308207317171, 47.04930799450051637 ) ) ;
#30449=DIRECTION ( 'NONE',  ( 0.000000000000000000, -0.000000000000000000, -1.000000000000000000 ) ) ;
#30454=EDGE_LOOP ( 'NONE', ( #29972, #6834, #13016, #16182 ) ) ;
#30455=CARTESIAN_POINT ( 'NONE',  ( 21.09992658989239089, 29.72145308207318237, 47.04930799450051637 ) ) ;
#30461=DIRECTION ( 'NONE',  ( -1.000000000000000000, 0.000000000000000000, 0.000000000000000000 ) ) ;
#30464=CIRCLE ( 'NONE', #17863, 12.62506659569710443 ) ;
#30479=CIRCLE ( 'NONE', #16312, 12.62506659569710266 ) ;
#30482=CARTESIAN_POINT ( 'NONE',  ( 33.72499318558949710, 29.84184655352422411, 47.04930799450051637 ) ) ;
#30485=EDGE_LOOP ( 'NONE', ( #18943, #12131, #12594, #26509 ) ) ;
#30488=DIRECTION ( 'NONE',  ( 1.000000000000000000, 0.000000000000000000, 0.000000000000000000 ) ) ;
#30493=CARTESIAN_POINT ( 'NONE',  ( 8.482002859293453767, 29.46664230456640254, 47.04930799450051637 ) ) ;
#30494=FACE_OUTER_BOUND ( 'NONE', #29976, .T. ) ;
#30496=AXIS2_PLACEMENT_3D ( 'NONE', #1725, #8783, #14043 ) ;
#30498=DIRECTION ( 'NONE',  ( -1.101824276508909887E-16, 1.000000000000000000, -0.000000000000000000 ) ) ;
#30500=DIRECTION ( 'NONE',  ( -1.000000000000000000, -1.101824276508910010E-16, 0.000000000000000000 ) ) ;
#30503=ORIENTED_EDGE ( 'NONE', *, *, #4009, .F. ) ;
#30506=CARTESIAN_POINT ( 'NONE',  ( 21.09992658989238734, 38.56284415653841791, 47.04930799450051637 ) ) ;
#30509=ORIENTED_EDGE ( 'NONE', *, *, #7951, .T. ) ;
#30511=EDGE_CURVE ( 'NONE', #2007, #4802, #30016, .T. ) ;
#30515=CARTESIAN_POINT ( 'NONE',  ( 21.09992658989239089, 29.84164230456639899, 47.04930799450051637 ) ) ;
#30517=ORIENTED_EDGE ( 'NONE', *, *, #18767, .F. ) ;
#30523=ORIENTED_EDGE ( 'NONE', *, *, #14764, .F. ) ;
#30525=CARTESIAN_POINT ( 'NONE',  ( 8.482002859293473307, 31.96664230456639544, 47.04930799450051637 ) ) ;
#30527=AXIS2_PLACEMENT_3D ( 'NONE', #10501, #2933, #20008 ) ;
#30532=DIRECTION ( 'NONE',  ( -1.101824276508909887E-16, 1.000000000000000000, -0.000000000000000000 ) ) ;
#30541=DIRECTION ( 'NONE',  ( -1.101824276508909887E-16, 1.000000000000000000, -0.000000000000000000 ) ) ;
#30546=AXIS2_PLACEMENT_3D ( 'NONE', #18218, #15928, #28250 ) ;
#30549=ORIENTED_EDGE ( 'NONE', *, *, #14682, .T. ) ;
#30551=AXIS2_PLACEMENT_3D ( 'NONE', #23903, #11755, #4691 ) ;
#30558=CARTESIAN_POINT ( 'NONE',  ( 33.46699938050304013, 38.56284415653841791, 47.04930799450051637 ) ) ;
#30564=DIRECTION ( 'NONE',  ( -1.000000000000000000, 0.000000000000000000, 0.000000000000000000 ) ) ;
#30571=ORIENTED_EDGE ( 'NONE', *, *, #6351, .T. ) ;
#30577=TOROIDAL_SURFACE ( 'NONE', #4867, 12.40141737965281976, 0.1249999999999999722 ) ;
#30578=DIRECTION ( 'NONE',  ( 1.000000000000000000, 0.000000000000000000, 0.000000000000000000 ) ) ;
#30580=DIRECTION ( 'NONE',  ( -1.000000000000000000, -1.101824276508909764E-16, 0.000000000000000000 ) ) ;
#30589=EDGE_LOOP ( 'NONE', ( #13420, #14027, #6860, #2205 ) ) ;
#30592=DIRECTION ( 'NONE',  ( -1.101824276508909887E-16, 1.000000000000000000, -0.000000000000000000 ) ) ;
#30593=CARTESIAN_POINT ( 'NONE',  ( 8.823509210239558698, 29.09164230456639899, 47.04930799450051637 ) ) ;
#30594=ORIENTED_EDGE ( 'NONE', *, *, #31985, .T. ) ;
#30598=DIRECTION ( 'NONE',  ( -1.101824276508909887E-16, 1.000000000000000000, -0.000000000000000000 ) ) ;
#30610=DIRECTION ( 'NONE',  ( -1.101824276508909887E-16, 1.000000000000000000, -0.000000000000000000 ) ) ;
#30612=AXIS2_PLACEMENT_3D ( 'NONE', #18249, #2998, #3155 ) ;
#30623=AXIS2_PLACEMENT_3D ( 'NONE', #16181, #16505, #19609 ) ;
#30630=EDGE_CURVE ( 'NONE', #28214, #10801, #7474, .T. ) ;
#30633=CARTESIAN_POINT ( 'NONE',  ( 33.37634396954519644, 31.09164230456639544, 47.04930799450051637 ) ) ;
#30640=CIRCLE ( 'NONE', #16471, 0.1250000000000001110 ) ;
#30641=DIRECTION ( 'NONE',  ( -1.101824276508909887E-16, 1.000000000000000000, -0.000000000000000000 ) ) ;
#30643=CARTESIAN_POINT ( 'NONE',  ( 33.72499318558949000, 38.56284415653841791, 47.04930799450051637 ) ) ;
#30644=CARTESIAN_POINT ( 'NONE',  ( 33.46699938050303302, 38.56284415653841791, 47.04930799450051637 ) ) ;
#30645=ORIENTED_EDGE ( 'NONE', *, *, #7821, .T. ) ;
#30646=DIRECTION ( 'NONE',  ( -1.000000000000000000, -1.101824276508909887E-16, 0.000000000000000000 ) ) ;
#30647=ORIENTED_EDGE ( 'NONE', *, *, #20665, .T. ) ;
#30650=EDGE_LOOP ( 'NONE', ( #2270, #15736, #17972, #14774 ) ) ;
#30653=CARTESIAN_POINT ( 'NONE',  ( 8.698509210239569356, 30.09164230456639544, 47.04930799450051637 ) ) ;
#30655=CYLINDRICAL_SURFACE ( 'NONE', #21520, 12.62506659569710266 ) ;
#30660=ADVANCED_FACE ( 'NONE', ( #3391 ), #8797, .T. ) ;
#30663=AXIS2_PLACEMENT_3D ( 'NONE', #27270, #14810, #24971 ) ;
#30666=CIRCLE ( 'NONE', #23295, 0.1250000000000001110 ) ;
#30667=AXIS2_PLACEMENT_3D ( 'NONE', #1596, #19477, #32129 ) ;
#30670=ADVANCED_FACE ( 'NONE', ( #11276 ), #30577, .T. ) ;
#30675=CARTESIAN_POINT ( 'NONE',  ( 21.09992658989239089, 26.46183152705960140, 47.04930799450051637 ) ) ;
#30677=DIRECTION ( 'NONE',  ( -1.101824276508909887E-16, 1.000000000000000000, -0.000000000000000000 ) ) ;
#30679=AXIS2_PLACEMENT_3D ( 'NONE', #3294, #20536, #8235 ) ;
#30682=ORIENTED_EDGE ( 'NONE', *, *, #28088, .T. ) ;
#30683=AXIS2_PLACEMENT_3D ( 'NONE', #28975, #4676, #9276 ) ;
#30691=FACE_OUTER_BOUND ( 'NONE', #19633, .T. ) ;
#30696=EDGE_CURVE ( 'NONE', #12851, #4827, #5403, .T. ) ;
#30697=DIRECTION ( 'NONE',  ( -1.224646799147353207E-16, -1.349345573449484691E-32, 1.000000000000000000 ) ) ;
#30702=DIRECTION ( 'NONE',  ( -1.101824276508909887E-16, 1.000000000000000000, -0.000000000000000000 ) ) ;
#30704=ORIENTED_EDGE ( 'NONE', *, *, #28137, .T. ) ;
#30705=TOROIDAL_SURFACE ( 'NONE', #5026, 12.61792373059894246, 0.1249999999999989730 ) ;
#30706=EDGE_CURVE ( 'NONE', #29823, #1311, #12204, .T. ) ;
#30707=TOROIDAL_SURFACE ( 'NONE', #17076, 12.40141737965280200, 0.1249999999999999445 ) ;
#30710=ORIENTED_EDGE ( 'NONE', *, *, #16661, .T. ) ;
#30720=DIRECTION ( 'NONE',  ( -1.000000000000000000, 0.000000000000000000, 0.000000000000000000 ) ) ;
#30722=CARTESIAN_POINT ( 'NONE',  ( 21.09992658989238734, 31.84164230456639544, 47.04930799450051637 ) ) ;
#30723=CARTESIAN_POINT ( 'NONE',  ( 8.732853799281738105, 24.96183152705960140, 47.04930799450051637 ) ) ;
#30725=DIRECTION ( 'NONE',  ( -1.101824276508909887E-16, 1.000000000000000000, -0.000000000000000000 ) ) ;
#30730=ORIENTED_EDGE ( 'NONE', *, *, #8062, .F. ) ;
#30731=ORIENTED_EDGE ( 'NONE', *, *, #30630, .T. ) ;
#30740=DIRECTION ( 'NONE',  ( -1.101824276508909887E-16, 1.000000000000000000, -0.000000000000000000 ) ) ;
#30742=ORIENTED_EDGE ( 'NONE', *, *, #31538, .F. ) ;
#30746=TOROIDAL_SURFACE ( 'NONE', #10314, 12.61792373059898154, 0.1249999999999967248 ) ;
#30748=ORIENTED_EDGE ( 'NONE', *, *, #8974, .F. ) ;
#30752=CARTESIAN_POINT ( 'NONE',  ( 21.09992658989239089, 23.71664230456639899, 47.04930799450051637 ) ) ;
#30753=VERTEX_POINT ( 'NONE', #6180 ) ;
#30756=CYLINDRICAL_SURFACE ( 'NONE', #29887, 12.36707279061065279 ) ;
#30762=DIRECTION ( 'NONE',  ( -1.101824276508909887E-16, 1.000000000000000000, -0.000000000000000000 ) ) ;
#30763=ORIENTED_EDGE ( 'NONE', *, *, #20157, .T. ) ;
#30772=CARTESIAN_POINT ( 'NONE',  ( 33.37634396954527460, 24.09164230456639544, 47.04930799450051637 ) ) ;
#30773=ORIENTED_EDGE ( 'NONE', *, *, #14449, .T. ) ;
#30774=DIRECTION ( 'NONE',  ( -1.000000000000000000, 0.000000000000000000, 0.000000000000000000 ) ) ;
#30776=AXIS2_PLACEMENT_3D ( 'NONE', #32228, #14179, #24496 ) ;
#30778=CARTESIAN_POINT ( 'NONE',  ( 21.09992658989239089, 26.09143805560860940, 47.04930799450051637 ) ) ;
#30782=AXIS2_PLACEMENT_3D ( 'NONE', #4187, #6166, #24369 ) ;
#30784=DIRECTION ( 'NONE',  ( -1.101824276508909887E-16, 1.000000000000000000, -0.000000000000000000 ) ) ;
#30787=CIRCLE ( 'NONE', #392, 0.1250000000000001110 ) ;
#30789=CARTESIAN_POINT ( 'NONE',  ( 8.698509210239523171, 25.84164230456639899, 47.04930799450051637 ) ) ;
#30790=EDGE_LOOP ( 'NONE', ( #16093, #27234, #7706, #27454 ) ) ;
#30796=ORIENTED_EDGE ( 'NONE', *, *, #28710, .F. ) ;
#30800=DIRECTION ( 'NONE',  ( -1.000000000000000000, 0.000000000000000000, 0.000000000000000000 ) ) ;
#30807=EDGE_CURVE ( 'NONE', #2021, #27386, #13789, .T. ) ;
#30809=DIRECTION ( 'NONE',  ( -1.000000000000000000, 0.000000000000000000, 0.000000000000000000 ) ) ;
#30810=EDGE_CURVE ( 'NONE', #9948, #21573, #27400, .T. ) ;
#30815=EDGE_CURVE ( 'NONE', #12709, #25906, #14831, .T. ) ;
#30816=ORIENTED_EDGE ( 'NONE', *, *, #18558, .T. ) ;
#30820=ORIENTED_EDGE ( 'NONE', *, *, #5538, .F. ) ;
#30822=UNCERTAINTY_MEASURE_WITH_UNIT (LENGTH_MEASURE( 1.000000000000000082E-05 ), #10061, 'distance_accuracy_value', 'NONE');
#30824=VERTEX_POINT ( 'NONE', #6831 ) ;
#30830=CARTESIAN_POINT ( 'NONE',  ( 8.823509210239514289, 24.84164230456639544, 47.04930799450051637 ) ) ;
#30831=ADVANCED_FACE ( 'NONE', ( #14383 ), #25323, .T. ) ;
#30835=DIRECTION ( 'NONE',  ( -1.101824276508909887E-16, 1.000000000000000000, -0.000000000000000000 ) ) ;
#30838=TOROIDAL_SURFACE ( 'NONE', #6200, 12.40141737965286062, 0.1249999999999998196 ) ;
#30840=DIRECTION ( 'NONE',  ( -1.000000000000000000, 0.000000000000000000, 0.000000000000000000 ) ) ;
#30849=DIRECTION ( 'NONE',  ( -1.000000000000000000, 0.000000000000000000, 0.000000000000000000 ) ) ;
#30852=DIRECTION ( 'NONE',  ( -1.101824276508909887E-16, 1.000000000000000000, -0.000000000000000000 ) ) ;
#30854=CIRCLE ( 'NONE', #11435, 12.27641737965288904 ) ;
#30857=VERTEX_POINT ( 'NONE', #19612 ) ;
#30860=EDGE_LOOP ( 'NONE', ( #20335, #5428, #6394, #12857 ) ) ;
#30862=ADVANCED_FACE ( 'NONE', ( #1413 ), #21623, .T. ) ;
#30868=EDGE_CURVE ( 'NONE', #30342, #17679, #7497, .T. ) ;
#30870=CARTESIAN_POINT ( 'NONE',  ( 21.09992658989239089, 29.97145308207317527, 47.04930799450051637 ) ) ;
#30871=EDGE_CURVE ( 'NONE', #17692, #5687, #1571, .T. ) ;
#30876=DIRECTION ( 'NONE',  ( -1.000000000000000000, 0.000000000000000000, 0.000000000000000000 ) ) ;
#30886=EDGE_CURVE ( 'NONE', #14337, #29823, #27011, .T. ) ;
#30887=EDGE_LOOP ( 'NONE', ( #22402, #5924, #4313, #18321 ) ) ;
#30890=CIRCLE ( 'NONE', #14109, 12.62506659569710266 ) ;
#30891=DIRECTION ( 'NONE',  ( -1.000000000000000000, 0.000000000000000000, 0.000000000000000000 ) ) ;
#30893=CARTESIAN_POINT ( 'NONE',  ( 21.09992658989239089, 25.96183152705960140, 47.04930799450051637 ) ) ;
#30897=DIRECTION ( 'NONE',  ( -1.101824276508909887E-16, 1.000000000000000000, -0.000000000000000000 ) ) ;
#30899=VECTOR ( 'NONE', #10026, 1000.000000000000000 ) ;
#30901=VECTOR ( 'NONE', #5429, 1000.000000000000000 ) ;
#30903=EDGE_CURVE ( 'NONE', #25423, #20369, #11686, .T. ) ;
#30909=EDGE_CURVE ( 'NONE', #24538, #27344, #2773, .T. ) ;
#30910=AXIS2_PLACEMENT_3D ( 'NONE', #29114, #28628, #21543 ) ;
#30911=ORIENTED_EDGE ( 'NONE', *, *, #18885, .T. ) ;
#30918=CIRCLE ( 'NONE', #31429, 12.27641737965279845 ) ;
#30922=AXIS2_PLACEMENT_3D ( 'NONE', #7035, #26567, #1941 ) ;
#30925=VERTEX_POINT ( 'NONE', #20108 ) ;
#30928=CARTESIAN_POINT ( 'NONE',  ( 8.474859994195282908, 38.56284415653841791, 47.04930799450051637 ) ) ;
#30931=VERTEX_POINT ( 'NONE', #5182 ) ;
#30934=DIRECTION ( 'NONE',  ( -1.101824276508909887E-16, 1.000000000000000000, -0.000000000000000000 ) ) ;
#30935=ORIENTED_EDGE ( 'NONE', *, *, #26572, .T. ) ;
#30939=TOROIDAL_SURFACE ( 'NONE', #4191, 12.40141737965284641, 0.1249999999999995698 ) ;
#30942=EDGE_LOOP ( 'NONE', ( #18509, #12654, #27944, #9523 ) ) ;
#30943=DIRECTION ( 'NONE',  ( -1.101824276508909887E-16, 1.000000000000000000, -0.000000000000000000 ) ) ;
#30945=EDGE_CURVE ( 'NONE', #8602, #28135, #12222, .T. ) ;
#30947=CIRCLE ( 'NONE', #16765, 0.1250000000000001110 ) ;
#30948=EDGE_CURVE ( 'NONE', #7900, #20619, #20066, .T. ) ;
#30949=ORIENTED_EDGE ( 'NONE', *, *, #29258, .F. ) ;
#30956=DIRECTION ( 'NONE',  ( -1.000000000000000000, -1.101824276508909887E-16, 0.000000000000000000 ) ) ;
#30957=AXIS2_PLACEMENT_3D ( 'NONE', #10415, #8272, #20409 ) ;
#30960=ORIENTED_EDGE ( 'NONE', *, *, #29853, .T. ) ;
#30964=DIRECTION ( 'NONE',  ( -1.000000000000000000, 0.000000000000000000, 0.000000000000000000 ) ) ;
#30965=ORIENTED_EDGE ( 'NONE', *, *, #15719, .F. ) ;
#30966=CARTESIAN_POINT ( 'NONE',  ( 21.09992658989239089, 29.84143805560861296, 47.04930799450051637 ) ) ;
#30968=DIRECTION ( 'NONE',  ( -1.224646799147353207E-16, -1.349345573449484691E-32, 1.000000000000000000 ) ) ;
#30971=TOROIDAL_SURFACE ( 'NONE', #16278, 12.40141737965283042, 0.1249999999999995420 ) ;
#30974=DIRECTION ( 'NONE',  ( -1.101824276508909887E-16, 1.000000000000000000, -0.000000000000000000 ) ) ;
#30975=CARTESIAN_POINT ( 'NONE',  ( 21.09992658989238734, 38.56284415653841791, 47.04930799450051637 ) ) ;
#30981=CIRCLE ( 'NONE', #16799, 12.62506659569710443 ) ;
#30986=ORIENTED_EDGE ( 'NONE', *, *, #30991, .F. ) ;
#30988=CIRCLE ( 'NONE', #24676, 12.27641737965288904 ) ;
#30991=EDGE_CURVE ( 'NONE', #17073, #20369, #24252, .T. ) ;
#30994=ORIENTED_EDGE ( 'NONE', *, *, #8618, .T. ) ;
#30995=TOROIDAL_SURFACE ( 'NONE', #2688, 12.40141737965282687, 0.1250000000000004718 ) ;
#31003=DIRECTION ( 'NONE',  ( -1.000000000000000000, -1.101824276508910010E-16, 0.000000000000000000 ) ) ;
#31009=DIRECTION ( 'NONE',  ( -1.000000000000000000, -1.101824276508909887E-16, 0.000000000000000000 ) ) ;
#31010=CARTESIAN_POINT ( 'NONE',  ( 21.09992658989239089, 30.59143805560860585, 47.04930799450051637 ) ) ;
#31012=ORIENTED_EDGE ( 'NONE', *, *, #11440, .T. ) ;
#31016=CIRCLE ( 'NONE', #19992, 0.1250000000000001110 ) ;
#31020=EDGE_LOOP ( 'NONE', ( #32017, #9663, #9589, #13668 ) ) ;
#31022=CYLINDRICAL_SURFACE ( 'NONE', #15146, 12.36707279061065101 ) ;
#31023=EDGE_CURVE ( 'NONE', #5687, #10697, #28457, .T. ) ;
#31024=ORIENTED_EDGE ( 'NONE', *, *, #28841, .F. ) ;
#31030=ADVANCED_FACE ( 'NONE', ( #10435 ), #2397, .F. ) ;
#31038=CIRCLE ( 'NONE', #2728, 12.62506659569710443 ) ;
#31045=DIRECTION ( 'NONE',  ( -1.000000000000000000, -1.101824276508909887E-16, 0.000000000000000000 ) ) ;
#31046=FACE_OUTER_BOUND ( 'NONE', #9836, .T. ) ;
#31047=CARTESIAN_POINT ( 'NONE',  ( 21.09992658989239089, 27.21183152705960495, 47.04930799450051637 ) ) ;
#31049=ORIENTED_EDGE ( 'NONE', *, *, #10278, .T. ) ;
#31054=CIRCLE ( 'NONE', #16413, 12.62506659569710266 ) ;
#31056=DIRECTION ( 'NONE',  ( -1.224646799147353207E-16, -1.349345573449484691E-32, 1.000000000000000000 ) ) ;
#31062=EDGE_CURVE ( 'NONE', #29646, #30180, #29806, .T. ) ;
#31063=AXIS2_PLACEMENT_3D ( 'NONE', #30525, #8041, #2616 ) ;
#31068=ORIENTED_EDGE ( 'NONE', *, *, #10838, .F. ) ;
#31070=CARTESIAN_POINT ( 'NONE',  ( 8.823509210239585343, 32.09164230456639899, 47.04930799450051637 ) ) ;
#31071=CARTESIAN_POINT ( 'NONE',  ( 21.09992658989239089, 23.84184655352419213, 47.04930799450051637 ) ) ;
#31083=EDGE_CURVE ( 'NONE', #18497, #321, #12253, .T. ) ;
#31084=DIRECTION ( 'NONE',  ( -1.000000000000000000, -1.101824276508909887E-16, 0.000000000000000000 ) ) ;
#31087=CARTESIAN_POINT ( 'NONE',  ( 33.46699938050303302, 38.56284415653841791, 47.04930799450051637 ) ) ;
#31088=DIRECTION ( 'NONE',  ( -1.000000000000000000, 0.000000000000000000, 0.000000000000000000 ) ) ;
#31090=EDGE_CURVE ( 'NONE', #231, #11810, #5948, .T. ) ;
#31091=CARTESIAN_POINT ( 'NONE',  ( 21.09992658989239089, 23.59164230456639544, 47.04930799450051637 ) ) ;
#31097=ORIENTED_EDGE ( 'NONE', *, *, #27936, .F. ) ;
#31103=DIRECTION ( 'NONE',  ( -1.000000000000000000, 0.000000000000000000, 0.000000000000000000 ) ) ;
#31106=ORIENTED_EDGE ( 'NONE', *, *, #6994, .F. ) ;
#31109=AXIS2_PLACEMENT_3D ( 'NONE', #10666, #30677, #18180 ) ;
#31110=ORIENTED_EDGE ( 'NONE', *, *, #10814, .T. ) ;
#31111=TOROIDAL_SURFACE ( 'NONE', #13815, 12.40141737965287128, 0.1249999999999993477 ) ;
#31116=DIRECTION ( 'NONE',  ( -1.101824276508909887E-16, 1.000000000000000000, -0.000000000000000000 ) ) ;
#31121=CARTESIAN_POINT ( 'NONE',  ( 21.09992658989239089, 28.71183152705961206, 47.04930799450051637 ) ) ;
#31123=EDGE_CURVE ( 'NONE', #31925, #5749, #1741, .T. ) ;
#31126=CARTESIAN_POINT ( 'NONE',  ( 21.09992658989239089, 27.59184655352419568, 47.04930799450051637 ) ) ;
#31130=ORIENTED_EDGE ( 'NONE', *, *, #28504, .T. ) ;
#31132=ADVANCED_FACE ( 'NONE', ( #25998 ), #11703, .T. ) ;
#31137=CIRCLE ( 'NONE', #22739, 12.36707279061065101 ) ;
#31138=ORIENTED_EDGE ( 'NONE', *, *, #19402, .T. ) ;
#31139=DIRECTION ( 'NONE',  ( -1.000000000000000000, 0.000000000000000000, 0.000000000000000000 ) ) ;
#31147=TOROIDAL_SURFACE ( 'NONE', #4395, 12.40141737965287660, 0.1250000000000007772 ) ;
#31149=PRODUCT_DEFINITION_CONTEXT ( 'detailed design', #6357, 'design' ) ;
#31150=ORIENTED_EDGE ( 'NONE', *, *, #1766, .T. ) ;
#31151=CIRCLE ( 'NONE', #8671, 12.36707279061065101 ) ;
#31152=ORIENTED_EDGE ( 'NONE', *, *, #31090, .F. ) ;
#31159=VERTEX_POINT ( 'NONE', #13232 ) ;
#31161=ORIENTED_EDGE ( 'NONE', *, *, #26671, .F. ) ;
#31162=DIRECTION ( 'NONE',  ( -1.000000000000000000, 0.000000000000000000, 0.000000000000000000 ) ) ;
#31165=CIRCLE ( 'NONE', #29572, 12.62506659569710266 ) ;
#31166=CIRCLE ( 'NONE', #7047, 12.36707279061065101 ) ;
#31167=CARTESIAN_POINT ( 'NONE',  ( 21.09992658989238734, 32.09164230456639899, 47.04930799450051637 ) ) ;
#31171=ORIENTED_EDGE ( 'NONE', *, *, #23494, .T. ) ;
#31173=DIRECTION ( 'NONE',  ( 1.000000000000000000, 0.000000000000000000, 0.000000000000000000 ) ) ;
#31174=TOROIDAL_SURFACE ( 'NONE', #21187, 12.61792373059894068, 0.1249999999999991118 ) ;
#31177=EDGE_CURVE ( 'NONE', #16985, #17658, #13288, .T. ) ;
#31179=DIRECTION ( 'NONE',  ( -1.101824276508909887E-16, 1.000000000000000000, -0.000000000000000000 ) ) ;
#31180=CARTESIAN_POINT ( 'NONE',  ( 8.823509210239564027, 29.59164230456639899, 47.04930799450051637 ) ) ;
#31181=EDGE_CURVE ( 'NONE', #2384, #7990, #12779, .T. ) ;
#31183=DIRECTION ( 'NONE',  ( -1.101824276508909887E-16, 1.000000000000000000, -0.000000000000000000 ) ) ;
#31189=ORIENTED_EDGE ( 'NONE', *, *, #11566, .T. ) ;
#31190=AXIS2_PLACEMENT_3D ( 'NONE', #24818, #12519, #29745 ) ;
#31191=DIRECTION ( 'NONE',  ( 1.000000000000000000, 0.000000000000000000, 0.000000000000000000 ) ) ;
#31194=CARTESIAN_POINT ( 'NONE',  ( 21.09992658989239089, 24.34164230456639544, 47.04930799450051637 ) ) ;
#31195=AXIS2_PLACEMENT_3D ( 'NONE', #17629, #25023, #27646 ) ;
#31200=DIRECTION ( 'NONE',  ( -1.101824276508909887E-16, 1.000000000000000000, -0.000000000000000000 ) ) ;
#31201=EDGE_LOOP ( 'NONE', ( #6194, #7726, #6845, #27631 ) ) ;
#31202=CYLINDRICAL_SURFACE ( 'NONE', #1272, 12.62506659569710443 ) ;
#31208=ORIENTED_EDGE ( 'NONE', *, *, #17114, .T. ) ;
#31212=EDGE_CURVE ( 'NONE', #10074, #21925, #22185, .T. ) ;
#31213=CARTESIAN_POINT ( 'NONE',  ( 21.09992658989239089, 24.46664230456639899, 47.04930799450051637 ) ) ;
#31214=ADVANCED_FACE ( 'NONE', ( #14346 ), #31111, .T. ) ;
#31215=AXIS2_PLACEMENT_3D ( 'NONE', #1112, #3734, #8669 ) ;
#31218=FACE_OUTER_BOUND ( 'NONE', #9510, .T. ) ;
#31227=CARTESIAN_POINT ( 'NONE',  ( 21.09992658989239089, 27.47145308207318593, 47.04930799450051637 ) ) ;
#31228=CIRCLE ( 'NONE', #2913, 12.36707279061065279 ) ;
#31229=CIRCLE ( 'NONE', #9750, 0.1249999999999983763 ) ;
#31233=DIRECTION ( 'NONE',  ( -1.101824276508909887E-16, 1.000000000000000000, -0.000000000000000000 ) ) ;
#31235=DIRECTION ( 'NONE',  ( -1.101824276508909887E-16, 1.000000000000000000, -0.000000000000000000 ) ) ;
#31240=ORIENTED_EDGE ( 'NONE', *, *, #23309, .F. ) ;
#31241=CARTESIAN_POINT ( 'NONE',  ( 33.50134396954525329, 26.09164230456639899, 47.04930799450051637 ) ) ;
#31247=DIRECTION ( 'NONE',  ( -1.000000000000000000, 0.000000000000000000, 0.000000000000000000 ) ) ;
#31251=AXIS2_PLACEMENT_3D ( 'NONE', #11096, #21080, #24515 ) ;
#31259=DIRECTION ( 'NONE',  ( -1.101824276508909887E-16, 1.000000000000000000, -0.000000000000000000 ) ) ;
#31266=ORIENTED_EDGE ( 'NONE', *, *, #21426, .F. ) ;
#31268=ADVANCED_FACE ( 'NONE', ( #4160 ), #3849, .T. ) ;
#31269=AXIS2_PLACEMENT_3D ( 'NONE', #25168, #2838, #27793 ) ;
#31278=DIRECTION ( 'NONE',  ( -1.000000000000000000, -1.101824276508909887E-16, 0.000000000000000000 ) ) ;
#31279=CARTESIAN_POINT ( 'NONE',  ( 33.46699938050304013, 30.22145308207317527, 47.04930799450050927 ) ) ;
#31281=DIRECTION ( 'NONE',  ( -1.101824276508909887E-16, 1.000000000000000000, -0.000000000000000000 ) ) ;
#31282=FACE_OUTER_BOUND ( 'NONE', #19004, .T. ) ;
#31284=VECTOR ( 'NONE', #481, 1000.000000000000000 ) ;
#31288=DIRECTION ( 'NONE',  ( -1.224646799147353207E-16, -1.349345573449484691E-32, 1.000000000000000000 ) ) ;
#31289=CARTESIAN_POINT ( 'NONE',  ( 8.474859994195282908, 38.56284415653841791, 47.04930799450051637 ) ) ;
#31292=ORIENTED_EDGE ( 'NONE', *, *, #1108, .T. ) ;
#31293=CARTESIAN_POINT ( 'NONE',  ( 21.09992658989239089, 24.22145308207319303, 47.04930799450051637 ) ) ;
#31302=ORIENTED_EDGE ( 'NONE', *, *, #7680, .F. ) ;
#31309=ADVANCED_FACE ( 'NONE', ( #9751 ), #19560, .T. ) ;
#31330=DIRECTION ( 'NONE',  ( -1.101824276508909887E-16, 1.000000000000000000, -0.000000000000000000 ) ) ;
#31331=CIRCLE ( 'NONE', #12990, 12.27641737965280200 ) ;
#31332=CYLINDRICAL_SURFACE ( 'NONE', #31400, 12.36707279061065101 ) ;
#31333=TOROIDAL_SURFACE ( 'NONE', #14631, 12.40141737965285174, 0.1249999999999993200 ) ;
#31334=DIRECTION ( 'NONE',  ( -1.000000000000000000, -1.101824276508909887E-16, 0.000000000000000000 ) ) ;
#31336=ORIENTED_EDGE ( 'NONE', *, *, #21401, .F. ) ;
#31337=CARTESIAN_POINT ( 'NONE',  ( 21.09992658989238734, 38.56284415653841791, 47.04930799450051637 ) ) ;
#31338=VECTOR ( 'NONE', #18117, 1000.000000000000000 ) ;
#31339=EDGE_LOOP ( 'NONE', ( #2919, #28015, #905, #8628 ) ) ;
#31340=DIRECTION ( 'NONE',  ( -1.101824276508909887E-16, 1.000000000000000000, -0.000000000000000000 ) ) ;
#31343=VERTEX_POINT ( 'NONE', #29769 ) ;
#31346=ORIENTED_EDGE ( 'NONE', *, *, #23203, .T. ) ;
#31351=CIRCLE ( 'NONE', #17187, 12.52641737965279489 ) ;
#31352=EDGE_CURVE ( 'NONE', #10115, #24757, #4891, .T. ) ;
#31355=CARTESIAN_POINT ( 'NONE',  ( 21.09992658989238734, 32.22145308207317527, 47.04930799450051637 ) ) ;
#31356=AXIS2_PLACEMENT_3D ( 'NONE', #28550, #25152, #50 ) ;
#31368=CARTESIAN_POINT ( 'NONE',  ( 21.09992658989239089, 29.59184655352418858, 47.04930799450051637 ) ) ;
#31370=DIRECTION ( 'NONE',  ( -1.101824276508909887E-16, 1.000000000000000000, -0.000000000000000000 ) ) ;
#31373=CARTESIAN_POINT ( 'NONE',  ( 21.09992658989238734, 31.34164230456639544, 47.04930799450051637 ) ) ;
#31377=AXIS2_PLACEMENT_3D ( 'NONE', #28281, #20724, #18721 ) ;
#31379=CIRCLE ( 'NONE', #16154, 0.1250000000000001110 ) ;
#31381=VECTOR ( 'NONE', #13493, 1000.000000000000000 ) ;
#31384=DIRECTION ( 'NONE',  ( -1.101824276508909887E-16, 1.000000000000000000, -0.000000000000000000 ) ) ;
#31386=CARTESIAN_POINT ( 'NONE',  ( 33.46699938050304013, 30.71183152705961916, 47.04930799450051637 ) ) ;
#31388=ADVANCED_FACE ( 'NONE', ( #22860 ), #22367, .T. ) ;
#31389=ORIENTED_EDGE ( 'NONE', *, *, #6346, .F. ) ;
#31391=EDGE_CURVE ( 'NONE', #12749, #1400, #10160, .T. ) ;
#31394=FACE_OUTER_BOUND ( 'NONE', #24955, .T. ) ;
#31400=AXIS2_PLACEMENT_3D ( 'NONE', #10837, #13614, #18677 ) ;
#31408=DIRECTION ( 'NONE',  ( -1.000000000000000000, -1.101824276508909887E-16, 0.000000000000000000 ) ) ;
#31415=LINE ( 'NONE', #16785, #27778 ) ;
#31416=EDGE_LOOP ( 'NONE', ( #5177, #4839, #3653, #22283 ) ) ;
#31418=DIRECTION ( 'NONE',  ( -1.000000000000000000, -1.101824276508909764E-16, 0.000000000000000000 ) ) ;
#31420=CARTESIAN_POINT ( 'NONE',  ( 21.09992658989238734, 31.59164230456639544, 47.04930799450051637 ) ) ;
#31425=AXIS2_PLACEMENT_3D ( 'NONE', #6810, #8945, #16969 ) ;
#31427=VERTEX_POINT ( 'NONE', #4654 ) ;
#31428=AXIS2_PLACEMENT_3D ( 'NONE', #31373, #29398, #24303 ) ;
#31429=AXIS2_PLACEMENT_3D ( 'NONE', #17610, #5314, #217 ) ;
#31430=EDGE_CURVE ( 'NONE', #16793, #9226, #23258, .T. ) ;
#31431=EDGE_CURVE ( 'NONE', #13965, #14963, #31137, .T. ) ;
#31432=EDGE_CURVE ( 'NONE', #3559, #11753, #5964, .T. ) ;
#31433=AXIS2_PLACEMENT_3D ( 'NONE', #140, #10482, #8020 ) ;
#31435=FACE_OUTER_BOUND ( 'NONE', #7530, .T. ) ;
#31437=ADVANCED_FACE ( 'NONE', ( #27628 ), #22702, .F. ) ;
#31438=AXIS2_PLACEMENT_3D ( 'NONE', #27828, #404, #30291 ) ;
#31439=ORIENTED_EDGE ( 'NONE', *, *, #22901, .F. ) ;
#31441=ORIENTED_EDGE ( 'NONE', *, *, #1580, .T. ) ;
#31444=ORIENTED_EDGE ( 'NONE', *, *, #27757, .F. ) ;
#31445=CARTESIAN_POINT ( 'NONE',  ( 33.72499318558949000, 38.56284415653841791, 47.04930799450051637 ) ) ;
#31446=CARTESIAN_POINT ( 'NONE',  ( 21.09992658989239089, 30.59143805560860585, 47.04930799450051637 ) ) ;
#31453=CARTESIAN_POINT ( 'NONE',  ( 8.474859994195281132, 38.56284415653841791, 47.04930799450051637 ) ) ;
#31455=EDGE_LOOP ( 'NONE', ( #15265, #21303, #25879, #22698 ) ) ;
#31457=DIRECTION ( 'NONE',  ( -1.000000000000000000, 0.000000000000000000, 0.000000000000000000 ) ) ;
#31459=CARTESIAN_POINT ( 'NONE',  ( 21.09992658989238734, 38.56284415653841791, 47.04930799450051637 ) ) ;
#31460=AXIS2_PLACEMENT_3D ( 'NONE', #1795, #1304, #6564 ) ;
#31464=AXIS2_PLACEMENT_3D ( 'NONE', #23812, #30897, #18713 ) ;
#31468=AXIS2_PLACEMENT_3D ( 'NONE', #15608, #28256, #351 ) ;
#31474=CARTESIAN_POINT ( 'NONE',  ( 21.09992658989238734, 38.56284415653841791, 47.04930799450051637 ) ) ;
#31477=CIRCLE ( 'NONE', #10524, 0.1250000000000001110 ) ;
#31482=AXIS2_PLACEMENT_3D ( 'NONE', #6174, #18635, #25722 ) ;
#31485=DIRECTION ( 'NONE',  ( -1.101824276508909887E-16, 1.000000000000000000, -0.000000000000000000 ) ) ;
#31487=CYLINDRICAL_SURFACE ( 'NONE', #12137, 12.36707279061065101 ) ;
#31500=CARTESIAN_POINT ( 'NONE',  ( 21.09992658989238734, 38.56284415653841791, 47.04930799450051637 ) ) ;
#31503=VERTEX_POINT ( 'NONE', #18410 ) ;
#31508=AXIS2_PLACEMENT_3D ( 'NONE', #4357, #21902, #4517 ) ;
#31512=VECTOR ( 'NONE', #599, 1000.000000000000000 ) ;
#31513=CIRCLE ( 'NONE', #29947, 12.62506659569710266 ) ;
#31515=ORIENTED_EDGE ( 'NONE', *, *, #23439, .F. ) ;
#31520=ORIENTED_EDGE ( 'NONE', *, *, #16257, .T. ) ;
#31524=EDGE_LOOP ( 'NONE', ( #24300, #10679, #7130, #25258 ) ) ;
#31525=ORIENTED_EDGE ( 'NONE', *, *, #18767, .T. ) ;
#31528=CARTESIAN_POINT ( 'NONE',  ( 33.50134396954523908, 27.59164230456639544, 47.04930799450051637 ) ) ;
#31536=DIRECTION ( 'NONE',  ( -1.000000000000000000, 0.000000000000000000, 0.000000000000000000 ) ) ;
#31538=EDGE_CURVE ( 'NONE', #21064, #21045, #24301, .T. ) ;
#31547=DIRECTION ( 'NONE',  ( -1.000000000000000000, 0.000000000000000000, 0.000000000000000000 ) ) ;
#31548=ADVANCED_FACE ( 'NONE', ( #1334 ), #6914, .F. ) ;
#31550=AXIS2_PLACEMENT_3D ( 'NONE', #29299, #26349, #28818 ) ;
#31551=AXIS2_PLACEMENT_3D ( 'NONE', #5502, #25517, #25835 ) ;
#31552=CARTESIAN_POINT ( 'NONE',  ( 8.823509210239581790, 31.59164230456639544, 47.04930799450051637 ) ) ;
#31558=CARTESIAN_POINT ( 'NONE',  ( 8.732853799281738105, 29.71183152705961561, 47.04930799450051637 ) ) ;
#31560=DIRECTION ( 'NONE',  ( -1.101824276508909887E-16, 1.000000000000000000, -0.000000000000000000 ) ) ;
#31561=DIRECTION ( 'NONE',  ( -1.000000000000000000, 0.000000000000000000, 0.000000000000000000 ) ) ;
#31565=AXIS2_PLACEMENT_3D ( 'NONE', #15688, #25707, #910 ) ;
#31572=AXIS2_PLACEMENT_3D ( 'NONE', #19842, #1266, #10825 ) ;
#31586=ADVANCED_FACE ( 'NONE', ( #21339 ), #16915, .T. ) ;
#31587=ORIENTED_EDGE ( 'NONE', *, *, #16516, .F. ) ;
#31599=CARTESIAN_POINT ( 'NONE',  ( 33.72499318558949710, 31.34143805560860585, 47.04930799450051637 ) ) ;
#31600=ORIENTED_EDGE ( 'NONE', *, *, #30945, .F. ) ;
#31615=CARTESIAN_POINT ( 'NONE',  ( 8.732853799281734553, 38.56284415653841791, 47.04930799450051637 ) ) ;
#31616=CIRCLE ( 'NONE', #26372, 0.1249999999999983763 ) ;
#31618=DIRECTION ( 'NONE',  ( -1.101824276508909887E-16, 1.000000000000000000, -0.000000000000000000 ) ) ;
#31620=EDGE_CURVE ( 'NONE', #104, #29220, #13313, .T. ) ;
#31622=ORIENTED_EDGE ( 'NONE', *, *, #24805, .F. ) ;
#31624=VECTOR ( 'NONE', #5024, 1000.000000000000000 ) ;
#31628=EDGE_CURVE ( 'NONE', #16708, #9505, #29564, .T. ) ;
#31630=TOROIDAL_SURFACE ( 'NONE', #29531, 12.40141737965281088, 0.1249999999999987788 ) ;
#31631=CIRCLE ( 'NONE', #15913, 12.27641737965284108 ) ;
#31637=AXIS2_PLACEMENT_3D ( 'NONE', #800, #15902, #31003 ) ;
#31639=AXIS2_PLACEMENT_3D ( 'NONE', #2836, #373, #29940 ) ;
#31640=AXIS2_PLACEMENT_3D ( 'NONE', #3231, #23577, #26033 ) ;
#31644=VERTEX_POINT ( 'NONE', #1492 ) ;
#31649=VERTEX_POINT ( 'NONE', #8887 ) ;
#31651=DIRECTION ( 'NONE',  ( 1.000000000000000000, 0.000000000000000000, 0.000000000000000000 ) ) ;
#31660=CARTESIAN_POINT ( 'NONE',  ( 21.09992658989239089, 25.21664230456640254, 47.04930799450051637 ) ) ;
#31662=FACE_OUTER_BOUND ( 'NONE', #4291, .T. ) ;
#31663=DIRECTION ( 'NONE',  ( -1.000000000000000000, 0.000000000000000000, 0.000000000000000000 ) ) ;
#31667=CARTESIAN_POINT ( 'NONE',  ( 21.09992658989239089, 27.84164230456639544, 47.04930799450051637 ) ) ;
#31671=ADVANCED_FACE ( 'NONE', ( #28923 ), #26446, .T. ) ;
#31684=AXIS2_PLACEMENT_3D ( 'NONE', #6282, #4137, #31561 ) ;
#31685=EDGE_CURVE ( 'NONE', #1229, #12851, #10238, .T. ) ;
#31688=FACE_OUTER_BOUND ( 'NONE', #18290, .T. ) ;
#31692=ORIENTED_EDGE ( 'NONE', *, *, #13470, .T. ) ;
#31693=DIRECTION ( 'NONE',  ( -1.000000000000000000, 0.000000000000000000, 0.000000000000000000 ) ) ;
#31699=EDGE_LOOP ( 'NONE', ( #1307, #7226, #3546, #27292 ) ) ;
#31705=AXIS2_PLACEMENT_3D ( 'NONE', #24242, #6686, #7013 ) ;
#31706=TOROIDAL_SURFACE ( 'NONE', #11250, 12.40141737965279667, 0.1249999999999991951 ) ;
#31707=CIRCLE ( 'NONE', #21733, 12.27641737965280200 ) ;
#31715=CARTESIAN_POINT ( 'NONE',  ( 8.732853799281731000, 28.72145308207318237, 47.04930799450051637 ) ) ;
#31720=EDGE_CURVE ( 'NONE', #19781, #28214, #23319, .T. ) ;
#31721=DIRECTION ( 'NONE',  ( -1.101824276508909887E-16, 1.000000000000000000, -0.000000000000000000 ) ) ;
#31728=DIRECTION ( 'NONE',  ( -1.101824276508909887E-16, 1.000000000000000000, -0.000000000000000000 ) ) ;
#31730=CIRCLE ( 'NONE', #17575, 12.36707279061065279 ) ;
#31733=TOROIDAL_SURFACE ( 'NONE', #19671, 12.61792373059861028, 0.1250000000000006106 ) ;
#31735=ORIENTED_EDGE ( 'NONE', *, *, #16585, .F. ) ;
#31736=DIRECTION ( 'NONE',  ( -1.000000000000000000, 0.000000000000000000, 0.000000000000000000 ) ) ;
#31741=DIRECTION ( 'NONE',  ( -1.000000000000000000, -1.101824276508909887E-16, 0.000000000000000000 ) ) ;
#31743=DIRECTION ( 'NONE',  ( -1.224646799147353207E-16, -1.349345573449484691E-32, 1.000000000000000000 ) ) ;
#31747=ORIENTED_EDGE ( 'NONE', *, *, #7127, .T. ) ;
#31749=ADVANCED_FACE ( 'NONE', ( #27427 ), #31706, .T. ) ;
#31751=AXIS2_PLACEMENT_3D ( 'NONE', #6455, #26628, #16454 ) ;
#31753=DIRECTION ( 'NONE',  ( -1.101824276508909887E-16, 1.000000000000000000, -0.000000000000000000 ) ) ;
#31755=FACE_OUTER_BOUND ( 'NONE', #29949, .T. ) ;
#31761=DIRECTION ( 'NONE',  ( -1.000000000000000000, 0.000000000000000000, 0.000000000000000000 ) ) ;
#31763=DIRECTION ( 'NONE',  ( -1.000000000000000000, 0.000000000000000000, 0.000000000000000000 ) ) ;
#31765=DIRECTION ( 'NONE',  ( -1.000000000000000000, -1.101824276508909887E-16, 0.000000000000000000 ) ) ;
#31766=CARTESIAN_POINT ( 'NONE',  ( 8.732853799281734553, 29.22145308207318237, 47.04930799450051637 ) ) ;
#31771=CARTESIAN_POINT ( 'NONE',  ( 21.09992658989239089, 28.47145308207318237, 47.04930799450051637 ) ) ;
#31784=AXIS2_PLACEMENT_3D ( 'NONE', #23134, #2943, #650 ) ;
#31794=CARTESIAN_POINT ( 'NONE',  ( 33.46699938050302592, 31.47145308207317882, 47.04930799450050927 ) ) ;
#31797=ORIENTED_EDGE ( 'NONE', *, *, #21858, .T. ) ;
#31798=DIRECTION ( 'NONE',  ( 1.000000000000000000, 0.000000000000000000, 0.000000000000000000 ) ) ;
#31801=ORIENTED_EDGE ( 'NONE', *, *, #7161, .F. ) ;
#31803=DIRECTION ( 'NONE',  ( -1.000000000000000000, -1.101824276508909887E-16, 0.000000000000000000 ) ) ;
#31804=CIRCLE ( 'NONE', #3487, 12.62506659569710266 ) ;
#31805=DIRECTION ( 'NONE',  ( -1.101824276508909887E-16, 1.000000000000000000, -0.000000000000000000 ) ) ;
#31811=ORIENTED_EDGE ( 'NONE', *, *, #23159, .F. ) ;
#31820=EDGE_CURVE ( 'NONE', #13562, #14664, #19703, .T. ) ;
#31821=CARTESIAN_POINT ( 'NONE',  ( 21.09992658989239089, 27.34184655352419568, 47.04930799450051637 ) ) ;
#31822=EDGE_LOOP ( 'NONE', ( #9114, #30152, #16453, #12642 ) ) ;
#31824=ORIENTED_EDGE ( 'NONE', *, *, #15474, .F. ) ;
#31827=CARTESIAN_POINT ( 'NONE',  ( 8.474859994195286461, 24.59143805560860940, 47.04930799450051637 ) ) ;
#31828=ORIENTED_EDGE ( 'NONE', *, *, #15635, .F. ) ;
#31829=TOROIDAL_SURFACE ( 'NONE', #16106, 12.40141737965283397, 0.1249999999999992922 ) ;
#31832=EDGE_CURVE ( 'NONE', #5841, #31904, #5587, .T. ) ;
#31833=AXIS2_PLACEMENT_3D ( 'NONE', #9381, #16436, #4294 ) ;
#31837=ORIENTED_EDGE ( 'NONE', *, *, #256, .T. ) ;
#31839=ORIENTED_EDGE ( 'NONE', *, *, #22990, .F. ) ;
#31841=VERTEX_POINT ( 'NONE', #10350 ) ;
#31843=DIRECTION ( 'NONE',  ( -1.000000000000000000, 0.000000000000000000, 0.000000000000000000 ) ) ;
#31845=AXIS2_PLACEMENT_3D ( 'NONE', #4639, #11867, #12028 ) ;
#31852=AXIS2_PLACEMENT_3D ( 'NONE', #22378, #17294, #15011 ) ;
#31856=CARTESIAN_POINT ( 'NONE',  ( 33.71785032049135111, 26.96664230456639899, 47.04930799450051637 ) ) ;
#31859=EDGE_CURVE ( 'NONE', #28129, #26531, #4985, .T. ) ;
#31862=AXIS2_PLACEMENT_3D ( 'NONE', #26406, #8843, #1287 ) ;
#31866=AXIS2_PLACEMENT_3D ( 'NONE', #31977, #17525, #22281 ) ;
#31873=DIRECTION ( 'NONE',  ( -1.101824276508909887E-16, 1.000000000000000000, -0.000000000000000000 ) ) ;
#31880=CARTESIAN_POINT ( 'NONE',  ( 33.50134396954525329, 26.34164230456639899, 47.04930799450051637 ) ) ;
#31892=CARTESIAN_POINT ( 'NONE',  ( 33.72499318558949710, 30.84143805560860585, 47.04930799450051637 ) ) ;
#31894=CIRCLE ( 'NONE', #963, 12.27641737965288371 ) ;
#31904=VERTEX_POINT ( 'NONE', #113 ) ;
#31905=DIRECTION ( 'NONE',  ( -1.101824276508909887E-16, 1.000000000000000000, -0.000000000000000000 ) ) ;
#31907=EDGE_CURVE ( 'NONE', #30099, #1027, #14394, .T. ) ;
#31912=AXIS2_PLACEMENT_3D ( 'NONE', #4049, #12102, #2078 ) ;
#31913=TOROIDAL_SURFACE ( 'NONE', #13071, 12.61792373059895667, 0.1249999999999982098 ) ;
#31915=TOROIDAL_SURFACE ( 'NONE', #25097, 12.40141737965288371, 0.1249999999999996253 ) ;
#31918=EDGE_LOOP ( 'NONE', ( #2303, #3088, #7338, #8225 ) ) ;
#31919=CIRCLE ( 'NONE', #2592, 12.36707279061065101 ) ;
#31922=DIRECTION ( 'NONE',  ( -1.000000000000000000, 0.000000000000000000, 0.000000000000000000 ) ) ;
#31925=VERTEX_POINT ( 'NONE', #12111 ) ;
#31932=VERTEX_POINT ( 'NONE', #17172 ) ;
#31936=ORIENTED_EDGE ( 'NONE', *, *, #12421, .F. ) ;
#31937=DIRECTION ( 'NONE',  ( -1.000000000000000000, 0.000000000000000000, 0.000000000000000000 ) ) ;
#31938=AXIS2_PLACEMENT_3D ( 'NONE', #21927, #6522, #28849 ) ;
#31939=AXIS2_PLACEMENT_3D ( 'NONE', #7975, #10277, #25521 ) ;
#31942=EDGE_LOOP ( 'NONE', ( #20648, #19359, #13598, #914 ) ) ;
#31943=ORIENTED_EDGE ( 'NONE', *, *, #11481, .T. ) ;
#31944=EDGE_CURVE ( 'NONE', #5329, #3369, #4432, .T. ) ;
#31959=ORIENTED_EDGE ( 'NONE', *, *, #5362, .T. ) ;
#31960=EDGE_LOOP ( 'NONE', ( #24858, #24719, #5830, #12434 ) ) ;
#31962=VERTEX_POINT ( 'NONE', #10941 ) ;
#31964=CARTESIAN_POINT ( 'NONE',  ( 21.09992658989238734, 30.84164230456639544, 47.04930799450051637 ) ) ;
#31969=DIRECTION ( 'NONE',  ( -1.101824276508909887E-16, 1.000000000000000000, -0.000000000000000000 ) ) ;
#31971=TOROIDAL_SURFACE ( 'NONE', #17815, 12.40141737965282154, 0.1250000000000006939 ) ;
#31973=DIRECTION ( 'NONE',  ( -1.101824276508909887E-16, 1.000000000000000000, -0.000000000000000000 ) ) ;
#31974=ORIENTED_EDGE ( 'NONE', *, *, #11719, .T. ) ;
#31977=CARTESIAN_POINT ( 'NONE',  ( 21.09992658989239089, 23.59164230456639544, 47.04930799450051637 ) ) ;
#31978=DIRECTION ( 'NONE',  ( -1.101824276508909887E-16, 1.000000000000000000, -0.000000000000000000 ) ) ;
#31982=ORIENTED_EDGE ( 'NONE', *, *, #19658, .T. ) ;
#31985=EDGE_CURVE ( 'NONE', #21006, #25197, #26971, .T. ) ;
#31989=AXIS2_PLACEMENT_3D ( 'NONE', #26909, #6238, #14113 ) ;
#31990=AXIS2_PLACEMENT_3D ( 'NONE', #18867, #13805, #28905 ) ;
#31991=EDGE_LOOP ( 'NONE', ( #21445, #11802, #4057, #3926 ) ) ;
#31993=AXIS2_PLACEMENT_3D ( 'NONE', #22855, #368, #15623 ) ;
#31997=ORIENTED_EDGE ( 'NONE', *, *, #6526, .T. ) ;
#31999=DIRECTION ( 'NONE',  ( -1.000000000000000000, 0.000000000000000000, 0.000000000000000000 ) ) ;
#32003=DIRECTION ( 'NONE',  ( 1.000000000000000000, 0.000000000000000000, 0.000000000000000000 ) ) ;
#32005=EDGE_LOOP ( 'NONE', ( #30048, #22959, #29377, #22854 ) ) ;
#32012=ORIENTED_EDGE ( 'NONE', *, *, #19205, .T. ) ;
#32017=ORIENTED_EDGE ( 'NONE', *, *, #2115, .F. ) ;
#32025=AXIS2_PLACEMENT_3D ( 'NONE', #11869, #24007, #21536 ) ;
#32031=CIRCLE ( 'NONE', #16273, 0.1249999999999931721 ) ;
#32035=DIRECTION ( 'NONE',  ( 1.000000000000000000, 0.000000000000000000, 0.000000000000000000 ) ) ;
#32037=ORIENTED_EDGE ( 'NONE', *, *, #2155, .T. ) ;
#32038=AXIS2_PLACEMENT_3D ( 'NONE', #22235, #27164, #22394 ) ;
#32041=VECTOR ( 'NONE', #30762, 1000.000000000000000 ) ;
#32044=VECTOR ( 'NONE', #25237, 1000.000000000000000 ) ;
#32049=DIRECTION ( 'NONE',  ( -1.101824276508909887E-16, 1.000000000000000000, -0.000000000000000000 ) ) ;
#32069=DIRECTION ( 'NONE',  ( -1.101824276508909887E-16, 1.000000000000000000, -0.000000000000000000 ) ) ;
#32070=CIRCLE ( 'NONE', #28389, 12.27641737965281798 ) ;
#32080=EDGE_CURVE ( 'NONE', #31343, #24565, #20172, .T. ) ;
#32083=EDGE_CURVE ( 'NONE', #28828, #32275, #13876, .T. ) ;
#32085=CARTESIAN_POINT ( 'NONE',  ( 33.72499318558949710, 30.34184655352422411, 47.04930799450051637 ) ) ;
#32087=CARTESIAN_POINT ( 'NONE',  ( 21.09992658989239089, 24.59164230456639544, 47.04930799450051637 ) ) ;
#32092=ORIENTED_EDGE ( 'NONE', *, *, #16744, .T. ) ;
#32100=DIRECTION ( 'NONE',  ( -1.101824276508909887E-16, 1.000000000000000000, -0.000000000000000000 ) ) ;
#32103=VERTEX_POINT ( 'NONE', #13412 ) ;
#32107=DIRECTION ( 'NONE',  ( -1.000000000000000000, 0.000000000000000000, 0.000000000000000000 ) ) ;
#32108=DIRECTION ( 'NONE',  ( -1.101824276508909887E-16, 1.000000000000000000, -0.000000000000000000 ) ) ;
#32109=AXIS2_PLACEMENT_3D ( 'NONE', #15260, #2462, #22803 ) ;
#32111=PRODUCT_DEFINITION_SHAPE ( 'NONE', 'NONE',  #9511 ) ;
#32113=EDGE_CURVE ( 'NONE', #8460, #3912, #1849, .T. ) ;
#32115=ORIENTED_EDGE ( 'NONE', *, *, #31538, .T. ) ;
#32118=DIRECTION ( 'NONE',  ( -1.101824276508909887E-16, 1.000000000000000000, -0.000000000000000000 ) ) ;
#32119=EDGE_CURVE ( 'NONE', #5692, #13543, #11581, .T. ) ;
#32120=ORIENTED_EDGE ( 'NONE', *, *, #7152, .F. ) ;
#32122=DIRECTION ( 'NONE',  ( -1.224646799147353207E-16, -1.349345573449484691E-32, 1.000000000000000000 ) ) ;
#32126=AXIS2_PLACEMENT_3D ( 'NONE', #10820, #23600, #20812 ) ;
#32127=FACE_OUTER_BOUND ( 'NONE', #20890, .T. ) ;
#32129=DIRECTION ( 'NONE',  ( -1.000000000000000000, 0.000000000000000000, 0.000000000000000000 ) ) ;
#32137=LINE ( 'NONE', #7181, #23657 ) ;
#32145=EDGE_LOOP ( 'NONE', ( #5994, #23386, #5091, #7553 ) ) ;
#32154=VERTEX_POINT ( 'NONE', #26348 ) ;
#32157=TOROIDAL_SURFACE ( 'NONE', #24820, 12.40141737965286595, 0.1249999999999979183 ) ;
#32165=DIRECTION ( 'NONE',  ( -1.101824276508909887E-16, 1.000000000000000000, -0.000000000000000000 ) ) ;
#32166=DIRECTION ( 'NONE',  ( -1.000000000000000000, 0.000000000000000000, 0.000000000000000000 ) ) ;
#32173=CARTESIAN_POINT ( 'NONE',  ( 33.37634396954523197, 28.09164230456639544, 47.04930799450051637 ) ) ;
#32176=EDGE_CURVE ( 'NONE', #24311, #25250, #20196, .T. ) ;
#32178=EDGE_CURVE ( 'NONE', #13562, #10069, #3940, .T. ) ;
#32186=VECTOR ( 'NONE', #1896, 1000.000000000000000 ) ;
#32193=CARTESIAN_POINT ( 'NONE',  ( 8.474859994195282908, 38.56284415653841791, 47.04930799450051637 ) ) ;
#32197=ORIENTED_EDGE ( 'NONE', *, *, #17217, .T. ) ;
#32203=VERTEX_POINT ( 'NONE', #29921 ) ;
#32204=DIRECTION ( 'NONE',  ( 1.000000000000000000, 0.000000000000000000, 0.000000000000000000 ) ) ;
#32207=EDGE_CURVE ( 'NONE', #28202, #19596, #24658, .T. ) ;
#32209=FACE_OUTER_BOUND ( 'NONE', #8804, .T. ) ;
#32212=FACE_OUTER_BOUND ( 'NONE', #21126, .T. ) ;
#32214=ADVANCED_FACE ( 'NONE', ( #7264 ), #22187, .F. ) ;
#32215=ADVANCED_FACE ( 'NONE', ( #4632 ), #9710, .T. ) ;
#32217=DIRECTION ( 'NONE',  ( -1.000000000000000000, 0.000000000000000000, 0.000000000000000000 ) ) ;
#32221=VERTEX_POINT ( 'NONE', #28817 ) ;
#32228=CARTESIAN_POINT ( 'NONE',  ( 21.09992658989239089, 23.84164230456639544, 47.04930799450051637 ) ) ;
#32237=AXIS2_PLACEMENT_3D ( 'NONE', #16018, #8313, #30488 ) ;
#32243=ORIENTED_EDGE ( 'NONE', *, *, #21401, .T. ) ;
#32244=DIRECTION ( 'NONE',  ( -1.000000000000000000, -1.101824276508909887E-16, 0.000000000000000000 ) ) ;
#32247=DIRECTION ( 'NONE',  ( -1.101824276508909887E-16, 1.000000000000000000, -0.000000000000000000 ) ) ;
#32248=DIRECTION ( 'NONE',  ( -1.101824276508909887E-16, 1.000000000000000000, -0.000000000000000000 ) ) ;
#32249=CIRCLE ( 'NONE', #10235, 12.36707279061065279 ) ;
#32250=CIRCLE ( 'NONE', #12884, 12.62506659569710266 ) ;
#32253=DIRECTION ( 'NONE',  ( -1.224646799147353207E-16, -1.349345573449484691E-32, 1.000000000000000000 ) ) ;
#32255=AXIS2_PLACEMENT_3D ( 'NONE', #6396, #3936, #27060 ) ;
#32258=CARTESIAN_POINT ( 'NONE',  ( 8.732853799281734553, 38.56284415653841791, 47.04930799450051637 ) ) ;
#32270=ORIENTED_EDGE ( 'NONE', *, *, #4625, .T. ) ;
#32275=VERTEX_POINT ( 'NONE', #29960 ) ;
#32282=AXIS2_PLACEMENT_3D ( 'NONE', #23150, #667, #10700 ) ;
#32291=EDGE_CURVE ( 'NONE', #6807, #30857, #16514, .T. ) ;
#32296=TOROIDAL_SURFACE ( 'NONE', #9230, 12.40141737965280733, 0.1250000000000013878 ) ;
#32297=DIRECTION ( 'NONE',  ( -1.000000000000000000, -1.101824276508909887E-16, 0.000000000000000000 ) ) ;
#32303=DIRECTION ( 'NONE',  ( -1.101824276508909887E-16, 1.000000000000000000, -0.000000000000000000 ) ) ;
#32309=FACE_OUTER_BOUND ( 'NONE', #26682, .T. ) ;
#32317=CARTESIAN_POINT ( 'NONE',  ( 33.71785032049133690, 28.96664230456639899, 47.04930799450051637 ) ) ;
#32323=EDGE_CURVE ( 'NONE', #9250, #31904, #26991, .T. ) ;
#32325=CARTESIAN_POINT ( 'NONE',  ( 8.732853799281725671, 25.97145308207318593, 47.04930799450051637 ) ) ;
#32326=DIRECTION ( 'NONE',  ( -1.000000000000000000, 0.000000000000000000, 0.000000000000000000 ) ) ;
#32328=ORIENTED_EDGE ( 'NONE', *, *, #12798, .T. ) ;
#32336=ORIENTED_EDGE ( 'NONE', *, *, #17114, .F. ) ;
#32337=DIRECTION ( 'NONE',  ( -1.101824276508909887E-16, 1.000000000000000000, -0.000000000000000000 ) ) ;
#32339=DIRECTION ( 'NONE',  ( -1.101824276508909887E-16, 1.000000000000000000, -0.000000000000000000 ) ) ;
#32343=ORIENTED_EDGE ( 'NONE', *, *, #9964, .F. ) ;
#32344=VERTEX_POINT ( 'NONE', #9274 ) ;
#32345=DIRECTION ( 'NONE',  ( -1.101824276508909887E-16, 1.000000000000000000, -0.000000000000000000 ) ) ;
#32349=ORIENTED_EDGE ( 'NONE', *, *, #28398, .F. ) ;
#32362=AXIS2_PLACEMENT_3D ( 'NONE', #16099, #31056, #30578 ) ;
#32364=FACE_OUTER_BOUND ( 'NONE', #12331, .T. ) ;
#32365=ORIENTED_EDGE ( 'NONE', *, *, #27085, .T. ) ;
#32367=FACE_OUTER_BOUND ( 'NONE', #13618, .T. ) ;
#32378=ORIENTED_EDGE ( 'NONE', *, *, #4828, .F. ) ;
#32381=DIRECTION ( 'NONE',  ( -1.224646799147353207E-16, -1.349345573449484691E-32, 1.000000000000000000 ) ) ;
#32384=DIRECTION ( 'NONE',  ( -1.101824276508909887E-16, 1.000000000000000000, -0.000000000000000000 ) ) ;
#32393=AXIS2_PLACEMENT_3D ( 'NONE', #7028, #31978, #6873 ) ;
#32401=ADVANCED_FACE ( 'NONE', ( #25189 ), #7637, .T. ) ;
#32403=EDGE_CURVE ( 'NONE', #10702, #3113, #31730, .T. ) ;
#32406=ORIENTED_EDGE ( 'NONE', *, *, #22751, .T. ) ;
#32408=CARTESIAN_POINT ( 'NONE',  ( 8.732853799281734553, 38.56284415653841791, 47.04930799450051637 ) ) ;
#32409=AXIS2_PLACEMENT_3D ( 'NONE', #23826, #25810, #6271 ) ;
#32415=FACE_OUTER_BOUND ( 'NONE', #6707, .T. ) ;
#32417=CARTESIAN_POINT ( 'NONE',  ( 8.732853799281734553, 29.97145308207317527, 47.04930799450051637 ) ) ;
#32419=ORIENTED_EDGE ( 'NONE', *, *, #6149, .T. ) ;
#32422=DIRECTION ( 'NONE',  ( -1.000000000000000000, 0.000000000000000000, 0.000000000000000000 ) ) ;
#32428=ORIENTED_EDGE ( 'NONE', *, *, #25793, .T. ) ;
#32429=DIRECTION ( 'NONE',  ( -1.000000000000000000, -1.101824276508909887E-16, 0.000000000000000000 ) ) ;
#32434=ORIENTED_EDGE ( 'NONE', *, *, #19134, .T. ) ;
#32437=CIRCLE ( 'NONE', #8826, 12.62506659569710266 ) ;
#32438=ORIENTED_EDGE ( 'NONE', *, *, #4106, .F. ) ;
#32443=CIRCLE ( 'NONE', #26654, 12.27641737965287128 ) ;
#32447=ORIENTED_EDGE ( 'NONE', *, *, #9790, .F. ) ;
#32455=VERTEX_POINT ( 'NONE', #22722 ) ;
#32456=DIRECTION ( 'NONE',  ( -1.000000000000000000, 0.000000000000000000, 0.000000000000000000 ) ) ;
#32457=CIRCLE ( 'NONE', #11474, 12.62506659569710266 ) ;
#32458=ORIENTED_EDGE ( 'NONE', *, *, #2984, .F. ) ;
#32462=DIRECTION ( 'NONE',  ( 0.000000000000000000, -0.000000000000000000, -1.000000000000000000 ) ) ;
#32464=CARTESIAN_POINT ( 'NONE',  ( 21.09992658989239089, 26.84143805560860940, 47.04930799450051637 ) ) ;
#32467=DIRECTION ( 'NONE',  ( -1.101824276508909887E-16, 1.000000000000000000, -0.000000000000000000 ) ) ;
#32472=ORIENTED_EDGE ( 'NONE', *, *, #20670, .T. ) ;
#32480=EDGE_CURVE ( 'NONE', #6910, #25250, #3170, .T. ) ;
#32486=AXIS2_PLACEMENT_3D ( 'NONE', #13859, #31743, #26488 ) ;
#32494=VECTOR ( 'NONE', #19078, 1000.000000000000000 ) ;
#32516=COLOUR_RGB('Light Blue',0.38,0.62,0.78);
#32517=FILL_AREA_STYLE_COLOUR('',#32516);
#32518=FILL_AREA_STYLE('',(#32517));
#32519=SURFACE_STYLE_FILL_AREA(#32518);
#32520=SURFACE_SIDE_STYLE('',(#32519));
#32521=SURFACE_STYLE_USAGE(.BOTH.,#32520);
#32522=PRESENTATION_STYLE_ASSIGNMENT((#32521));
ENDSEC;
END-ISO-10303-21;
